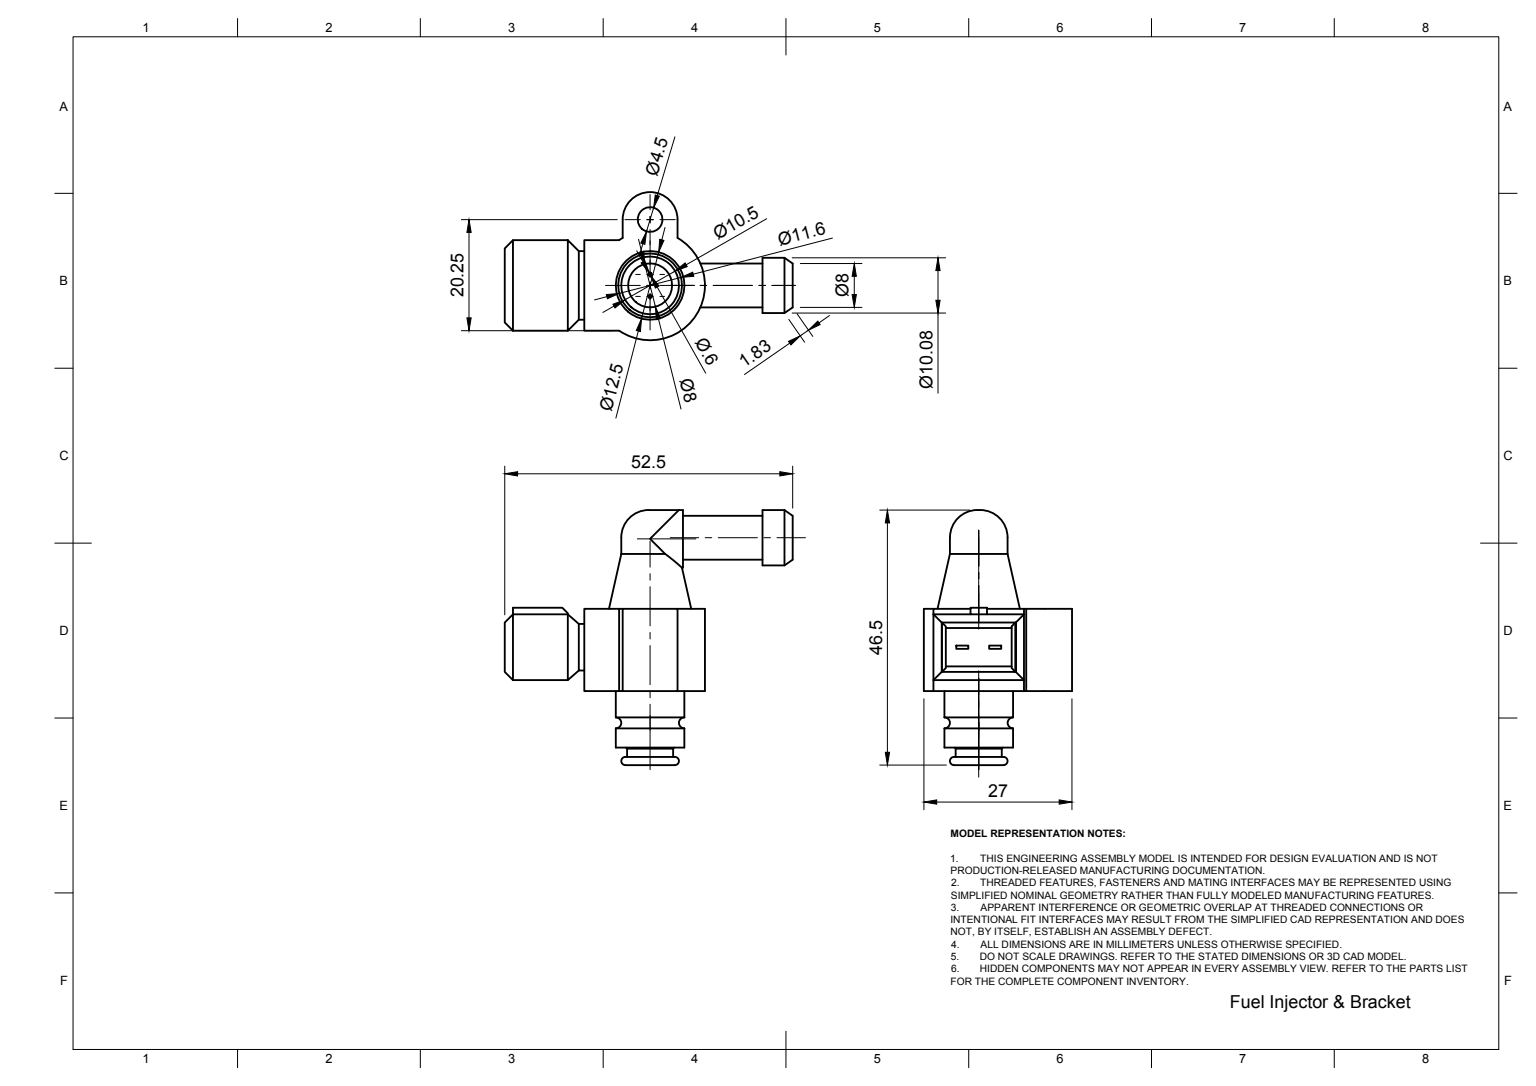
ISO-10303-21;
HEADER;
/* Generated by software containing ST-Developer
 * from STEP Tools, Inc. (www.steptools.com) 
 */

FILE_DESCRIPTION(
/* description */ ('STEP AP214'),
/* implementation_level */ '2;1');

FILE_NAME(
/* name */ 'Fuel Injector & Bracket.step',
/* time_stamp */ '2026-10-07T12:18:07-07:00',
/* author */ (''),
/* organization */ (''),
/* preprocessor_version */ 'ST-DEVELOPER v20.2',
/* originating_system */ 'Autodesk Translation Framework v15.15.0.0',
/* authorisation */ '');

FILE_SCHEMA (('AUTOMOTIVE_DESIGN { 1 0 10303 214 3 1 1 }'));
ENDSEC;

DATA;
#10=MECHANICAL_DESIGN_GEOMETRIC_PRESENTATION_REPRESENTATION('',(#122),#62974);
#98=SHAPE_REPRESENTATION_RELATIONSHIP('SRR','None',#63021,#110);
#110=ADVANCED_BREP_SHAPE_REPRESENTATION('',(#134),#62962);
#122=STYLED_ITEM('',(#63090),#134);
#134=MANIFOLD_SOLID_BREP('Body1',#15192);
#146=(
BOUNDED_SURFACE()
B_SPLINE_SURFACE(2,2,((#27768,#27769,#27770,#27771,#27772,#27773,#27774),
(#27775,#27776,#27777,#27778,#27779,#27780,#27781),(#27782,#27783,#27784,
#27785,#27786,#27787,#27788)),.UNSPECIFIED.,.F.,.F.,.F.)
B_SPLINE_SURFACE_WITH_KNOTS((3,3),(3,2,2,3),(-1.57079632681342,3.50763862399952E-12),
(-1.6184333897888,-0.539477796596266,0.539477796596266,1.6184333897888),
 .UNSPECIFIED.)
GEOMETRIC_REPRESENTATION_ITEM()
RATIONAL_B_SPLINE_SURFACE(((1.,0.857977047969415,1.,0.857977047969415,1.,
0.857977047969415,1.),(0.707106781178761,0.606681388714908,0.707106781178761,
0.606681388714908,0.707106781178761,0.606681388714908,0.707106781178761),
(1.,0.857977047969415,1.,0.857977047969415,1.,0.857977047969415,1.)))
REPRESENTATION_ITEM('')
SURFACE()
);
#192=B_SPLINE_SURFACE_WITH_KNOTS('',3,3,((#21716,#21717,#21718,#21719,#21720,
#21721,#21722,#21723,#21724,#21725,#21726,#21727,#21728,#21729,#21730,#21731,
#21732,#21733,#21734,#21735,#21736,#21737,#21738,#21739,#21740,#21741,#21742,
#21743,#21744,#21745,#21746,#21747,#21748,#21749,#21750,#21751,#21752,#21753,
#21754,#21755,#21756,#21757,#21758,#21759,#21760,#21761,#21762,#21763,#21764),
(#21765,#21766,#21767,#21768,#21769,#21770,#21771,#21772,#21773,#21774,
#21775,#21776,#21777,#21778,#21779,#21780,#21781,#21782,#21783,#21784,#21785,
#21786,#21787,#21788,#21789,#21790,#21791,#21792,#21793,#21794,#21795,#21796,
#21797,#21798,#21799,#21800,#21801,#21802,#21803,#21804,#21805,#21806,#21807,
#21808,#21809,#21810,#21811,#21812,#21813),(#21814,#21815,#21816,#21817,
#21818,#21819,#21820,#21821,#21822,#21823,#21824,#21825,#21826,#21827,#21828,
#21829,#21830,#21831,#21832,#21833,#21834,#21835,#21836,#21837,#21838,#21839,
#21840,#21841,#21842,#21843,#21844,#21845,#21846,#21847,#21848,#21849,#21850,
#21851,#21852,#21853,#21854,#21855,#21856,#21857,#21858,#21859,#21860,#21861,
#21862),(#21863,#21864,#21865,#21866,#21867,#21868,#21869,#21870,#21871,
#21872,#21873,#21874,#21875,#21876,#21877,#21878,#21879,#21880,#21881,#21882,
#21883,#21884,#21885,#21886,#21887,#21888,#21889,#21890,#21891,#21892,#21893,
#21894,#21895,#21896,#21897,#21898,#21899,#21900,#21901,#21902,#21903,#21904,
#21905,#21906,#21907,#21908,#21909,#21910,#21911),(#21912,#21913,#21914,
#21915,#21916,#21917,#21918,#21919,#21920,#21921,#21922,#21923,#21924,#21925,
#21926,#21927,#21928,#21929,#21930,#21931,#21932,#21933,#21934,#21935,#21936,
#21937,#21938,#21939,#21940,#21941,#21942,#21943,#21944,#21945,#21946,#21947,
#21948,#21949,#21950,#21951,#21952,#21953,#21954,#21955,#21956,#21957,#21958,
#21959,#21960),(#21961,#21962,#21963,#21964,#21965,#21966,#21967,#21968,
#21969,#21970,#21971,#21972,#21973,#21974,#21975,#21976,#21977,#21978,#21979,
#21980,#21981,#21982,#21983,#21984,#21985,#21986,#21987,#21988,#21989,#21990,
#21991,#21992,#21993,#21994,#21995,#21996,#21997,#21998,#21999,#22000,#22001,
#22002,#22003,#22004,#22005,#22006,#22007,#22008,#22009),(#22010,#22011,
#22012,#22013,#22014,#22015,#22016,#22017,#22018,#22019,#22020,#22021,#22022,
#22023,#22024,#22025,#22026,#22027,#22028,#22029,#22030,#22031,#22032,#22033,
#22034,#22035,#22036,#22037,#22038,#22039,#22040,#22041,#22042,#22043,#22044,
#22045,#22046,#22047,#22048,#22049,#22050,#22051,#22052,#22053,#22054,#22055,
#22056,#22057,#22058),(#22059,#22060,#22061,#22062,#22063,#22064,#22065,
#22066,#22067,#22068,#22069,#22070,#22071,#22072,#22073,#22074,#22075,#22076,
#22077,#22078,#22079,#22080,#22081,#22082,#22083,#22084,#22085,#22086,#22087,
#22088,#22089,#22090,#22091,#22092,#22093,#22094,#22095,#22096,#22097,#22098,
#22099,#22100,#22101,#22102,#22103,#22104,#22105,#22106,#22107),(#22108,
#22109,#22110,#22111,#22112,#22113,#22114,#22115,#22116,#22117,#22118,#22119,
#22120,#22121,#22122,#22123,#22124,#22125,#22126,#22127,#22128,#22129,#22130,
#22131,#22132,#22133,#22134,#22135,#22136,#22137,#22138,#22139,#22140,#22141,
#22142,#22143,#22144,#22145,#22146,#22147,#22148,#22149,#22150,#22151,#22152,
#22153,#22154,#22155,#22156),(#22157,#22158,#22159,#22160,#22161,#22162,
#22163,#22164,#22165,#22166,#22167,#22168,#22169,#22170,#22171,#22172,#22173,
#22174,#22175,#22176,#22177,#22178,#22179,#22180,#22181,#22182,#22183,#22184,
#22185,#22186,#22187,#22188,#22189,#22190,#22191,#22192,#22193,#22194,#22195,
#22196,#22197,#22198,#22199,#22200,#22201,#22202,#22203,#22204,#22205),
(#22206,#22207,#22208,#22209,#22210,#22211,#22212,#22213,#22214,#22215,
#22216,#22217,#22218,#22219,#22220,#22221,#22222,#22223,#22224,#22225,#22226,
#22227,#22228,#22229,#22230,#22231,#22232,#22233,#22234,#22235,#22236,#22237,
#22238,#22239,#22240,#22241,#22242,#22243,#22244,#22245,#22246,#22247,#22248,
#22249,#22250,#22251,#22252,#22253,#22254),(#22255,#22256,#22257,#22258,
#22259,#22260,#22261,#22262,#22263,#22264,#22265,#22266,#22267,#22268,#22269,
#22270,#22271,#22272,#22273,#22274,#22275,#22276,#22277,#22278,#22279,#22280,
#22281,#22282,#22283,#22284,#22285,#22286,#22287,#22288,#22289,#22290,#22291,
#22292,#22293,#22294,#22295,#22296,#22297,#22298,#22299,#22300,#22301,#22302,
#22303),(#22304,#22305,#22306,#22307,#22308,#22309,#22310,#22311,#22312,
#22313,#22314,#22315,#22316,#22317,#22318,#22319,#22320,#22321,#22322,#22323,
#22324,#22325,#22326,#22327,#22328,#22329,#22330,#22331,#22332,#22333,#22334,
#22335,#22336,#22337,#22338,#22339,#22340,#22341,#22342,#22343,#22344,#22345,
#22346,#22347,#22348,#22349,#22350,#22351,#22352),(#22353,#22354,#22355,
#22356,#22357,#22358,#22359,#22360,#22361,#22362,#22363,#22364,#22365,#22366,
#22367,#22368,#22369,#22370,#22371,#22372,#22373,#22374,#22375,#22376,#22377,
#22378,#22379,#22380,#22381,#22382,#22383,#22384,#22385,#22386,#22387,#22388,
#22389,#22390,#22391,#22392,#22393,#22394,#22395,#22396,#22397,#22398,#22399,
#22400,#22401),(#22402,#22403,#22404,#22405,#22406,#22407,#22408,#22409,
#22410,#22411,#22412,#22413,#22414,#22415,#22416,#22417,#22418,#22419,#22420,
#22421,#22422,#22423,#22424,#22425,#22426,#22427,#22428,#22429,#22430,#22431,
#22432,#22433,#22434,#22435,#22436,#22437,#22438,#22439,#22440,#22441,#22442,
#22443,#22444,#22445,#22446,#22447,#22448,#22449,#22450),(#22451,#22452,
#22453,#22454,#22455,#22456,#22457,#22458,#22459,#22460,#22461,#22462,#22463,
#22464,#22465,#22466,#22467,#22468,#22469,#22470,#22471,#22472,#22473,#22474,
#22475,#22476,#22477,#22478,#22479,#22480,#22481,#22482,#22483,#22484,#22485,
#22486,#22487,#22488,#22489,#22490,#22491,#22492,#22493,#22494,#22495,#22496,
#22497,#22498,#22499),(#22500,#22501,#22502,#22503,#22504,#22505,#22506,
#22507,#22508,#22509,#22510,#22511,#22512,#22513,#22514,#22515,#22516,#22517,
#22518,#22519,#22520,#22521,#22522,#22523,#22524,#22525,#22526,#22527,#22528,
#22529,#22530,#22531,#22532,#22533,#22534,#22535,#22536,#22537,#22538,#22539,
#22540,#22541,#22542,#22543,#22544,#22545,#22546,#22547,#22548),(#22549,
#22550,#22551,#22552,#22553,#22554,#22555,#22556,#22557,#22558,#22559,#22560,
#22561,#22562,#22563,#22564,#22565,#22566,#22567,#22568,#22569,#22570,#22571,
#22572,#22573,#22574,#22575,#22576,#22577,#22578,#22579,#22580,#22581,#22582,
#22583,#22584,#22585,#22586,#22587,#22588,#22589,#22590,#22591,#22592,#22593,
#22594,#22595,#22596,#22597),(#22598,#22599,#22600,#22601,#22602,#22603,
#22604,#22605,#22606,#22607,#22608,#22609,#22610,#22611,#22612,#22613,#22614,
#22615,#22616,#22617,#22618,#22619,#22620,#22621,#22622,#22623,#22624,#22625,
#22626,#22627,#22628,#22629,#22630,#22631,#22632,#22633,#22634,#22635,#22636,
#22637,#22638,#22639,#22640,#22641,#22642,#22643,#22644,#22645,#22646),
(#22647,#22648,#22649,#22650,#22651,#22652,#22653,#22654,#22655,#22656,
#22657,#22658,#22659,#22660,#22661,#22662,#22663,#22664,#22665,#22666,#22667,
#22668,#22669,#22670,#22671,#22672,#22673,#22674,#22675,#22676,#22677,#22678,
#22679,#22680,#22681,#22682,#22683,#22684,#22685,#22686,#22687,#22688,#22689,
#22690,#22691,#22692,#22693,#22694,#22695),(#22696,#22697,#22698,#22699,
#22700,#22701,#22702,#22703,#22704,#22705,#22706,#22707,#22708,#22709,#22710,
#22711,#22712,#22713,#22714,#22715,#22716,#22717,#22718,#22719,#22720,#22721,
#22722,#22723,#22724,#22725,#22726,#22727,#22728,#22729,#22730,#22731,#22732,
#22733,#22734,#22735,#22736,#22737,#22738,#22739,#22740,#22741,#22742,#22743,
#22744),(#22745,#22746,#22747,#22748,#22749,#22750,#22751,#22752,#22753,
#22754,#22755,#22756,#22757,#22758,#22759,#22760,#22761,#22762,#22763,#22764,
#22765,#22766,#22767,#22768,#22769,#22770,#22771,#22772,#22773,#22774,#22775,
#22776,#22777,#22778,#22779,#22780,#22781,#22782,#22783,#22784,#22785,#22786,
#22787,#22788,#22789,#22790,#22791,#22792,#22793),(#22794,#22795,#22796,
#22797,#22798,#22799,#22800,#22801,#22802,#22803,#22804,#22805,#22806,#22807,
#22808,#22809,#22810,#22811,#22812,#22813,#22814,#22815,#22816,#22817,#22818,
#22819,#22820,#22821,#22822,#22823,#22824,#22825,#22826,#22827,#22828,#22829,
#22830,#22831,#22832,#22833,#22834,#22835,#22836,#22837,#22838,#22839,#22840,
#22841,#22842),(#22843,#22844,#22845,#22846,#22847,#22848,#22849,#22850,
#22851,#22852,#22853,#22854,#22855,#22856,#22857,#22858,#22859,#22860,#22861,
#22862,#22863,#22864,#22865,#22866,#22867,#22868,#22869,#22870,#22871,#22872,
#22873,#22874,#22875,#22876,#22877,#22878,#22879,#22880,#22881,#22882,#22883,
#22884,#22885,#22886,#22887,#22888,#22889,#22890,#22891),(#22892,#22893,
#22894,#22895,#22896,#22897,#22898,#22899,#22900,#22901,#22902,#22903,#22904,
#22905,#22906,#22907,#22908,#22909,#22910,#22911,#22912,#22913,#22914,#22915,
#22916,#22917,#22918,#22919,#22920,#22921,#22922,#22923,#22924,#22925,#22926,
#22927,#22928,#22929,#22930,#22931,#22932,#22933,#22934,#22935,#22936,#22937,
#22938,#22939,#22940),(#22941,#22942,#22943,#22944,#22945,#22946,#22947,
#22948,#22949,#22950,#22951,#22952,#22953,#22954,#22955,#22956,#22957,#22958,
#22959,#22960,#22961,#22962,#22963,#22964,#22965,#22966,#22967,#22968,#22969,
#22970,#22971,#22972,#22973,#22974,#22975,#22976,#22977,#22978,#22979,#22980,
#22981,#22982,#22983,#22984,#22985,#22986,#22987,#22988,#22989),(#22990,
#22991,#22992,#22993,#22994,#22995,#22996,#22997,#22998,#22999,#23000,#23001,
#23002,#23003,#23004,#23005,#23006,#23007,#23008,#23009,#23010,#23011,#23012,
#23013,#23014,#23015,#23016,#23017,#23018,#23019,#23020,#23021,#23022,#23023,
#23024,#23025,#23026,#23027,#23028,#23029,#23030,#23031,#23032,#23033,#23034,
#23035,#23036,#23037,#23038),(#23039,#23040,#23041,#23042,#23043,#23044,
#23045,#23046,#23047,#23048,#23049,#23050,#23051,#23052,#23053,#23054,#23055,
#23056,#23057,#23058,#23059,#23060,#23061,#23062,#23063,#23064,#23065,#23066,
#23067,#23068,#23069,#23070,#23071,#23072,#23073,#23074,#23075,#23076,#23077,
#23078,#23079,#23080,#23081,#23082,#23083,#23084,#23085,#23086,#23087),
(#23088,#23089,#23090,#23091,#23092,#23093,#23094,#23095,#23096,#23097,
#23098,#23099,#23100,#23101,#23102,#23103,#23104,#23105,#23106,#23107,#23108,
#23109,#23110,#23111,#23112,#23113,#23114,#23115,#23116,#23117,#23118,#23119,
#23120,#23121,#23122,#23123,#23124,#23125,#23126,#23127,#23128,#23129,#23130,
#23131,#23132,#23133,#23134,#23135,#23136),(#23137,#23138,#23139,#23140,
#23141,#23142,#23143,#23144,#23145,#23146,#23147,#23148,#23149,#23150,#23151,
#23152,#23153,#23154,#23155,#23156,#23157,#23158,#23159,#23160,#23161,#23162,
#23163,#23164,#23165,#23166,#23167,#23168,#23169,#23170,#23171,#23172,#23173,
#23174,#23175,#23176,#23177,#23178,#23179,#23180,#23181,#23182,#23183,#23184,
#23185),(#23186,#23187,#23188,#23189,#23190,#23191,#23192,#23193,#23194,
#23195,#23196,#23197,#23198,#23199,#23200,#23201,#23202,#23203,#23204,#23205,
#23206,#23207,#23208,#23209,#23210,#23211,#23212,#23213,#23214,#23215,#23216,
#23217,#23218,#23219,#23220,#23221,#23222,#23223,#23224,#23225,#23226,#23227,
#23228,#23229,#23230,#23231,#23232,#23233,#23234),(#23235,#23236,#23237,
#23238,#23239,#23240,#23241,#23242,#23243,#23244,#23245,#23246,#23247,#23248,
#23249,#23250,#23251,#23252,#23253,#23254,#23255,#23256,#23257,#23258,#23259,
#23260,#23261,#23262,#23263,#23264,#23265,#23266,#23267,#23268,#23269,#23270,
#23271,#23272,#23273,#23274,#23275,#23276,#23277,#23278,#23279,#23280,#23281,
#23282,#23283),(#23284,#23285,#23286,#23287,#23288,#23289,#23290,#23291,
#23292,#23293,#23294,#23295,#23296,#23297,#23298,#23299,#23300,#23301,#23302,
#23303,#23304,#23305,#23306,#23307,#23308,#23309,#23310,#23311,#23312,#23313,
#23314,#23315,#23316,#23317,#23318,#23319,#23320,#23321,#23322,#23323,#23324,
#23325,#23326,#23327,#23328,#23329,#23330,#23331,#23332),(#23333,#23334,
#23335,#23336,#23337,#23338,#23339,#23340,#23341,#23342,#23343,#23344,#23345,
#23346,#23347,#23348,#23349,#23350,#23351,#23352,#23353,#23354,#23355,#23356,
#23357,#23358,#23359,#23360,#23361,#23362,#23363,#23364,#23365,#23366,#23367,
#23368,#23369,#23370,#23371,#23372,#23373,#23374,#23375,#23376,#23377,#23378,
#23379,#23380,#23381),(#23382,#23383,#23384,#23385,#23386,#23387,#23388,
#23389,#23390,#23391,#23392,#23393,#23394,#23395,#23396,#23397,#23398,#23399,
#23400,#23401,#23402,#23403,#23404,#23405,#23406,#23407,#23408,#23409,#23410,
#23411,#23412,#23413,#23414,#23415,#23416,#23417,#23418,#23419,#23420,#23421,
#23422,#23423,#23424,#23425,#23426,#23427,#23428,#23429,#23430),(#23431,
#23432,#23433,#23434,#23435,#23436,#23437,#23438,#23439,#23440,#23441,#23442,
#23443,#23444,#23445,#23446,#23447,#23448,#23449,#23450,#23451,#23452,#23453,
#23454,#23455,#23456,#23457,#23458,#23459,#23460,#23461,#23462,#23463,#23464,
#23465,#23466,#23467,#23468,#23469,#23470,#23471,#23472,#23473,#23474,#23475,
#23476,#23477,#23478,#23479),(#23480,#23481,#23482,#23483,#23484,#23485,
#23486,#23487,#23488,#23489,#23490,#23491,#23492,#23493,#23494,#23495,#23496,
#23497,#23498,#23499,#23500,#23501,#23502,#23503,#23504,#23505,#23506,#23507,
#23508,#23509,#23510,#23511,#23512,#23513,#23514,#23515,#23516,#23517,#23518,
#23519,#23520,#23521,#23522,#23523,#23524,#23525,#23526,#23527,#23528),
(#23529,#23530,#23531,#23532,#23533,#23534,#23535,#23536,#23537,#23538,
#23539,#23540,#23541,#23542,#23543,#23544,#23545,#23546,#23547,#23548,#23549,
#23550,#23551,#23552,#23553,#23554,#23555,#23556,#23557,#23558,#23559,#23560,
#23561,#23562,#23563,#23564,#23565,#23566,#23567,#23568,#23569,#23570,#23571,
#23572,#23573,#23574,#23575,#23576,#23577),(#23578,#23579,#23580,#23581,
#23582,#23583,#23584,#23585,#23586,#23587,#23588,#23589,#23590,#23591,#23592,
#23593,#23594,#23595,#23596,#23597,#23598,#23599,#23600,#23601,#23602,#23603,
#23604,#23605,#23606,#23607,#23608,#23609,#23610,#23611,#23612,#23613,#23614,
#23615,#23616,#23617,#23618,#23619,#23620,#23621,#23622,#23623,#23624,#23625,
#23626),(#23627,#23628,#23629,#23630,#23631,#23632,#23633,#23634,#23635,
#23636,#23637,#23638,#23639,#23640,#23641,#23642,#23643,#23644,#23645,#23646,
#23647,#23648,#23649,#23650,#23651,#23652,#23653,#23654,#23655,#23656,#23657,
#23658,#23659,#23660,#23661,#23662,#23663,#23664,#23665,#23666,#23667,#23668,
#23669,#23670,#23671,#23672,#23673,#23674,#23675),(#23676,#23677,#23678,
#23679,#23680,#23681,#23682,#23683,#23684,#23685,#23686,#23687,#23688,#23689,
#23690,#23691,#23692,#23693,#23694,#23695,#23696,#23697,#23698,#23699,#23700,
#23701,#23702,#23703,#23704,#23705,#23706,#23707,#23708,#23709,#23710,#23711,
#23712,#23713,#23714,#23715,#23716,#23717,#23718,#23719,#23720,#23721,#23722,
#23723,#23724),(#23725,#23726,#23727,#23728,#23729,#23730,#23731,#23732,
#23733,#23734,#23735,#23736,#23737,#23738,#23739,#23740,#23741,#23742,#23743,
#23744,#23745,#23746,#23747,#23748,#23749,#23750,#23751,#23752,#23753,#23754,
#23755,#23756,#23757,#23758,#23759,#23760,#23761,#23762,#23763,#23764,#23765,
#23766,#23767,#23768,#23769,#23770,#23771,#23772,#23773),(#23774,#23775,
#23776,#23777,#23778,#23779,#23780,#23781,#23782,#23783,#23784,#23785,#23786,
#23787,#23788,#23789,#23790,#23791,#23792,#23793,#23794,#23795,#23796,#23797,
#23798,#23799,#23800,#23801,#23802,#23803,#23804,#23805,#23806,#23807,#23808,
#23809,#23810,#23811,#23812,#23813,#23814,#23815,#23816,#23817,#23818,#23819,
#23820,#23821,#23822),(#23823,#23824,#23825,#23826,#23827,#23828,#23829,
#23830,#23831,#23832,#23833,#23834,#23835,#23836,#23837,#23838,#23839,#23840,
#23841,#23842,#23843,#23844,#23845,#23846,#23847,#23848,#23849,#23850,#23851,
#23852,#23853,#23854,#23855,#23856,#23857,#23858,#23859,#23860,#23861,#23862,
#23863,#23864,#23865,#23866,#23867,#23868,#23869,#23870,#23871),(#23872,
#23873,#23874,#23875,#23876,#23877,#23878,#23879,#23880,#23881,#23882,#23883,
#23884,#23885,#23886,#23887,#23888,#23889,#23890,#23891,#23892,#23893,#23894,
#23895,#23896,#23897,#23898,#23899,#23900,#23901,#23902,#23903,#23904,#23905,
#23906,#23907,#23908,#23909,#23910,#23911,#23912,#23913,#23914,#23915,#23916,
#23917,#23918,#23919,#23920),(#23921,#23922,#23923,#23924,#23925,#23926,
#23927,#23928,#23929,#23930,#23931,#23932,#23933,#23934,#23935,#23936,#23937,
#23938,#23939,#23940,#23941,#23942,#23943,#23944,#23945,#23946,#23947,#23948,
#23949,#23950,#23951,#23952,#23953,#23954,#23955,#23956,#23957,#23958,#23959,
#23960,#23961,#23962,#23963,#23964,#23965,#23966,#23967,#23968,#23969),
(#23970,#23971,#23972,#23973,#23974,#23975,#23976,#23977,#23978,#23979,
#23980,#23981,#23982,#23983,#23984,#23985,#23986,#23987,#23988,#23989,#23990,
#23991,#23992,#23993,#23994,#23995,#23996,#23997,#23998,#23999,#24000,#24001,
#24002,#24003,#24004,#24005,#24006,#24007,#24008,#24009,#24010,#24011,#24012,
#24013,#24014,#24015,#24016,#24017,#24018),(#24019,#24020,#24021,#24022,
#24023,#24024,#24025,#24026,#24027,#24028,#24029,#24030,#24031,#24032,#24033,
#24034,#24035,#24036,#24037,#24038,#24039,#24040,#24041,#24042,#24043,#24044,
#24045,#24046,#24047,#24048,#24049,#24050,#24051,#24052,#24053,#24054,#24055,
#24056,#24057,#24058,#24059,#24060,#24061,#24062,#24063,#24064,#24065,#24066,
#24067),(#24068,#24069,#24070,#24071,#24072,#24073,#24074,#24075,#24076,
#24077,#24078,#24079,#24080,#24081,#24082,#24083,#24084,#24085,#24086,#24087,
#24088,#24089,#24090,#24091,#24092,#24093,#24094,#24095,#24096,#24097,#24098,
#24099,#24100,#24101,#24102,#24103,#24104,#24105,#24106,#24107,#24108,#24109,
#24110,#24111,#24112,#24113,#24114,#24115,#24116),(#24117,#24118,#24119,
#24120,#24121,#24122,#24123,#24124,#24125,#24126,#24127,#24128,#24129,#24130,
#24131,#24132,#24133,#24134,#24135,#24136,#24137,#24138,#24139,#24140,#24141,
#24142,#24143,#24144,#24145,#24146,#24147,#24148,#24149,#24150,#24151,#24152,
#24153,#24154,#24155,#24156,#24157,#24158,#24159,#24160,#24161,#24162,#24163,
#24164,#24165),(#24166,#24167,#24168,#24169,#24170,#24171,#24172,#24173,
#24174,#24175,#24176,#24177,#24178,#24179,#24180,#24181,#24182,#24183,#24184,
#24185,#24186,#24187,#24188,#24189,#24190,#24191,#24192,#24193,#24194,#24195,
#24196,#24197,#24198,#24199,#24200,#24201,#24202,#24203,#24204,#24205,#24206,
#24207,#24208,#24209,#24210,#24211,#24212,#24213,#24214),(#24215,#24216,
#24217,#24218,#24219,#24220,#24221,#24222,#24223,#24224,#24225,#24226,#24227,
#24228,#24229,#24230,#24231,#24232,#24233,#24234,#24235,#24236,#24237,#24238,
#24239,#24240,#24241,#24242,#24243,#24244,#24245,#24246,#24247,#24248,#24249,
#24250,#24251,#24252,#24253,#24254,#24255,#24256,#24257,#24258,#24259,#24260,
#24261,#24262,#24263),(#24264,#24265,#24266,#24267,#24268,#24269,#24270,
#24271,#24272,#24273,#24274,#24275,#24276,#24277,#24278,#24279,#24280,#24281,
#24282,#24283,#24284,#24285,#24286,#24287,#24288,#24289,#24290,#24291,#24292,
#24293,#24294,#24295,#24296,#24297,#24298,#24299,#24300,#24301,#24302,#24303,
#24304,#24305,#24306,#24307,#24308,#24309,#24310,#24311,#24312),(#24313,
#24314,#24315,#24316,#24317,#24318,#24319,#24320,#24321,#24322,#24323,#24324,
#24325,#24326,#24327,#24328,#24329,#24330,#24331,#24332,#24333,#24334,#24335,
#24336,#24337,#24338,#24339,#24340,#24341,#24342,#24343,#24344,#24345,#24346,
#24347,#24348,#24349,#24350,#24351,#24352,#24353,#24354,#24355,#24356,#24357,
#24358,#24359,#24360,#24361),(#24362,#24363,#24364,#24365,#24366,#24367,
#24368,#24369,#24370,#24371,#24372,#24373,#24374,#24375,#24376,#24377,#24378,
#24379,#24380,#24381,#24382,#24383,#24384,#24385,#24386,#24387,#24388,#24389,
#24390,#24391,#24392,#24393,#24394,#24395,#24396,#24397,#24398,#24399,#24400,
#24401,#24402,#24403,#24404,#24405,#24406,#24407,#24408,#24409,#24410),
(#24411,#24412,#24413,#24414,#24415,#24416,#24417,#24418,#24419,#24420,
#24421,#24422,#24423,#24424,#24425,#24426,#24427,#24428,#24429,#24430,#24431,
#24432,#24433,#24434,#24435,#24436,#24437,#24438,#24439,#24440,#24441,#24442,
#24443,#24444,#24445,#24446,#24447,#24448,#24449,#24450,#24451,#24452,#24453,
#24454,#24455,#24456,#24457,#24458,#24459),(#24460,#24461,#24462,#24463,
#24464,#24465,#24466,#24467,#24468,#24469,#24470,#24471,#24472,#24473,#24474,
#24475,#24476,#24477,#24478,#24479,#24480,#24481,#24482,#24483,#24484,#24485,
#24486,#24487,#24488,#24489,#24490,#24491,#24492,#24493,#24494,#24495,#24496,
#24497,#24498,#24499,#24500,#24501,#24502,#24503,#24504,#24505,#24506,#24507,
#24508),(#24509,#24510,#24511,#24512,#24513,#24514,#24515,#24516,#24517,
#24518,#24519,#24520,#24521,#24522,#24523,#24524,#24525,#24526,#24527,#24528,
#24529,#24530,#24531,#24532,#24533,#24534,#24535,#24536,#24537,#24538,#24539,
#24540,#24541,#24542,#24543,#24544,#24545,#24546,#24547,#24548,#24549,#24550,
#24551,#24552,#24553,#24554,#24555,#24556,#24557),(#24558,#24559,#24560,
#24561,#24562,#24563,#24564,#24565,#24566,#24567,#24568,#24569,#24570,#24571,
#24572,#24573,#24574,#24575,#24576,#24577,#24578,#24579,#24580,#24581,#24582,
#24583,#24584,#24585,#24586,#24587,#24588,#24589,#24590,#24591,#24592,#24593,
#24594,#24595,#24596,#24597,#24598,#24599,#24600,#24601,#24602,#24603,#24604,
#24605,#24606),(#24607,#24608,#24609,#24610,#24611,#24612,#24613,#24614,
#24615,#24616,#24617,#24618,#24619,#24620,#24621,#24622,#24623,#24624,#24625,
#24626,#24627,#24628,#24629,#24630,#24631,#24632,#24633,#24634,#24635,#24636,
#24637,#24638,#24639,#24640,#24641,#24642,#24643,#24644,#24645,#24646,#24647,
#24648,#24649,#24650,#24651,#24652,#24653,#24654,#24655),(#24656,#24657,
#24658,#24659,#24660,#24661,#24662,#24663,#24664,#24665,#24666,#24667,#24668,
#24669,#24670,#24671,#24672,#24673,#24674,#24675,#24676,#24677,#24678,#24679,
#24680,#24681,#24682,#24683,#24684,#24685,#24686,#24687,#24688,#24689,#24690,
#24691,#24692,#24693,#24694,#24695,#24696,#24697,#24698,#24699,#24700,#24701,
#24702,#24703,#24704),(#24705,#24706,#24707,#24708,#24709,#24710,#24711,
#24712,#24713,#24714,#24715,#24716,#24717,#24718,#24719,#24720,#24721,#24722,
#24723,#24724,#24725,#24726,#24727,#24728,#24729,#24730,#24731,#24732,#24733,
#24734,#24735,#24736,#24737,#24738,#24739,#24740,#24741,#24742,#24743,#24744,
#24745,#24746,#24747,#24748,#24749,#24750,#24751,#24752,#24753),(#24754,
#24755,#24756,#24757,#24758,#24759,#24760,#24761,#24762,#24763,#24764,#24765,
#24766,#24767,#24768,#24769,#24770,#24771,#24772,#24773,#24774,#24775,#24776,
#24777,#24778,#24779,#24780,#24781,#24782,#24783,#24784,#24785,#24786,#24787,
#24788,#24789,#24790,#24791,#24792,#24793,#24794,#24795,#24796,#24797,#24798,
#24799,#24800,#24801,#24802),(#24803,#24804,#24805,#24806,#24807,#24808,
#24809,#24810,#24811,#24812,#24813,#24814,#24815,#24816,#24817,#24818,#24819,
#24820,#24821,#24822,#24823,#24824,#24825,#24826,#24827,#24828,#24829,#24830,
#24831,#24832,#24833,#24834,#24835,#24836,#24837,#24838,#24839,#24840,#24841,
#24842,#24843,#24844,#24845,#24846,#24847,#24848,#24849,#24850,#24851),
(#24852,#24853,#24854,#24855,#24856,#24857,#24858,#24859,#24860,#24861,
#24862,#24863,#24864,#24865,#24866,#24867,#24868,#24869,#24870,#24871,#24872,
#24873,#24874,#24875,#24876,#24877,#24878,#24879,#24880,#24881,#24882,#24883,
#24884,#24885,#24886,#24887,#24888,#24889,#24890,#24891,#24892,#24893,#24894,
#24895,#24896,#24897,#24898,#24899,#24900),(#24901,#24902,#24903,#24904,
#24905,#24906,#24907,#24908,#24909,#24910,#24911,#24912,#24913,#24914,#24915,
#24916,#24917,#24918,#24919,#24920,#24921,#24922,#24923,#24924,#24925,#24926,
#24927,#24928,#24929,#24930,#24931,#24932,#24933,#24934,#24935,#24936,#24937,
#24938,#24939,#24940,#24941,#24942,#24943,#24944,#24945,#24946,#24947,#24948,
#24949),(#24950,#24951,#24952,#24953,#24954,#24955,#24956,#24957,#24958,
#24959,#24960,#24961,#24962,#24963,#24964,#24965,#24966,#24967,#24968,#24969,
#24970,#24971,#24972,#24973,#24974,#24975,#24976,#24977,#24978,#24979,#24980,
#24981,#24982,#24983,#24984,#24985,#24986,#24987,#24988,#24989,#24990,#24991,
#24992,#24993,#24994,#24995,#24996,#24997,#24998),(#24999,#25000,#25001,
#25002,#25003,#25004,#25005,#25006,#25007,#25008,#25009,#25010,#25011,#25012,
#25013,#25014,#25015,#25016,#25017,#25018,#25019,#25020,#25021,#25022,#25023,
#25024,#25025,#25026,#25027,#25028,#25029,#25030,#25031,#25032,#25033,#25034,
#25035,#25036,#25037,#25038,#25039,#25040,#25041,#25042,#25043,#25044,#25045,
#25046,#25047),(#25048,#25049,#25050,#25051,#25052,#25053,#25054,#25055,
#25056,#25057,#25058,#25059,#25060,#25061,#25062,#25063,#25064,#25065,#25066,
#25067,#25068,#25069,#25070,#25071,#25072,#25073,#25074,#25075,#25076,#25077,
#25078,#25079,#25080,#25081,#25082,#25083,#25084,#25085,#25086,#25087,#25088,
#25089,#25090,#25091,#25092,#25093,#25094,#25095,#25096),(#25097,#25098,
#25099,#25100,#25101,#25102,#25103,#25104,#25105,#25106,#25107,#25108,#25109,
#25110,#25111,#25112,#25113,#25114,#25115,#25116,#25117,#25118,#25119,#25120,
#25121,#25122,#25123,#25124,#25125,#25126,#25127,#25128,#25129,#25130,#25131,
#25132,#25133,#25134,#25135,#25136,#25137,#25138,#25139,#25140,#25141,#25142,
#25143,#25144,#25145),(#25146,#25147,#25148,#25149,#25150,#25151,#25152,
#25153,#25154,#25155,#25156,#25157,#25158,#25159,#25160,#25161,#25162,#25163,
#25164,#25165,#25166,#25167,#25168,#25169,#25170,#25171,#25172,#25173,#25174,
#25175,#25176,#25177,#25178,#25179,#25180,#25181,#25182,#25183,#25184,#25185,
#25186,#25187,#25188,#25189,#25190,#25191,#25192,#25193,#25194),(#25195,
#25196,#25197,#25198,#25199,#25200,#25201,#25202,#25203,#25204,#25205,#25206,
#25207,#25208,#25209,#25210,#25211,#25212,#25213,#25214,#25215,#25216,#25217,
#25218,#25219,#25220,#25221,#25222,#25223,#25224,#25225,#25226,#25227,#25228,
#25229,#25230,#25231,#25232,#25233,#25234,#25235,#25236,#25237,#25238,#25239,
#25240,#25241,#25242,#25243),(#25244,#25245,#25246,#25247,#25248,#25249,
#25250,#25251,#25252,#25253,#25254,#25255,#25256,#25257,#25258,#25259,#25260,
#25261,#25262,#25263,#25264,#25265,#25266,#25267,#25268,#25269,#25270,#25271,
#25272,#25273,#25274,#25275,#25276,#25277,#25278,#25279,#25280,#25281,#25282,
#25283,#25284,#25285,#25286,#25287,#25288,#25289,#25290,#25291,#25292),
(#25293,#25294,#25295,#25296,#25297,#25298,#25299,#25300,#25301,#25302,
#25303,#25304,#25305,#25306,#25307,#25308,#25309,#25310,#25311,#25312,#25313,
#25314,#25315,#25316,#25317,#25318,#25319,#25320,#25321,#25322,#25323,#25324,
#25325,#25326,#25327,#25328,#25329,#25330,#25331,#25332,#25333,#25334,#25335,
#25336,#25337,#25338,#25339,#25340,#25341),(#25342,#25343,#25344,#25345,
#25346,#25347,#25348,#25349,#25350,#25351,#25352,#25353,#25354,#25355,#25356,
#25357,#25358,#25359,#25360,#25361,#25362,#25363,#25364,#25365,#25366,#25367,
#25368,#25369,#25370,#25371,#25372,#25373,#25374,#25375,#25376,#25377,#25378,
#25379,#25380,#25381,#25382,#25383,#25384,#25385,#25386,#25387,#25388,#25389,
#25390),(#25391,#25392,#25393,#25394,#25395,#25396,#25397,#25398,#25399,
#25400,#25401,#25402,#25403,#25404,#25405,#25406,#25407,#25408,#25409,#25410,
#25411,#25412,#25413,#25414,#25415,#25416,#25417,#25418,#25419,#25420,#25421,
#25422,#25423,#25424,#25425,#25426,#25427,#25428,#25429,#25430,#25431,#25432,
#25433,#25434,#25435,#25436,#25437,#25438,#25439),(#25440,#25441,#25442,
#25443,#25444,#25445,#25446,#25447,#25448,#25449,#25450,#25451,#25452,#25453,
#25454,#25455,#25456,#25457,#25458,#25459,#25460,#25461,#25462,#25463,#25464,
#25465,#25466,#25467,#25468,#25469,#25470,#25471,#25472,#25473,#25474,#25475,
#25476,#25477,#25478,#25479,#25480,#25481,#25482,#25483,#25484,#25485,#25486,
#25487,#25488),(#25489,#25490,#25491,#25492,#25493,#25494,#25495,#25496,
#25497,#25498,#25499,#25500,#25501,#25502,#25503,#25504,#25505,#25506,#25507,
#25508,#25509,#25510,#25511,#25512,#25513,#25514,#25515,#25516,#25517,#25518,
#25519,#25520,#25521,#25522,#25523,#25524,#25525,#25526,#25527,#25528,#25529,
#25530,#25531,#25532,#25533,#25534,#25535,#25536,#25537),(#25538,#25539,
#25540,#25541,#25542,#25543,#25544,#25545,#25546,#25547,#25548,#25549,#25550,
#25551,#25552,#25553,#25554,#25555,#25556,#25557,#25558,#25559,#25560,#25561,
#25562,#25563,#25564,#25565,#25566,#25567,#25568,#25569,#25570,#25571,#25572,
#25573,#25574,#25575,#25576,#25577,#25578,#25579,#25580,#25581,#25582,#25583,
#25584,#25585,#25586),(#25587,#25588,#25589,#25590,#25591,#25592,#25593,
#25594,#25595,#25596,#25597,#25598,#25599,#25600,#25601,#25602,#25603,#25604,
#25605,#25606,#25607,#25608,#25609,#25610,#25611,#25612,#25613,#25614,#25615,
#25616,#25617,#25618,#25619,#25620,#25621,#25622,#25623,#25624,#25625,#25626,
#25627,#25628,#25629,#25630,#25631,#25632,#25633,#25634,#25635),(#25636,
#25637,#25638,#25639,#25640,#25641,#25642,#25643,#25644,#25645,#25646,#25647,
#25648,#25649,#25650,#25651,#25652,#25653,#25654,#25655,#25656,#25657,#25658,
#25659,#25660,#25661,#25662,#25663,#25664,#25665,#25666,#25667,#25668,#25669,
#25670,#25671,#25672,#25673,#25674,#25675,#25676,#25677,#25678,#25679,#25680,
#25681,#25682,#25683,#25684),(#25685,#25686,#25687,#25688,#25689,#25690,
#25691,#25692,#25693,#25694,#25695,#25696,#25697,#25698,#25699,#25700,#25701,
#25702,#25703,#25704,#25705,#25706,#25707,#25708,#25709,#25710,#25711,#25712,
#25713,#25714,#25715,#25716,#25717,#25718,#25719,#25720,#25721,#25722,#25723,
#25724,#25725,#25726,#25727,#25728,#25729,#25730,#25731,#25732,#25733),
(#25734,#25735,#25736,#25737,#25738,#25739,#25740,#25741,#25742,#25743,
#25744,#25745,#25746,#25747,#25748,#25749,#25750,#25751,#25752,#25753,#25754,
#25755,#25756,#25757,#25758,#25759,#25760,#25761,#25762,#25763,#25764,#25765,
#25766,#25767,#25768,#25769,#25770,#25771,#25772,#25773,#25774,#25775,#25776,
#25777,#25778,#25779,#25780,#25781,#25782),(#25783,#25784,#25785,#25786,
#25787,#25788,#25789,#25790,#25791,#25792,#25793,#25794,#25795,#25796,#25797,
#25798,#25799,#25800,#25801,#25802,#25803,#25804,#25805,#25806,#25807,#25808,
#25809,#25810,#25811,#25812,#25813,#25814,#25815,#25816,#25817,#25818,#25819,
#25820,#25821,#25822,#25823,#25824,#25825,#25826,#25827,#25828,#25829,#25830,
#25831),(#25832,#25833,#25834,#25835,#25836,#25837,#25838,#25839,#25840,
#25841,#25842,#25843,#25844,#25845,#25846,#25847,#25848,#25849,#25850,#25851,
#25852,#25853,#25854,#25855,#25856,#25857,#25858,#25859,#25860,#25861,#25862,
#25863,#25864,#25865,#25866,#25867,#25868,#25869,#25870,#25871,#25872,#25873,
#25874,#25875,#25876,#25877,#25878,#25879,#25880),(#25881,#25882,#25883,
#25884,#25885,#25886,#25887,#25888,#25889,#25890,#25891,#25892,#25893,#25894,
#25895,#25896,#25897,#25898,#25899,#25900,#25901,#25902,#25903,#25904,#25905,
#25906,#25907,#25908,#25909,#25910,#25911,#25912,#25913,#25914,#25915,#25916,
#25917,#25918,#25919,#25920,#25921,#25922,#25923,#25924,#25925,#25926,#25927,
#25928,#25929),(#25930,#25931,#25932,#25933,#25934,#25935,#25936,#25937,
#25938,#25939,#25940,#25941,#25942,#25943,#25944,#25945,#25946,#25947,#25948,
#25949,#25950,#25951,#25952,#25953,#25954,#25955,#25956,#25957,#25958,#25959,
#25960,#25961,#25962,#25963,#25964,#25965,#25966,#25967,#25968,#25969,#25970,
#25971,#25972,#25973,#25974,#25975,#25976,#25977,#25978),(#25979,#25980,
#25981,#25982,#25983,#25984,#25985,#25986,#25987,#25988,#25989,#25990,#25991,
#25992,#25993,#25994,#25995,#25996,#25997,#25998,#25999,#26000,#26001,#26002,
#26003,#26004,#26005,#26006,#26007,#26008,#26009,#26010,#26011,#26012,#26013,
#26014,#26015,#26016,#26017,#26018,#26019,#26020,#26021,#26022,#26023,#26024,
#26025,#26026,#26027),(#26028,#26029,#26030,#26031,#26032,#26033,#26034,
#26035,#26036,#26037,#26038,#26039,#26040,#26041,#26042,#26043,#26044,#26045,
#26046,#26047,#26048,#26049,#26050,#26051,#26052,#26053,#26054,#26055,#26056,
#26057,#26058,#26059,#26060,#26061,#26062,#26063,#26064,#26065,#26066,#26067,
#26068,#26069,#26070,#26071,#26072,#26073,#26074,#26075,#26076),(#26077,
#26078,#26079,#26080,#26081,#26082,#26083,#26084,#26085,#26086,#26087,#26088,
#26089,#26090,#26091,#26092,#26093,#26094,#26095,#26096,#26097,#26098,#26099,
#26100,#26101,#26102,#26103,#26104,#26105,#26106,#26107,#26108,#26109,#26110,
#26111,#26112,#26113,#26114,#26115,#26116,#26117,#26118,#26119,#26120,#26121,
#26122,#26123,#26124,#26125),(#26126,#26127,#26128,#26129,#26130,#26131,
#26132,#26133,#26134,#26135,#26136,#26137,#26138,#26139,#26140,#26141,#26142,
#26143,#26144,#26145,#26146,#26147,#26148,#26149,#26150,#26151,#26152,#26153,
#26154,#26155,#26156,#26157,#26158,#26159,#26160,#26161,#26162,#26163,#26164,
#26165,#26166,#26167,#26168,#26169,#26170,#26171,#26172,#26173,#26174),
(#26175,#26176,#26177,#26178,#26179,#26180,#26181,#26182,#26183,#26184,
#26185,#26186,#26187,#26188,#26189,#26190,#26191,#26192,#26193,#26194,#26195,
#26196,#26197,#26198,#26199,#26200,#26201,#26202,#26203,#26204,#26205,#26206,
#26207,#26208,#26209,#26210,#26211,#26212,#26213,#26214,#26215,#26216,#26217,
#26218,#26219,#26220,#26221,#26222,#26223),(#26224,#26225,#26226,#26227,
#26228,#26229,#26230,#26231,#26232,#26233,#26234,#26235,#26236,#26237,#26238,
#26239,#26240,#26241,#26242,#26243,#26244,#26245,#26246,#26247,#26248,#26249,
#26250,#26251,#26252,#26253,#26254,#26255,#26256,#26257,#26258,#26259,#26260,
#26261,#26262,#26263,#26264,#26265,#26266,#26267,#26268,#26269,#26270,#26271,
#26272),(#26273,#26274,#26275,#26276,#26277,#26278,#26279,#26280,#26281,
#26282,#26283,#26284,#26285,#26286,#26287,#26288,#26289,#26290,#26291,#26292,
#26293,#26294,#26295,#26296,#26297,#26298,#26299,#26300,#26301,#26302,#26303,
#26304,#26305,#26306,#26307,#26308,#26309,#26310,#26311,#26312,#26313,#26314,
#26315,#26316,#26317,#26318,#26319,#26320,#26321),(#26322,#26323,#26324,
#26325,#26326,#26327,#26328,#26329,#26330,#26331,#26332,#26333,#26334,#26335,
#26336,#26337,#26338,#26339,#26340,#26341,#26342,#26343,#26344,#26345,#26346,
#26347,#26348,#26349,#26350,#26351,#26352,#26353,#26354,#26355,#26356,#26357,
#26358,#26359,#26360,#26361,#26362,#26363,#26364,#26365,#26366,#26367,#26368,
#26369,#26370),(#26371,#26372,#26373,#26374,#26375,#26376,#26377,#26378,
#26379,#26380,#26381,#26382,#26383,#26384,#26385,#26386,#26387,#26388,#26389,
#26390,#26391,#26392,#26393,#26394,#26395,#26396,#26397,#26398,#26399,#26400,
#26401,#26402,#26403,#26404,#26405,#26406,#26407,#26408,#26409,#26410,#26411,
#26412,#26413,#26414,#26415,#26416,#26417,#26418,#26419),(#26420,#26421,
#26422,#26423,#26424,#26425,#26426,#26427,#26428,#26429,#26430,#26431,#26432,
#26433,#26434,#26435,#26436,#26437,#26438,#26439,#26440,#26441,#26442,#26443,
#26444,#26445,#26446,#26447,#26448,#26449,#26450,#26451,#26452,#26453,#26454,
#26455,#26456,#26457,#26458,#26459,#26460,#26461,#26462,#26463,#26464,#26465,
#26466,#26467,#26468),(#26469,#26470,#26471,#26472,#26473,#26474,#26475,
#26476,#26477,#26478,#26479,#26480,#26481,#26482,#26483,#26484,#26485,#26486,
#26487,#26488,#26489,#26490,#26491,#26492,#26493,#26494,#26495,#26496,#26497,
#26498,#26499,#26500,#26501,#26502,#26503,#26504,#26505,#26506,#26507,#26508,
#26509,#26510,#26511,#26512,#26513,#26514,#26515,#26516,#26517),(#26518,
#26519,#26520,#26521,#26522,#26523,#26524,#26525,#26526,#26527,#26528,#26529,
#26530,#26531,#26532,#26533,#26534,#26535,#26536,#26537,#26538,#26539,#26540,
#26541,#26542,#26543,#26544,#26545,#26546,#26547,#26548,#26549,#26550,#26551,
#26552,#26553,#26554,#26555,#26556,#26557,#26558,#26559,#26560,#26561,#26562,
#26563,#26564,#26565,#26566),(#26567,#26568,#26569,#26570,#26571,#26572,
#26573,#26574,#26575,#26576,#26577,#26578,#26579,#26580,#26581,#26582,#26583,
#26584,#26585,#26586,#26587,#26588,#26589,#26590,#26591,#26592,#26593,#26594,
#26595,#26596,#26597,#26598,#26599,#26600,#26601,#26602,#26603,#26604,#26605,
#26606,#26607,#26608,#26609,#26610,#26611,#26612,#26613,#26614,#26615),
(#26616,#26617,#26618,#26619,#26620,#26621,#26622,#26623,#26624,#26625,
#26626,#26627,#26628,#26629,#26630,#26631,#26632,#26633,#26634,#26635,#26636,
#26637,#26638,#26639,#26640,#26641,#26642,#26643,#26644,#26645,#26646,#26647,
#26648,#26649,#26650,#26651,#26652,#26653,#26654,#26655,#26656,#26657,#26658,
#26659,#26660,#26661,#26662,#26663,#26664),(#26665,#26666,#26667,#26668,
#26669,#26670,#26671,#26672,#26673,#26674,#26675,#26676,#26677,#26678,#26679,
#26680,#26681,#26682,#26683,#26684,#26685,#26686,#26687,#26688,#26689,#26690,
#26691,#26692,#26693,#26694,#26695,#26696,#26697,#26698,#26699,#26700,#26701,
#26702,#26703,#26704,#26705,#26706,#26707,#26708,#26709,#26710,#26711,#26712,
#26713),(#26714,#26715,#26716,#26717,#26718,#26719,#26720,#26721,#26722,
#26723,#26724,#26725,#26726,#26727,#26728,#26729,#26730,#26731,#26732,#26733,
#26734,#26735,#26736,#26737,#26738,#26739,#26740,#26741,#26742,#26743,#26744,
#26745,#26746,#26747,#26748,#26749,#26750,#26751,#26752,#26753,#26754,#26755,
#26756,#26757,#26758,#26759,#26760,#26761,#26762),(#26763,#26764,#26765,
#26766,#26767,#26768,#26769,#26770,#26771,#26772,#26773,#26774,#26775,#26776,
#26777,#26778,#26779,#26780,#26781,#26782,#26783,#26784,#26785,#26786,#26787,
#26788,#26789,#26790,#26791,#26792,#26793,#26794,#26795,#26796,#26797,#26798,
#26799,#26800,#26801,#26802,#26803,#26804,#26805,#26806,#26807,#26808,#26809,
#26810,#26811),(#26812,#26813,#26814,#26815,#26816,#26817,#26818,#26819,
#26820,#26821,#26822,#26823,#26824,#26825,#26826,#26827,#26828,#26829,#26830,
#26831,#26832,#26833,#26834,#26835,#26836,#26837,#26838,#26839,#26840,#26841,
#26842,#26843,#26844,#26845,#26846,#26847,#26848,#26849,#26850,#26851,#26852,
#26853,#26854,#26855,#26856,#26857,#26858,#26859,#26860),(#26861,#26862,
#26863,#26864,#26865,#26866,#26867,#26868,#26869,#26870,#26871,#26872,#26873,
#26874,#26875,#26876,#26877,#26878,#26879,#26880,#26881,#26882,#26883,#26884,
#26885,#26886,#26887,#26888,#26889,#26890,#26891,#26892,#26893,#26894,#26895,
#26896,#26897,#26898,#26899,#26900,#26901,#26902,#26903,#26904,#26905,#26906,
#26907,#26908,#26909),(#26910,#26911,#26912,#26913,#26914,#26915,#26916,
#26917,#26918,#26919,#26920,#26921,#26922,#26923,#26924,#26925,#26926,#26927,
#26928,#26929,#26930,#26931,#26932,#26933,#26934,#26935,#26936,#26937,#26938,
#26939,#26940,#26941,#26942,#26943,#26944,#26945,#26946,#26947,#26948,#26949,
#26950,#26951,#26952,#26953,#26954,#26955,#26956,#26957,#26958),(#26959,
#26960,#26961,#26962,#26963,#26964,#26965,#26966,#26967,#26968,#26969,#26970,
#26971,#26972,#26973,#26974,#26975,#26976,#26977,#26978,#26979,#26980,#26981,
#26982,#26983,#26984,#26985,#26986,#26987,#26988,#26989,#26990,#26991,#26992,
#26993,#26994,#26995,#26996,#26997,#26998,#26999,#27000,#27001,#27002,#27003,
#27004,#27005,#27006,#27007),(#27008,#27009,#27010,#27011,#27012,#27013,
#27014,#27015,#27016,#27017,#27018,#27019,#27020,#27021,#27022,#27023,#27024,
#27025,#27026,#27027,#27028,#27029,#27030,#27031,#27032,#27033,#27034,#27035,
#27036,#27037,#27038,#27039,#27040,#27041,#27042,#27043,#27044,#27045,#27046,
#27047,#27048,#27049,#27050,#27051,#27052,#27053,#27054,#27055,#27056),
(#27057,#27058,#27059,#27060,#27061,#27062,#27063,#27064,#27065,#27066,
#27067,#27068,#27069,#27070,#27071,#27072,#27073,#27074,#27075,#27076,#27077,
#27078,#27079,#27080,#27081,#27082,#27083,#27084,#27085,#27086,#27087,#27088,
#27089,#27090,#27091,#27092,#27093,#27094,#27095,#27096,#27097,#27098,#27099,
#27100,#27101,#27102,#27103,#27104,#27105),(#27106,#27107,#27108,#27109,
#27110,#27111,#27112,#27113,#27114,#27115,#27116,#27117,#27118,#27119,#27120,
#27121,#27122,#27123,#27124,#27125,#27126,#27127,#27128,#27129,#27130,#27131,
#27132,#27133,#27134,#27135,#27136,#27137,#27138,#27139,#27140,#27141,#27142,
#27143,#27144,#27145,#27146,#27147,#27148,#27149,#27150,#27151,#27152,#27153,
#27154),(#27155,#27156,#27157,#27158,#27159,#27160,#27161,#27162,#27163,
#27164,#27165,#27166,#27167,#27168,#27169,#27170,#27171,#27172,#27173,#27174,
#27175,#27176,#27177,#27178,#27179,#27180,#27181,#27182,#27183,#27184,#27185,
#27186,#27187,#27188,#27189,#27190,#27191,#27192,#27193,#27194,#27195,#27196,
#27197,#27198,#27199,#27200,#27201,#27202,#27203),(#27204,#27205,#27206,
#27207,#27208,#27209,#27210,#27211,#27212,#27213,#27214,#27215,#27216,#27217,
#27218,#27219,#27220,#27221,#27222,#27223,#27224,#27225,#27226,#27227,#27228,
#27229,#27230,#27231,#27232,#27233,#27234,#27235,#27236,#27237,#27238,#27239,
#27240,#27241,#27242,#27243,#27244,#27245,#27246,#27247,#27248,#27249,#27250,
#27251,#27252),(#27253,#27254,#27255,#27256,#27257,#27258,#27259,#27260,
#27261,#27262,#27263,#27264,#27265,#27266,#27267,#27268,#27269,#27270,#27271,
#27272,#27273,#27274,#27275,#27276,#27277,#27278,#27279,#27280,#27281,#27282,
#27283,#27284,#27285,#27286,#27287,#27288,#27289,#27290,#27291,#27292,#27293,
#27294,#27295,#27296,#27297,#27298,#27299,#27300,#27301),(#27302,#27303,
#27304,#27305,#27306,#27307,#27308,#27309,#27310,#27311,#27312,#27313,#27314,
#27315,#27316,#27317,#27318,#27319,#27320,#27321,#27322,#27323,#27324,#27325,
#27326,#27327,#27328,#27329,#27330,#27331,#27332,#27333,#27334,#27335,#27336,
#27337,#27338,#27339,#27340,#27341,#27342,#27343,#27344,#27345,#27346,#27347,
#27348,#27349,#27350),(#27351,#27352,#27353,#27354,#27355,#27356,#27357,
#27358,#27359,#27360,#27361,#27362,#27363,#27364,#27365,#27366,#27367,#27368,
#27369,#27370,#27371,#27372,#27373,#27374,#27375,#27376,#27377,#27378,#27379,
#27380,#27381,#27382,#27383,#27384,#27385,#27386,#27387,#27388,#27389,#27390,
#27391,#27392,#27393,#27394,#27395,#27396,#27397,#27398,#27399),(#27400,
#27401,#27402,#27403,#27404,#27405,#27406,#27407,#27408,#27409,#27410,#27411,
#27412,#27413,#27414,#27415,#27416,#27417,#27418,#27419,#27420,#27421,#27422,
#27423,#27424,#27425,#27426,#27427,#27428,#27429,#27430,#27431,#27432,#27433,
#27434,#27435,#27436,#27437,#27438,#27439,#27440,#27441,#27442,#27443,#27444,
#27445,#27446,#27447,#27448),(#27449,#27450,#27451,#27452,#27453,#27454,
#27455,#27456,#27457,#27458,#27459,#27460,#27461,#27462,#27463,#27464,#27465,
#27466,#27467,#27468,#27469,#27470,#27471,#27472,#27473,#27474,#27475,#27476,
#27477,#27478,#27479,#27480,#27481,#27482,#27483,#27484,#27485,#27486,#27487,
#27488,#27489,#27490,#27491,#27492,#27493,#27494,#27495,#27496,#27497),
(#27498,#27499,#27500,#27501,#27502,#27503,#27504,#27505,#27506,#27507,
#27508,#27509,#27510,#27511,#27512,#27513,#27514,#27515,#27516,#27517,#27518,
#27519,#27520,#27521,#27522,#27523,#27524,#27525,#27526,#27527,#27528,#27529,
#27530,#27531,#27532,#27533,#27534,#27535,#27536,#27537,#27538,#27539,#27540,
#27541,#27542,#27543,#27544,#27545,#27546),(#27547,#27548,#27549,#27550,
#27551,#27552,#27553,#27554,#27555,#27556,#27557,#27558,#27559,#27560,#27561,
#27562,#27563,#27564,#27565,#27566,#27567,#27568,#27569,#27570,#27571,#27572,
#27573,#27574,#27575,#27576,#27577,#27578,#27579,#27580,#27581,#27582,#27583,
#27584,#27585,#27586,#27587,#27588,#27589,#27590,#27591,#27592,#27593,#27594,
#27595),(#27596,#27597,#27598,#27599,#27600,#27601,#27602,#27603,#27604,
#27605,#27606,#27607,#27608,#27609,#27610,#27611,#27612,#27613,#27614,#27615,
#27616,#27617,#27618,#27619,#27620,#27621,#27622,#27623,#27624,#27625,#27626,
#27627,#27628,#27629,#27630,#27631,#27632,#27633,#27634,#27635,#27636,#27637,
#27638,#27639,#27640,#27641,#27642,#27643,#27644)),.UNSPECIFIED.,.F.,.F.,
 .F.,(4,3,3,3,3,3,3,3,3,3,3,3,3,3,3,3,3,3,3,3,3,3,3,3,3,3,3,3,3,3,3,3,3,
3,3,3,3,3,3,3,4),(4,3,3,3,3,3,3,3,3,3,3,3,3,3,3,3,4),(-1.41424042909535E-5,
-3.89974880004448E-6,-1.33908492731722E-6,-5.87529909535886E-8,1.22157894541004E-6,
6.34290669086456E-6,2.68282176726826E-5,4.73135286545007E-5,6.77988396363188E-5,
8.82841506181369E-5,0.000108769461599955,0.000129254772581773,0.000149740083563591,
0.000190710705527227,0.000231681327490863,0.0002726519494545,0.000313622571418136,
0.000354593193381772,0.000395563815345408,0.00047750505927268,0.000559446303199953,
0.000641387547127225,0.000723328791054497,0.00080527003498177,0.000887211278909042,
0.000969152522836314,0.00113303501069086,0.0012969174985454,0.00146079998639995,
0.00162468247425449,0.00178856496210904,0.00195244744996358,0.00228021242567267,
0.00260797740138176,0.00293574237709085,0.00326350735279994,0.00359127232850903,
0.00391903730421812,0.00424680227992721,0.0045745672556363,0.00528564362815289),
(-5.55464210984207E-5,0.0625,0.125,0.1875,0.25,0.3125,0.375,0.4375,0.5,
0.5625,0.625,0.6875,0.75,0.8125,0.875,0.9375,1.),.UNSPECIFIED.);
#193=B_SPLINE_SURFACE_WITH_KNOTS('',3,3,((#27792,#27793,#27794,#27795,#27796,
#27797,#27798,#27799,#27800,#27801,#27802,#27803,#27804,#27805,#27806,#27807,
#27808,#27809,#27810,#27811,#27812,#27813,#27814,#27815,#27816,#27817,#27818,
#27819,#27820,#27821,#27822,#27823,#27824,#27825,#27826,#27827,#27828,#27829,
#27830,#27831,#27832,#27833,#27834,#27835,#27836,#27837,#27838,#27839,#27840),
(#27841,#27842,#27843,#27844,#27845,#27846,#27847,#27848,#27849,#27850,
#27851,#27852,#27853,#27854,#27855,#27856,#27857,#27858,#27859,#27860,#27861,
#27862,#27863,#27864,#27865,#27866,#27867,#27868,#27869,#27870,#27871,#27872,
#27873,#27874,#27875,#27876,#27877,#27878,#27879,#27880,#27881,#27882,#27883,
#27884,#27885,#27886,#27887,#27888,#27889),(#27890,#27891,#27892,#27893,
#27894,#27895,#27896,#27897,#27898,#27899,#27900,#27901,#27902,#27903,#27904,
#27905,#27906,#27907,#27908,#27909,#27910,#27911,#27912,#27913,#27914,#27915,
#27916,#27917,#27918,#27919,#27920,#27921,#27922,#27923,#27924,#27925,#27926,
#27927,#27928,#27929,#27930,#27931,#27932,#27933,#27934,#27935,#27936,#27937,
#27938),(#27939,#27940,#27941,#27942,#27943,#27944,#27945,#27946,#27947,
#27948,#27949,#27950,#27951,#27952,#27953,#27954,#27955,#27956,#27957,#27958,
#27959,#27960,#27961,#27962,#27963,#27964,#27965,#27966,#27967,#27968,#27969,
#27970,#27971,#27972,#27973,#27974,#27975,#27976,#27977,#27978,#27979,#27980,
#27981,#27982,#27983,#27984,#27985,#27986,#27987),(#27988,#27989,#27990,
#27991,#27992,#27993,#27994,#27995,#27996,#27997,#27998,#27999,#28000,#28001,
#28002,#28003,#28004,#28005,#28006,#28007,#28008,#28009,#28010,#28011,#28012,
#28013,#28014,#28015,#28016,#28017,#28018,#28019,#28020,#28021,#28022,#28023,
#28024,#28025,#28026,#28027,#28028,#28029,#28030,#28031,#28032,#28033,#28034,
#28035,#28036),(#28037,#28038,#28039,#28040,#28041,#28042,#28043,#28044,
#28045,#28046,#28047,#28048,#28049,#28050,#28051,#28052,#28053,#28054,#28055,
#28056,#28057,#28058,#28059,#28060,#28061,#28062,#28063,#28064,#28065,#28066,
#28067,#28068,#28069,#28070,#28071,#28072,#28073,#28074,#28075,#28076,#28077,
#28078,#28079,#28080,#28081,#28082,#28083,#28084,#28085),(#28086,#28087,
#28088,#28089,#28090,#28091,#28092,#28093,#28094,#28095,#28096,#28097,#28098,
#28099,#28100,#28101,#28102,#28103,#28104,#28105,#28106,#28107,#28108,#28109,
#28110,#28111,#28112,#28113,#28114,#28115,#28116,#28117,#28118,#28119,#28120,
#28121,#28122,#28123,#28124,#28125,#28126,#28127,#28128,#28129,#28130,#28131,
#28132,#28133,#28134),(#28135,#28136,#28137,#28138,#28139,#28140,#28141,
#28142,#28143,#28144,#28145,#28146,#28147,#28148,#28149,#28150,#28151,#28152,
#28153,#28154,#28155,#28156,#28157,#28158,#28159,#28160,#28161,#28162,#28163,
#28164,#28165,#28166,#28167,#28168,#28169,#28170,#28171,#28172,#28173,#28174,
#28175,#28176,#28177,#28178,#28179,#28180,#28181,#28182,#28183),(#28184,
#28185,#28186,#28187,#28188,#28189,#28190,#28191,#28192,#28193,#28194,#28195,
#28196,#28197,#28198,#28199,#28200,#28201,#28202,#28203,#28204,#28205,#28206,
#28207,#28208,#28209,#28210,#28211,#28212,#28213,#28214,#28215,#28216,#28217,
#28218,#28219,#28220,#28221,#28222,#28223,#28224,#28225,#28226,#28227,#28228,
#28229,#28230,#28231,#28232),(#28233,#28234,#28235,#28236,#28237,#28238,
#28239,#28240,#28241,#28242,#28243,#28244,#28245,#28246,#28247,#28248,#28249,
#28250,#28251,#28252,#28253,#28254,#28255,#28256,#28257,#28258,#28259,#28260,
#28261,#28262,#28263,#28264,#28265,#28266,#28267,#28268,#28269,#28270,#28271,
#28272,#28273,#28274,#28275,#28276,#28277,#28278,#28279,#28280,#28281),
(#28282,#28283,#28284,#28285,#28286,#28287,#28288,#28289,#28290,#28291,
#28292,#28293,#28294,#28295,#28296,#28297,#28298,#28299,#28300,#28301,#28302,
#28303,#28304,#28305,#28306,#28307,#28308,#28309,#28310,#28311,#28312,#28313,
#28314,#28315,#28316,#28317,#28318,#28319,#28320,#28321,#28322,#28323,#28324,
#28325,#28326,#28327,#28328,#28329,#28330),(#28331,#28332,#28333,#28334,
#28335,#28336,#28337,#28338,#28339,#28340,#28341,#28342,#28343,#28344,#28345,
#28346,#28347,#28348,#28349,#28350,#28351,#28352,#28353,#28354,#28355,#28356,
#28357,#28358,#28359,#28360,#28361,#28362,#28363,#28364,#28365,#28366,#28367,
#28368,#28369,#28370,#28371,#28372,#28373,#28374,#28375,#28376,#28377,#28378,
#28379),(#28380,#28381,#28382,#28383,#28384,#28385,#28386,#28387,#28388,
#28389,#28390,#28391,#28392,#28393,#28394,#28395,#28396,#28397,#28398,#28399,
#28400,#28401,#28402,#28403,#28404,#28405,#28406,#28407,#28408,#28409,#28410,
#28411,#28412,#28413,#28414,#28415,#28416,#28417,#28418,#28419,#28420,#28421,
#28422,#28423,#28424,#28425,#28426,#28427,#28428),(#28429,#28430,#28431,
#28432,#28433,#28434,#28435,#28436,#28437,#28438,#28439,#28440,#28441,#28442,
#28443,#28444,#28445,#28446,#28447,#28448,#28449,#28450,#28451,#28452,#28453,
#28454,#28455,#28456,#28457,#28458,#28459,#28460,#28461,#28462,#28463,#28464,
#28465,#28466,#28467,#28468,#28469,#28470,#28471,#28472,#28473,#28474,#28475,
#28476,#28477),(#28478,#28479,#28480,#28481,#28482,#28483,#28484,#28485,
#28486,#28487,#28488,#28489,#28490,#28491,#28492,#28493,#28494,#28495,#28496,
#28497,#28498,#28499,#28500,#28501,#28502,#28503,#28504,#28505,#28506,#28507,
#28508,#28509,#28510,#28511,#28512,#28513,#28514,#28515,#28516,#28517,#28518,
#28519,#28520,#28521,#28522,#28523,#28524,#28525,#28526),(#28527,#28528,
#28529,#28530,#28531,#28532,#28533,#28534,#28535,#28536,#28537,#28538,#28539,
#28540,#28541,#28542,#28543,#28544,#28545,#28546,#28547,#28548,#28549,#28550,
#28551,#28552,#28553,#28554,#28555,#28556,#28557,#28558,#28559,#28560,#28561,
#28562,#28563,#28564,#28565,#28566,#28567,#28568,#28569,#28570,#28571,#28572,
#28573,#28574,#28575),(#28576,#28577,#28578,#28579,#28580,#28581,#28582,
#28583,#28584,#28585,#28586,#28587,#28588,#28589,#28590,#28591,#28592,#28593,
#28594,#28595,#28596,#28597,#28598,#28599,#28600,#28601,#28602,#28603,#28604,
#28605,#28606,#28607,#28608,#28609,#28610,#28611,#28612,#28613,#28614,#28615,
#28616,#28617,#28618,#28619,#28620,#28621,#28622,#28623,#28624),(#28625,
#28626,#28627,#28628,#28629,#28630,#28631,#28632,#28633,#28634,#28635,#28636,
#28637,#28638,#28639,#28640,#28641,#28642,#28643,#28644,#28645,#28646,#28647,
#28648,#28649,#28650,#28651,#28652,#28653,#28654,#28655,#28656,#28657,#28658,
#28659,#28660,#28661,#28662,#28663,#28664,#28665,#28666,#28667,#28668,#28669,
#28670,#28671,#28672,#28673),(#28674,#28675,#28676,#28677,#28678,#28679,
#28680,#28681,#28682,#28683,#28684,#28685,#28686,#28687,#28688,#28689,#28690,
#28691,#28692,#28693,#28694,#28695,#28696,#28697,#28698,#28699,#28700,#28701,
#28702,#28703,#28704,#28705,#28706,#28707,#28708,#28709,#28710,#28711,#28712,
#28713,#28714,#28715,#28716,#28717,#28718,#28719,#28720,#28721,#28722),
(#28723,#28724,#28725,#28726,#28727,#28728,#28729,#28730,#28731,#28732,
#28733,#28734,#28735,#28736,#28737,#28738,#28739,#28740,#28741,#28742,#28743,
#28744,#28745,#28746,#28747,#28748,#28749,#28750,#28751,#28752,#28753,#28754,
#28755,#28756,#28757,#28758,#28759,#28760,#28761,#28762,#28763,#28764,#28765,
#28766,#28767,#28768,#28769,#28770,#28771),(#28772,#28773,#28774,#28775,
#28776,#28777,#28778,#28779,#28780,#28781,#28782,#28783,#28784,#28785,#28786,
#28787,#28788,#28789,#28790,#28791,#28792,#28793,#28794,#28795,#28796,#28797,
#28798,#28799,#28800,#28801,#28802,#28803,#28804,#28805,#28806,#28807,#28808,
#28809,#28810,#28811,#28812,#28813,#28814,#28815,#28816,#28817,#28818,#28819,
#28820),(#28821,#28822,#28823,#28824,#28825,#28826,#28827,#28828,#28829,
#28830,#28831,#28832,#28833,#28834,#28835,#28836,#28837,#28838,#28839,#28840,
#28841,#28842,#28843,#28844,#28845,#28846,#28847,#28848,#28849,#28850,#28851,
#28852,#28853,#28854,#28855,#28856,#28857,#28858,#28859,#28860,#28861,#28862,
#28863,#28864,#28865,#28866,#28867,#28868,#28869),(#28870,#28871,#28872,
#28873,#28874,#28875,#28876,#28877,#28878,#28879,#28880,#28881,#28882,#28883,
#28884,#28885,#28886,#28887,#28888,#28889,#28890,#28891,#28892,#28893,#28894,
#28895,#28896,#28897,#28898,#28899,#28900,#28901,#28902,#28903,#28904,#28905,
#28906,#28907,#28908,#28909,#28910,#28911,#28912,#28913,#28914,#28915,#28916,
#28917,#28918),(#28919,#28920,#28921,#28922,#28923,#28924,#28925,#28926,
#28927,#28928,#28929,#28930,#28931,#28932,#28933,#28934,#28935,#28936,#28937,
#28938,#28939,#28940,#28941,#28942,#28943,#28944,#28945,#28946,#28947,#28948,
#28949,#28950,#28951,#28952,#28953,#28954,#28955,#28956,#28957,#28958,#28959,
#28960,#28961,#28962,#28963,#28964,#28965,#28966,#28967),(#28968,#28969,
#28970,#28971,#28972,#28973,#28974,#28975,#28976,#28977,#28978,#28979,#28980,
#28981,#28982,#28983,#28984,#28985,#28986,#28987,#28988,#28989,#28990,#28991,
#28992,#28993,#28994,#28995,#28996,#28997,#28998,#28999,#29000,#29001,#29002,
#29003,#29004,#29005,#29006,#29007,#29008,#29009,#29010,#29011,#29012,#29013,
#29014,#29015,#29016),(#29017,#29018,#29019,#29020,#29021,#29022,#29023,
#29024,#29025,#29026,#29027,#29028,#29029,#29030,#29031,#29032,#29033,#29034,
#29035,#29036,#29037,#29038,#29039,#29040,#29041,#29042,#29043,#29044,#29045,
#29046,#29047,#29048,#29049,#29050,#29051,#29052,#29053,#29054,#29055,#29056,
#29057,#29058,#29059,#29060,#29061,#29062,#29063,#29064,#29065),(#29066,
#29067,#29068,#29069,#29070,#29071,#29072,#29073,#29074,#29075,#29076,#29077,
#29078,#29079,#29080,#29081,#29082,#29083,#29084,#29085,#29086,#29087,#29088,
#29089,#29090,#29091,#29092,#29093,#29094,#29095,#29096,#29097,#29098,#29099,
#29100,#29101,#29102,#29103,#29104,#29105,#29106,#29107,#29108,#29109,#29110,
#29111,#29112,#29113,#29114),(#29115,#29116,#29117,#29118,#29119,#29120,
#29121,#29122,#29123,#29124,#29125,#29126,#29127,#29128,#29129,#29130,#29131,
#29132,#29133,#29134,#29135,#29136,#29137,#29138,#29139,#29140,#29141,#29142,
#29143,#29144,#29145,#29146,#29147,#29148,#29149,#29150,#29151,#29152,#29153,
#29154,#29155,#29156,#29157,#29158,#29159,#29160,#29161,#29162,#29163),
(#29164,#29165,#29166,#29167,#29168,#29169,#29170,#29171,#29172,#29173,
#29174,#29175,#29176,#29177,#29178,#29179,#29180,#29181,#29182,#29183,#29184,
#29185,#29186,#29187,#29188,#29189,#29190,#29191,#29192,#29193,#29194,#29195,
#29196,#29197,#29198,#29199,#29200,#29201,#29202,#29203,#29204,#29205,#29206,
#29207,#29208,#29209,#29210,#29211,#29212),(#29213,#29214,#29215,#29216,
#29217,#29218,#29219,#29220,#29221,#29222,#29223,#29224,#29225,#29226,#29227,
#29228,#29229,#29230,#29231,#29232,#29233,#29234,#29235,#29236,#29237,#29238,
#29239,#29240,#29241,#29242,#29243,#29244,#29245,#29246,#29247,#29248,#29249,
#29250,#29251,#29252,#29253,#29254,#29255,#29256,#29257,#29258,#29259,#29260,
#29261),(#29262,#29263,#29264,#29265,#29266,#29267,#29268,#29269,#29270,
#29271,#29272,#29273,#29274,#29275,#29276,#29277,#29278,#29279,#29280,#29281,
#29282,#29283,#29284,#29285,#29286,#29287,#29288,#29289,#29290,#29291,#29292,
#29293,#29294,#29295,#29296,#29297,#29298,#29299,#29300,#29301,#29302,#29303,
#29304,#29305,#29306,#29307,#29308,#29309,#29310),(#29311,#29312,#29313,
#29314,#29315,#29316,#29317,#29318,#29319,#29320,#29321,#29322,#29323,#29324,
#29325,#29326,#29327,#29328,#29329,#29330,#29331,#29332,#29333,#29334,#29335,
#29336,#29337,#29338,#29339,#29340,#29341,#29342,#29343,#29344,#29345,#29346,
#29347,#29348,#29349,#29350,#29351,#29352,#29353,#29354,#29355,#29356,#29357,
#29358,#29359),(#29360,#29361,#29362,#29363,#29364,#29365,#29366,#29367,
#29368,#29369,#29370,#29371,#29372,#29373,#29374,#29375,#29376,#29377,#29378,
#29379,#29380,#29381,#29382,#29383,#29384,#29385,#29386,#29387,#29388,#29389,
#29390,#29391,#29392,#29393,#29394,#29395,#29396,#29397,#29398,#29399,#29400,
#29401,#29402,#29403,#29404,#29405,#29406,#29407,#29408),(#29409,#29410,
#29411,#29412,#29413,#29414,#29415,#29416,#29417,#29418,#29419,#29420,#29421,
#29422,#29423,#29424,#29425,#29426,#29427,#29428,#29429,#29430,#29431,#29432,
#29433,#29434,#29435,#29436,#29437,#29438,#29439,#29440,#29441,#29442,#29443,
#29444,#29445,#29446,#29447,#29448,#29449,#29450,#29451,#29452,#29453,#29454,
#29455,#29456,#29457),(#29458,#29459,#29460,#29461,#29462,#29463,#29464,
#29465,#29466,#29467,#29468,#29469,#29470,#29471,#29472,#29473,#29474,#29475,
#29476,#29477,#29478,#29479,#29480,#29481,#29482,#29483,#29484,#29485,#29486,
#29487,#29488,#29489,#29490,#29491,#29492,#29493,#29494,#29495,#29496,#29497,
#29498,#29499,#29500,#29501,#29502,#29503,#29504,#29505,#29506),(#29507,
#29508,#29509,#29510,#29511,#29512,#29513,#29514,#29515,#29516,#29517,#29518,
#29519,#29520,#29521,#29522,#29523,#29524,#29525,#29526,#29527,#29528,#29529,
#29530,#29531,#29532,#29533,#29534,#29535,#29536,#29537,#29538,#29539,#29540,
#29541,#29542,#29543,#29544,#29545,#29546,#29547,#29548,#29549,#29550,#29551,
#29552,#29553,#29554,#29555),(#29556,#29557,#29558,#29559,#29560,#29561,
#29562,#29563,#29564,#29565,#29566,#29567,#29568,#29569,#29570,#29571,#29572,
#29573,#29574,#29575,#29576,#29577,#29578,#29579,#29580,#29581,#29582,#29583,
#29584,#29585,#29586,#29587,#29588,#29589,#29590,#29591,#29592,#29593,#29594,
#29595,#29596,#29597,#29598,#29599,#29600,#29601,#29602,#29603,#29604),
(#29605,#29606,#29607,#29608,#29609,#29610,#29611,#29612,#29613,#29614,
#29615,#29616,#29617,#29618,#29619,#29620,#29621,#29622,#29623,#29624,#29625,
#29626,#29627,#29628,#29629,#29630,#29631,#29632,#29633,#29634,#29635,#29636,
#29637,#29638,#29639,#29640,#29641,#29642,#29643,#29644,#29645,#29646,#29647,
#29648,#29649,#29650,#29651,#29652,#29653),(#29654,#29655,#29656,#29657,
#29658,#29659,#29660,#29661,#29662,#29663,#29664,#29665,#29666,#29667,#29668,
#29669,#29670,#29671,#29672,#29673,#29674,#29675,#29676,#29677,#29678,#29679,
#29680,#29681,#29682,#29683,#29684,#29685,#29686,#29687,#29688,#29689,#29690,
#29691,#29692,#29693,#29694,#29695,#29696,#29697,#29698,#29699,#29700,#29701,
#29702),(#29703,#29704,#29705,#29706,#29707,#29708,#29709,#29710,#29711,
#29712,#29713,#29714,#29715,#29716,#29717,#29718,#29719,#29720,#29721,#29722,
#29723,#29724,#29725,#29726,#29727,#29728,#29729,#29730,#29731,#29732,#29733,
#29734,#29735,#29736,#29737,#29738,#29739,#29740,#29741,#29742,#29743,#29744,
#29745,#29746,#29747,#29748,#29749,#29750,#29751),(#29752,#29753,#29754,
#29755,#29756,#29757,#29758,#29759,#29760,#29761,#29762,#29763,#29764,#29765,
#29766,#29767,#29768,#29769,#29770,#29771,#29772,#29773,#29774,#29775,#29776,
#29777,#29778,#29779,#29780,#29781,#29782,#29783,#29784,#29785,#29786,#29787,
#29788,#29789,#29790,#29791,#29792,#29793,#29794,#29795,#29796,#29797,#29798,
#29799,#29800),(#29801,#29802,#29803,#29804,#29805,#29806,#29807,#29808,
#29809,#29810,#29811,#29812,#29813,#29814,#29815,#29816,#29817,#29818,#29819,
#29820,#29821,#29822,#29823,#29824,#29825,#29826,#29827,#29828,#29829,#29830,
#29831,#29832,#29833,#29834,#29835,#29836,#29837,#29838,#29839,#29840,#29841,
#29842,#29843,#29844,#29845,#29846,#29847,#29848,#29849),(#29850,#29851,
#29852,#29853,#29854,#29855,#29856,#29857,#29858,#29859,#29860,#29861,#29862,
#29863,#29864,#29865,#29866,#29867,#29868,#29869,#29870,#29871,#29872,#29873,
#29874,#29875,#29876,#29877,#29878,#29879,#29880,#29881,#29882,#29883,#29884,
#29885,#29886,#29887,#29888,#29889,#29890,#29891,#29892,#29893,#29894,#29895,
#29896,#29897,#29898),(#29899,#29900,#29901,#29902,#29903,#29904,#29905,
#29906,#29907,#29908,#29909,#29910,#29911,#29912,#29913,#29914,#29915,#29916,
#29917,#29918,#29919,#29920,#29921,#29922,#29923,#29924,#29925,#29926,#29927,
#29928,#29929,#29930,#29931,#29932,#29933,#29934,#29935,#29936,#29937,#29938,
#29939,#29940,#29941,#29942,#29943,#29944,#29945,#29946,#29947),(#29948,
#29949,#29950,#29951,#29952,#29953,#29954,#29955,#29956,#29957,#29958,#29959,
#29960,#29961,#29962,#29963,#29964,#29965,#29966,#29967,#29968,#29969,#29970,
#29971,#29972,#29973,#29974,#29975,#29976,#29977,#29978,#29979,#29980,#29981,
#29982,#29983,#29984,#29985,#29986,#29987,#29988,#29989,#29990,#29991,#29992,
#29993,#29994,#29995,#29996),(#29997,#29998,#29999,#30000,#30001,#30002,
#30003,#30004,#30005,#30006,#30007,#30008,#30009,#30010,#30011,#30012,#30013,
#30014,#30015,#30016,#30017,#30018,#30019,#30020,#30021,#30022,#30023,#30024,
#30025,#30026,#30027,#30028,#30029,#30030,#30031,#30032,#30033,#30034,#30035,
#30036,#30037,#30038,#30039,#30040,#30041,#30042,#30043,#30044,#30045),
(#30046,#30047,#30048,#30049,#30050,#30051,#30052,#30053,#30054,#30055,
#30056,#30057,#30058,#30059,#30060,#30061,#30062,#30063,#30064,#30065,#30066,
#30067,#30068,#30069,#30070,#30071,#30072,#30073,#30074,#30075,#30076,#30077,
#30078,#30079,#30080,#30081,#30082,#30083,#30084,#30085,#30086,#30087,#30088,
#30089,#30090,#30091,#30092,#30093,#30094),(#30095,#30096,#30097,#30098,
#30099,#30100,#30101,#30102,#30103,#30104,#30105,#30106,#30107,#30108,#30109,
#30110,#30111,#30112,#30113,#30114,#30115,#30116,#30117,#30118,#30119,#30120,
#30121,#30122,#30123,#30124,#30125,#30126,#30127,#30128,#30129,#30130,#30131,
#30132,#30133,#30134,#30135,#30136,#30137,#30138,#30139,#30140,#30141,#30142,
#30143),(#30144,#30145,#30146,#30147,#30148,#30149,#30150,#30151,#30152,
#30153,#30154,#30155,#30156,#30157,#30158,#30159,#30160,#30161,#30162,#30163,
#30164,#30165,#30166,#30167,#30168,#30169,#30170,#30171,#30172,#30173,#30174,
#30175,#30176,#30177,#30178,#30179,#30180,#30181,#30182,#30183,#30184,#30185,
#30186,#30187,#30188,#30189,#30190,#30191,#30192),(#30193,#30194,#30195,
#30196,#30197,#30198,#30199,#30200,#30201,#30202,#30203,#30204,#30205,#30206,
#30207,#30208,#30209,#30210,#30211,#30212,#30213,#30214,#30215,#30216,#30217,
#30218,#30219,#30220,#30221,#30222,#30223,#30224,#30225,#30226,#30227,#30228,
#30229,#30230,#30231,#30232,#30233,#30234,#30235,#30236,#30237,#30238,#30239,
#30240,#30241),(#30242,#30243,#30244,#30245,#30246,#30247,#30248,#30249,
#30250,#30251,#30252,#30253,#30254,#30255,#30256,#30257,#30258,#30259,#30260,
#30261,#30262,#30263,#30264,#30265,#30266,#30267,#30268,#30269,#30270,#30271,
#30272,#30273,#30274,#30275,#30276,#30277,#30278,#30279,#30280,#30281,#30282,
#30283,#30284,#30285,#30286,#30287,#30288,#30289,#30290),(#30291,#30292,
#30293,#30294,#30295,#30296,#30297,#30298,#30299,#30300,#30301,#30302,#30303,
#30304,#30305,#30306,#30307,#30308,#30309,#30310,#30311,#30312,#30313,#30314,
#30315,#30316,#30317,#30318,#30319,#30320,#30321,#30322,#30323,#30324,#30325,
#30326,#30327,#30328,#30329,#30330,#30331,#30332,#30333,#30334,#30335,#30336,
#30337,#30338,#30339),(#30340,#30341,#30342,#30343,#30344,#30345,#30346,
#30347,#30348,#30349,#30350,#30351,#30352,#30353,#30354,#30355,#30356,#30357,
#30358,#30359,#30360,#30361,#30362,#30363,#30364,#30365,#30366,#30367,#30368,
#30369,#30370,#30371,#30372,#30373,#30374,#30375,#30376,#30377,#30378,#30379,
#30380,#30381,#30382,#30383,#30384,#30385,#30386,#30387,#30388),(#30389,
#30390,#30391,#30392,#30393,#30394,#30395,#30396,#30397,#30398,#30399,#30400,
#30401,#30402,#30403,#30404,#30405,#30406,#30407,#30408,#30409,#30410,#30411,
#30412,#30413,#30414,#30415,#30416,#30417,#30418,#30419,#30420,#30421,#30422,
#30423,#30424,#30425,#30426,#30427,#30428,#30429,#30430,#30431,#30432,#30433,
#30434,#30435,#30436,#30437),(#30438,#30439,#30440,#30441,#30442,#30443,
#30444,#30445,#30446,#30447,#30448,#30449,#30450,#30451,#30452,#30453,#30454,
#30455,#30456,#30457,#30458,#30459,#30460,#30461,#30462,#30463,#30464,#30465,
#30466,#30467,#30468,#30469,#30470,#30471,#30472,#30473,#30474,#30475,#30476,
#30477,#30478,#30479,#30480,#30481,#30482,#30483,#30484,#30485,#30486),
(#30487,#30488,#30489,#30490,#30491,#30492,#30493,#30494,#30495,#30496,
#30497,#30498,#30499,#30500,#30501,#30502,#30503,#30504,#30505,#30506,#30507,
#30508,#30509,#30510,#30511,#30512,#30513,#30514,#30515,#30516,#30517,#30518,
#30519,#30520,#30521,#30522,#30523,#30524,#30525,#30526,#30527,#30528,#30529,
#30530,#30531,#30532,#30533,#30534,#30535),(#30536,#30537,#30538,#30539,
#30540,#30541,#30542,#30543,#30544,#30545,#30546,#30547,#30548,#30549,#30550,
#30551,#30552,#30553,#30554,#30555,#30556,#30557,#30558,#30559,#30560,#30561,
#30562,#30563,#30564,#30565,#30566,#30567,#30568,#30569,#30570,#30571,#30572,
#30573,#30574,#30575,#30576,#30577,#30578,#30579,#30580,#30581,#30582,#30583,
#30584),(#30585,#30586,#30587,#30588,#30589,#30590,#30591,#30592,#30593,
#30594,#30595,#30596,#30597,#30598,#30599,#30600,#30601,#30602,#30603,#30604,
#30605,#30606,#30607,#30608,#30609,#30610,#30611,#30612,#30613,#30614,#30615,
#30616,#30617,#30618,#30619,#30620,#30621,#30622,#30623,#30624,#30625,#30626,
#30627,#30628,#30629,#30630,#30631,#30632,#30633),(#30634,#30635,#30636,
#30637,#30638,#30639,#30640,#30641,#30642,#30643,#30644,#30645,#30646,#30647,
#30648,#30649,#30650,#30651,#30652,#30653,#30654,#30655,#30656,#30657,#30658,
#30659,#30660,#30661,#30662,#30663,#30664,#30665,#30666,#30667,#30668,#30669,
#30670,#30671,#30672,#30673,#30674,#30675,#30676,#30677,#30678,#30679,#30680,
#30681,#30682),(#30683,#30684,#30685,#30686,#30687,#30688,#30689,#30690,
#30691,#30692,#30693,#30694,#30695,#30696,#30697,#30698,#30699,#30700,#30701,
#30702,#30703,#30704,#30705,#30706,#30707,#30708,#30709,#30710,#30711,#30712,
#30713,#30714,#30715,#30716,#30717,#30718,#30719,#30720,#30721,#30722,#30723,
#30724,#30725,#30726,#30727,#30728,#30729,#30730,#30731),(#30732,#30733,
#30734,#30735,#30736,#30737,#30738,#30739,#30740,#30741,#30742,#30743,#30744,
#30745,#30746,#30747,#30748,#30749,#30750,#30751,#30752,#30753,#30754,#30755,
#30756,#30757,#30758,#30759,#30760,#30761,#30762,#30763,#30764,#30765,#30766,
#30767,#30768,#30769,#30770,#30771,#30772,#30773,#30774,#30775,#30776,#30777,
#30778,#30779,#30780),(#30781,#30782,#30783,#30784,#30785,#30786,#30787,
#30788,#30789,#30790,#30791,#30792,#30793,#30794,#30795,#30796,#30797,#30798,
#30799,#30800,#30801,#30802,#30803,#30804,#30805,#30806,#30807,#30808,#30809,
#30810,#30811,#30812,#30813,#30814,#30815,#30816,#30817,#30818,#30819,#30820,
#30821,#30822,#30823,#30824,#30825,#30826,#30827,#30828,#30829),(#30830,
#30831,#30832,#30833,#30834,#30835,#30836,#30837,#30838,#30839,#30840,#30841,
#30842,#30843,#30844,#30845,#30846,#30847,#30848,#30849,#30850,#30851,#30852,
#30853,#30854,#30855,#30856,#30857,#30858,#30859,#30860,#30861,#30862,#30863,
#30864,#30865,#30866,#30867,#30868,#30869,#30870,#30871,#30872,#30873,#30874,
#30875,#30876,#30877,#30878),(#30879,#30880,#30881,#30882,#30883,#30884,
#30885,#30886,#30887,#30888,#30889,#30890,#30891,#30892,#30893,#30894,#30895,
#30896,#30897,#30898,#30899,#30900,#30901,#30902,#30903,#30904,#30905,#30906,
#30907,#30908,#30909,#30910,#30911,#30912,#30913,#30914,#30915,#30916,#30917,
#30918,#30919,#30920,#30921,#30922,#30923,#30924,#30925,#30926,#30927),
(#30928,#30929,#30930,#30931,#30932,#30933,#30934,#30935,#30936,#30937,
#30938,#30939,#30940,#30941,#30942,#30943,#30944,#30945,#30946,#30947,#30948,
#30949,#30950,#30951,#30952,#30953,#30954,#30955,#30956,#30957,#30958,#30959,
#30960,#30961,#30962,#30963,#30964,#30965,#30966,#30967,#30968,#30969,#30970,
#30971,#30972,#30973,#30974,#30975,#30976),(#30977,#30978,#30979,#30980,
#30981,#30982,#30983,#30984,#30985,#30986,#30987,#30988,#30989,#30990,#30991,
#30992,#30993,#30994,#30995,#30996,#30997,#30998,#30999,#31000,#31001,#31002,
#31003,#31004,#31005,#31006,#31007,#31008,#31009,#31010,#31011,#31012,#31013,
#31014,#31015,#31016,#31017,#31018,#31019,#31020,#31021,#31022,#31023,#31024,
#31025),(#31026,#31027,#31028,#31029,#31030,#31031,#31032,#31033,#31034,
#31035,#31036,#31037,#31038,#31039,#31040,#31041,#31042,#31043,#31044,#31045,
#31046,#31047,#31048,#31049,#31050,#31051,#31052,#31053,#31054,#31055,#31056,
#31057,#31058,#31059,#31060,#31061,#31062,#31063,#31064,#31065,#31066,#31067,
#31068,#31069,#31070,#31071,#31072,#31073,#31074),(#31075,#31076,#31077,
#31078,#31079,#31080,#31081,#31082,#31083,#31084,#31085,#31086,#31087,#31088,
#31089,#31090,#31091,#31092,#31093,#31094,#31095,#31096,#31097,#31098,#31099,
#31100,#31101,#31102,#31103,#31104,#31105,#31106,#31107,#31108,#31109,#31110,
#31111,#31112,#31113,#31114,#31115,#31116,#31117,#31118,#31119,#31120,#31121,
#31122,#31123),(#31124,#31125,#31126,#31127,#31128,#31129,#31130,#31131,
#31132,#31133,#31134,#31135,#31136,#31137,#31138,#31139,#31140,#31141,#31142,
#31143,#31144,#31145,#31146,#31147,#31148,#31149,#31150,#31151,#31152,#31153,
#31154,#31155,#31156,#31157,#31158,#31159,#31160,#31161,#31162,#31163,#31164,
#31165,#31166,#31167,#31168,#31169,#31170,#31171,#31172),(#31173,#31174,
#31175,#31176,#31177,#31178,#31179,#31180,#31181,#31182,#31183,#31184,#31185,
#31186,#31187,#31188,#31189,#31190,#31191,#31192,#31193,#31194,#31195,#31196,
#31197,#31198,#31199,#31200,#31201,#31202,#31203,#31204,#31205,#31206,#31207,
#31208,#31209,#31210,#31211,#31212,#31213,#31214,#31215,#31216,#31217,#31218,
#31219,#31220,#31221),(#31222,#31223,#31224,#31225,#31226,#31227,#31228,
#31229,#31230,#31231,#31232,#31233,#31234,#31235,#31236,#31237,#31238,#31239,
#31240,#31241,#31242,#31243,#31244,#31245,#31246,#31247,#31248,#31249,#31250,
#31251,#31252,#31253,#31254,#31255,#31256,#31257,#31258,#31259,#31260,#31261,
#31262,#31263,#31264,#31265,#31266,#31267,#31268,#31269,#31270),(#31271,
#31272,#31273,#31274,#31275,#31276,#31277,#31278,#31279,#31280,#31281,#31282,
#31283,#31284,#31285,#31286,#31287,#31288,#31289,#31290,#31291,#31292,#31293,
#31294,#31295,#31296,#31297,#31298,#31299,#31300,#31301,#31302,#31303,#31304,
#31305,#31306,#31307,#31308,#31309,#31310,#31311,#31312,#31313,#31314,#31315,
#31316,#31317,#31318,#31319),(#31320,#31321,#31322,#31323,#31324,#31325,
#31326,#31327,#31328,#31329,#31330,#31331,#31332,#31333,#31334,#31335,#31336,
#31337,#31338,#31339,#31340,#31341,#31342,#31343,#31344,#31345,#31346,#31347,
#31348,#31349,#31350,#31351,#31352,#31353,#31354,#31355,#31356,#31357,#31358,
#31359,#31360,#31361,#31362,#31363,#31364,#31365,#31366,#31367,#31368),
(#31369,#31370,#31371,#31372,#31373,#31374,#31375,#31376,#31377,#31378,
#31379,#31380,#31381,#31382,#31383,#31384,#31385,#31386,#31387,#31388,#31389,
#31390,#31391,#31392,#31393,#31394,#31395,#31396,#31397,#31398,#31399,#31400,
#31401,#31402,#31403,#31404,#31405,#31406,#31407,#31408,#31409,#31410,#31411,
#31412,#31413,#31414,#31415,#31416,#31417),(#31418,#31419,#31420,#31421,
#31422,#31423,#31424,#31425,#31426,#31427,#31428,#31429,#31430,#31431,#31432,
#31433,#31434,#31435,#31436,#31437,#31438,#31439,#31440,#31441,#31442,#31443,
#31444,#31445,#31446,#31447,#31448,#31449,#31450,#31451,#31452,#31453,#31454,
#31455,#31456,#31457,#31458,#31459,#31460,#31461,#31462,#31463,#31464,#31465,
#31466),(#31467,#31468,#31469,#31470,#31471,#31472,#31473,#31474,#31475,
#31476,#31477,#31478,#31479,#31480,#31481,#31482,#31483,#31484,#31485,#31486,
#31487,#31488,#31489,#31490,#31491,#31492,#31493,#31494,#31495,#31496,#31497,
#31498,#31499,#31500,#31501,#31502,#31503,#31504,#31505,#31506,#31507,#31508,
#31509,#31510,#31511,#31512,#31513,#31514,#31515),(#31516,#31517,#31518,
#31519,#31520,#31521,#31522,#31523,#31524,#31525,#31526,#31527,#31528,#31529,
#31530,#31531,#31532,#31533,#31534,#31535,#31536,#31537,#31538,#31539,#31540,
#31541,#31542,#31543,#31544,#31545,#31546,#31547,#31548,#31549,#31550,#31551,
#31552,#31553,#31554,#31555,#31556,#31557,#31558,#31559,#31560,#31561,#31562,
#31563,#31564),(#31565,#31566,#31567,#31568,#31569,#31570,#31571,#31572,
#31573,#31574,#31575,#31576,#31577,#31578,#31579,#31580,#31581,#31582,#31583,
#31584,#31585,#31586,#31587,#31588,#31589,#31590,#31591,#31592,#31593,#31594,
#31595,#31596,#31597,#31598,#31599,#31600,#31601,#31602,#31603,#31604,#31605,
#31606,#31607,#31608,#31609,#31610,#31611,#31612,#31613),(#31614,#31615,
#31616,#31617,#31618,#31619,#31620,#31621,#31622,#31623,#31624,#31625,#31626,
#31627,#31628,#31629,#31630,#31631,#31632,#31633,#31634,#31635,#31636,#31637,
#31638,#31639,#31640,#31641,#31642,#31643,#31644,#31645,#31646,#31647,#31648,
#31649,#31650,#31651,#31652,#31653,#31654,#31655,#31656,#31657,#31658,#31659,
#31660,#31661,#31662),(#31663,#31664,#31665,#31666,#31667,#31668,#31669,
#31670,#31671,#31672,#31673,#31674,#31675,#31676,#31677,#31678,#31679,#31680,
#31681,#31682,#31683,#31684,#31685,#31686,#31687,#31688,#31689,#31690,#31691,
#31692,#31693,#31694,#31695,#31696,#31697,#31698,#31699,#31700,#31701,#31702,
#31703,#31704,#31705,#31706,#31707,#31708,#31709,#31710,#31711),(#31712,
#31713,#31714,#31715,#31716,#31717,#31718,#31719,#31720,#31721,#31722,#31723,
#31724,#31725,#31726,#31727,#31728,#31729,#31730,#31731,#31732,#31733,#31734,
#31735,#31736,#31737,#31738,#31739,#31740,#31741,#31742,#31743,#31744,#31745,
#31746,#31747,#31748,#31749,#31750,#31751,#31752,#31753,#31754,#31755,#31756,
#31757,#31758,#31759,#31760),(#31761,#31762,#31763,#31764,#31765,#31766,
#31767,#31768,#31769,#31770,#31771,#31772,#31773,#31774,#31775,#31776,#31777,
#31778,#31779,#31780,#31781,#31782,#31783,#31784,#31785,#31786,#31787,#31788,
#31789,#31790,#31791,#31792,#31793,#31794,#31795,#31796,#31797,#31798,#31799,
#31800,#31801,#31802,#31803,#31804,#31805,#31806,#31807,#31808,#31809),
(#31810,#31811,#31812,#31813,#31814,#31815,#31816,#31817,#31818,#31819,
#31820,#31821,#31822,#31823,#31824,#31825,#31826,#31827,#31828,#31829,#31830,
#31831,#31832,#31833,#31834,#31835,#31836,#31837,#31838,#31839,#31840,#31841,
#31842,#31843,#31844,#31845,#31846,#31847,#31848,#31849,#31850,#31851,#31852,
#31853,#31854,#31855,#31856,#31857,#31858),(#31859,#31860,#31861,#31862,
#31863,#31864,#31865,#31866,#31867,#31868,#31869,#31870,#31871,#31872,#31873,
#31874,#31875,#31876,#31877,#31878,#31879,#31880,#31881,#31882,#31883,#31884,
#31885,#31886,#31887,#31888,#31889,#31890,#31891,#31892,#31893,#31894,#31895,
#31896,#31897,#31898,#31899,#31900,#31901,#31902,#31903,#31904,#31905,#31906,
#31907),(#31908,#31909,#31910,#31911,#31912,#31913,#31914,#31915,#31916,
#31917,#31918,#31919,#31920,#31921,#31922,#31923,#31924,#31925,#31926,#31927,
#31928,#31929,#31930,#31931,#31932,#31933,#31934,#31935,#31936,#31937,#31938,
#31939,#31940,#31941,#31942,#31943,#31944,#31945,#31946,#31947,#31948,#31949,
#31950,#31951,#31952,#31953,#31954,#31955,#31956),(#31957,#31958,#31959,
#31960,#31961,#31962,#31963,#31964,#31965,#31966,#31967,#31968,#31969,#31970,
#31971,#31972,#31973,#31974,#31975,#31976,#31977,#31978,#31979,#31980,#31981,
#31982,#31983,#31984,#31985,#31986,#31987,#31988,#31989,#31990,#31991,#31992,
#31993,#31994,#31995,#31996,#31997,#31998,#31999,#32000,#32001,#32002,#32003,
#32004,#32005),(#32006,#32007,#32008,#32009,#32010,#32011,#32012,#32013,
#32014,#32015,#32016,#32017,#32018,#32019,#32020,#32021,#32022,#32023,#32024,
#32025,#32026,#32027,#32028,#32029,#32030,#32031,#32032,#32033,#32034,#32035,
#32036,#32037,#32038,#32039,#32040,#32041,#32042,#32043,#32044,#32045,#32046,
#32047,#32048,#32049,#32050,#32051,#32052,#32053,#32054),(#32055,#32056,
#32057,#32058,#32059,#32060,#32061,#32062,#32063,#32064,#32065,#32066,#32067,
#32068,#32069,#32070,#32071,#32072,#32073,#32074,#32075,#32076,#32077,#32078,
#32079,#32080,#32081,#32082,#32083,#32084,#32085,#32086,#32087,#32088,#32089,
#32090,#32091,#32092,#32093,#32094,#32095,#32096,#32097,#32098,#32099,#32100,
#32101,#32102,#32103),(#32104,#32105,#32106,#32107,#32108,#32109,#32110,
#32111,#32112,#32113,#32114,#32115,#32116,#32117,#32118,#32119,#32120,#32121,
#32122,#32123,#32124,#32125,#32126,#32127,#32128,#32129,#32130,#32131,#32132,
#32133,#32134,#32135,#32136,#32137,#32138,#32139,#32140,#32141,#32142,#32143,
#32144,#32145,#32146,#32147,#32148,#32149,#32150,#32151,#32152),(#32153,
#32154,#32155,#32156,#32157,#32158,#32159,#32160,#32161,#32162,#32163,#32164,
#32165,#32166,#32167,#32168,#32169,#32170,#32171,#32172,#32173,#32174,#32175,
#32176,#32177,#32178,#32179,#32180,#32181,#32182,#32183,#32184,#32185,#32186,
#32187,#32188,#32189,#32190,#32191,#32192,#32193,#32194,#32195,#32196,#32197,
#32198,#32199,#32200,#32201),(#32202,#32203,#32204,#32205,#32206,#32207,
#32208,#32209,#32210,#32211,#32212,#32213,#32214,#32215,#32216,#32217,#32218,
#32219,#32220,#32221,#32222,#32223,#32224,#32225,#32226,#32227,#32228,#32229,
#32230,#32231,#32232,#32233,#32234,#32235,#32236,#32237,#32238,#32239,#32240,
#32241,#32242,#32243,#32244,#32245,#32246,#32247,#32248,#32249,#32250),
(#32251,#32252,#32253,#32254,#32255,#32256,#32257,#32258,#32259,#32260,
#32261,#32262,#32263,#32264,#32265,#32266,#32267,#32268,#32269,#32270,#32271,
#32272,#32273,#32274,#32275,#32276,#32277,#32278,#32279,#32280,#32281,#32282,
#32283,#32284,#32285,#32286,#32287,#32288,#32289,#32290,#32291,#32292,#32293,
#32294,#32295,#32296,#32297,#32298,#32299),(#32300,#32301,#32302,#32303,
#32304,#32305,#32306,#32307,#32308,#32309,#32310,#32311,#32312,#32313,#32314,
#32315,#32316,#32317,#32318,#32319,#32320,#32321,#32322,#32323,#32324,#32325,
#32326,#32327,#32328,#32329,#32330,#32331,#32332,#32333,#32334,#32335,#32336,
#32337,#32338,#32339,#32340,#32341,#32342,#32343,#32344,#32345,#32346,#32347,
#32348),(#32349,#32350,#32351,#32352,#32353,#32354,#32355,#32356,#32357,
#32358,#32359,#32360,#32361,#32362,#32363,#32364,#32365,#32366,#32367,#32368,
#32369,#32370,#32371,#32372,#32373,#32374,#32375,#32376,#32377,#32378,#32379,
#32380,#32381,#32382,#32383,#32384,#32385,#32386,#32387,#32388,#32389,#32390,
#32391,#32392,#32393,#32394,#32395,#32396,#32397),(#32398,#32399,#32400,
#32401,#32402,#32403,#32404,#32405,#32406,#32407,#32408,#32409,#32410,#32411,
#32412,#32413,#32414,#32415,#32416,#32417,#32418,#32419,#32420,#32421,#32422,
#32423,#32424,#32425,#32426,#32427,#32428,#32429,#32430,#32431,#32432,#32433,
#32434,#32435,#32436,#32437,#32438,#32439,#32440,#32441,#32442,#32443,#32444,
#32445,#32446),(#32447,#32448,#32449,#32450,#32451,#32452,#32453,#32454,
#32455,#32456,#32457,#32458,#32459,#32460,#32461,#32462,#32463,#32464,#32465,
#32466,#32467,#32468,#32469,#32470,#32471,#32472,#32473,#32474,#32475,#32476,
#32477,#32478,#32479,#32480,#32481,#32482,#32483,#32484,#32485,#32486,#32487,
#32488,#32489,#32490,#32491,#32492,#32493,#32494,#32495),(#32496,#32497,
#32498,#32499,#32500,#32501,#32502,#32503,#32504,#32505,#32506,#32507,#32508,
#32509,#32510,#32511,#32512,#32513,#32514,#32515,#32516,#32517,#32518,#32519,
#32520,#32521,#32522,#32523,#32524,#32525,#32526,#32527,#32528,#32529,#32530,
#32531,#32532,#32533,#32534,#32535,#32536,#32537,#32538,#32539,#32540,#32541,
#32542,#32543,#32544),(#32545,#32546,#32547,#32548,#32549,#32550,#32551,
#32552,#32553,#32554,#32555,#32556,#32557,#32558,#32559,#32560,#32561,#32562,
#32563,#32564,#32565,#32566,#32567,#32568,#32569,#32570,#32571,#32572,#32573,
#32574,#32575,#32576,#32577,#32578,#32579,#32580,#32581,#32582,#32583,#32584,
#32585,#32586,#32587,#32588,#32589,#32590,#32591,#32592,#32593),(#32594,
#32595,#32596,#32597,#32598,#32599,#32600,#32601,#32602,#32603,#32604,#32605,
#32606,#32607,#32608,#32609,#32610,#32611,#32612,#32613,#32614,#32615,#32616,
#32617,#32618,#32619,#32620,#32621,#32622,#32623,#32624,#32625,#32626,#32627,
#32628,#32629,#32630,#32631,#32632,#32633,#32634,#32635,#32636,#32637,#32638,
#32639,#32640,#32641,#32642),(#32643,#32644,#32645,#32646,#32647,#32648,
#32649,#32650,#32651,#32652,#32653,#32654,#32655,#32656,#32657,#32658,#32659,
#32660,#32661,#32662,#32663,#32664,#32665,#32666,#32667,#32668,#32669,#32670,
#32671,#32672,#32673,#32674,#32675,#32676,#32677,#32678,#32679,#32680,#32681,
#32682,#32683,#32684,#32685,#32686,#32687,#32688,#32689,#32690,#32691),
(#32692,#32693,#32694,#32695,#32696,#32697,#32698,#32699,#32700,#32701,
#32702,#32703,#32704,#32705,#32706,#32707,#32708,#32709,#32710,#32711,#32712,
#32713,#32714,#32715,#32716,#32717,#32718,#32719,#32720,#32721,#32722,#32723,
#32724,#32725,#32726,#32727,#32728,#32729,#32730,#32731,#32732,#32733,#32734,
#32735,#32736,#32737,#32738,#32739,#32740),(#32741,#32742,#32743,#32744,
#32745,#32746,#32747,#32748,#32749,#32750,#32751,#32752,#32753,#32754,#32755,
#32756,#32757,#32758,#32759,#32760,#32761,#32762,#32763,#32764,#32765,#32766,
#32767,#32768,#32769,#32770,#32771,#32772,#32773,#32774,#32775,#32776,#32777,
#32778,#32779,#32780,#32781,#32782,#32783,#32784,#32785,#32786,#32787,#32788,
#32789),(#32790,#32791,#32792,#32793,#32794,#32795,#32796,#32797,#32798,
#32799,#32800,#32801,#32802,#32803,#32804,#32805,#32806,#32807,#32808,#32809,
#32810,#32811,#32812,#32813,#32814,#32815,#32816,#32817,#32818,#32819,#32820,
#32821,#32822,#32823,#32824,#32825,#32826,#32827,#32828,#32829,#32830,#32831,
#32832,#32833,#32834,#32835,#32836,#32837,#32838),(#32839,#32840,#32841,
#32842,#32843,#32844,#32845,#32846,#32847,#32848,#32849,#32850,#32851,#32852,
#32853,#32854,#32855,#32856,#32857,#32858,#32859,#32860,#32861,#32862,#32863,
#32864,#32865,#32866,#32867,#32868,#32869,#32870,#32871,#32872,#32873,#32874,
#32875,#32876,#32877,#32878,#32879,#32880,#32881,#32882,#32883,#32884,#32885,
#32886,#32887),(#32888,#32889,#32890,#32891,#32892,#32893,#32894,#32895,
#32896,#32897,#32898,#32899,#32900,#32901,#32902,#32903,#32904,#32905,#32906,
#32907,#32908,#32909,#32910,#32911,#32912,#32913,#32914,#32915,#32916,#32917,
#32918,#32919,#32920,#32921,#32922,#32923,#32924,#32925,#32926,#32927,#32928,
#32929,#32930,#32931,#32932,#32933,#32934,#32935,#32936),(#32937,#32938,
#32939,#32940,#32941,#32942,#32943,#32944,#32945,#32946,#32947,#32948,#32949,
#32950,#32951,#32952,#32953,#32954,#32955,#32956,#32957,#32958,#32959,#32960,
#32961,#32962,#32963,#32964,#32965,#32966,#32967,#32968,#32969,#32970,#32971,
#32972,#32973,#32974,#32975,#32976,#32977,#32978,#32979,#32980,#32981,#32982,
#32983,#32984,#32985),(#32986,#32987,#32988,#32989,#32990,#32991,#32992,
#32993,#32994,#32995,#32996,#32997,#32998,#32999,#33000,#33001,#33002,#33003,
#33004,#33005,#33006,#33007,#33008,#33009,#33010,#33011,#33012,#33013,#33014,
#33015,#33016,#33017,#33018,#33019,#33020,#33021,#33022,#33023,#33024,#33025,
#33026,#33027,#33028,#33029,#33030,#33031,#33032,#33033,#33034),(#33035,
#33036,#33037,#33038,#33039,#33040,#33041,#33042,#33043,#33044,#33045,#33046,
#33047,#33048,#33049,#33050,#33051,#33052,#33053,#33054,#33055,#33056,#33057,
#33058,#33059,#33060,#33061,#33062,#33063,#33064,#33065,#33066,#33067,#33068,
#33069,#33070,#33071,#33072,#33073,#33074,#33075,#33076,#33077,#33078,#33079,
#33080,#33081,#33082,#33083),(#33084,#33085,#33086,#33087,#33088,#33089,
#33090,#33091,#33092,#33093,#33094,#33095,#33096,#33097,#33098,#33099,#33100,
#33101,#33102,#33103,#33104,#33105,#33106,#33107,#33108,#33109,#33110,#33111,
#33112,#33113,#33114,#33115,#33116,#33117,#33118,#33119,#33120,#33121,#33122,
#33123,#33124,#33125,#33126,#33127,#33128,#33129,#33130,#33131,#33132),
(#33133,#33134,#33135,#33136,#33137,#33138,#33139,#33140,#33141,#33142,
#33143,#33144,#33145,#33146,#33147,#33148,#33149,#33150,#33151,#33152,#33153,
#33154,#33155,#33156,#33157,#33158,#33159,#33160,#33161,#33162,#33163,#33164,
#33165,#33166,#33167,#33168,#33169,#33170,#33171,#33172,#33173,#33174,#33175,
#33176,#33177,#33178,#33179,#33180,#33181),(#33182,#33183,#33184,#33185,
#33186,#33187,#33188,#33189,#33190,#33191,#33192,#33193,#33194,#33195,#33196,
#33197,#33198,#33199,#33200,#33201,#33202,#33203,#33204,#33205,#33206,#33207,
#33208,#33209,#33210,#33211,#33212,#33213,#33214,#33215,#33216,#33217,#33218,
#33219,#33220,#33221,#33222,#33223,#33224,#33225,#33226,#33227,#33228,#33229,
#33230),(#33231,#33232,#33233,#33234,#33235,#33236,#33237,#33238,#33239,
#33240,#33241,#33242,#33243,#33244,#33245,#33246,#33247,#33248,#33249,#33250,
#33251,#33252,#33253,#33254,#33255,#33256,#33257,#33258,#33259,#33260,#33261,
#33262,#33263,#33264,#33265,#33266,#33267,#33268,#33269,#33270,#33271,#33272,
#33273,#33274,#33275,#33276,#33277,#33278,#33279),(#33280,#33281,#33282,
#33283,#33284,#33285,#33286,#33287,#33288,#33289,#33290,#33291,#33292,#33293,
#33294,#33295,#33296,#33297,#33298,#33299,#33300,#33301,#33302,#33303,#33304,
#33305,#33306,#33307,#33308,#33309,#33310,#33311,#33312,#33313,#33314,#33315,
#33316,#33317,#33318,#33319,#33320,#33321,#33322,#33323,#33324,#33325,#33326,
#33327,#33328),(#33329,#33330,#33331,#33332,#33333,#33334,#33335,#33336,
#33337,#33338,#33339,#33340,#33341,#33342,#33343,#33344,#33345,#33346,#33347,
#33348,#33349,#33350,#33351,#33352,#33353,#33354,#33355,#33356,#33357,#33358,
#33359,#33360,#33361,#33362,#33363,#33364,#33365,#33366,#33367,#33368,#33369,
#33370,#33371,#33372,#33373,#33374,#33375,#33376,#33377),(#33378,#33379,
#33380,#33381,#33382,#33383,#33384,#33385,#33386,#33387,#33388,#33389,#33390,
#33391,#33392,#33393,#33394,#33395,#33396,#33397,#33398,#33399,#33400,#33401,
#33402,#33403,#33404,#33405,#33406,#33407,#33408,#33409,#33410,#33411,#33412,
#33413,#33414,#33415,#33416,#33417,#33418,#33419,#33420,#33421,#33422,#33423,
#33424,#33425,#33426),(#33427,#33428,#33429,#33430,#33431,#33432,#33433,
#33434,#33435,#33436,#33437,#33438,#33439,#33440,#33441,#33442,#33443,#33444,
#33445,#33446,#33447,#33448,#33449,#33450,#33451,#33452,#33453,#33454,#33455,
#33456,#33457,#33458,#33459,#33460,#33461,#33462,#33463,#33464,#33465,#33466,
#33467,#33468,#33469,#33470,#33471,#33472,#33473,#33474,#33475),(#33476,
#33477,#33478,#33479,#33480,#33481,#33482,#33483,#33484,#33485,#33486,#33487,
#33488,#33489,#33490,#33491,#33492,#33493,#33494,#33495,#33496,#33497,#33498,
#33499,#33500,#33501,#33502,#33503,#33504,#33505,#33506,#33507,#33508,#33509,
#33510,#33511,#33512,#33513,#33514,#33515,#33516,#33517,#33518,#33519,#33520,
#33521,#33522,#33523,#33524),(#33525,#33526,#33527,#33528,#33529,#33530,
#33531,#33532,#33533,#33534,#33535,#33536,#33537,#33538,#33539,#33540,#33541,
#33542,#33543,#33544,#33545,#33546,#33547,#33548,#33549,#33550,#33551,#33552,
#33553,#33554,#33555,#33556,#33557,#33558,#33559,#33560,#33561,#33562,#33563,
#33564,#33565,#33566,#33567,#33568,#33569,#33570,#33571,#33572,#33573),
(#33574,#33575,#33576,#33577,#33578,#33579,#33580,#33581,#33582,#33583,
#33584,#33585,#33586,#33587,#33588,#33589,#33590,#33591,#33592,#33593,#33594,
#33595,#33596,#33597,#33598,#33599,#33600,#33601,#33602,#33603,#33604,#33605,
#33606,#33607,#33608,#33609,#33610,#33611,#33612,#33613,#33614,#33615,#33616,
#33617,#33618,#33619,#33620,#33621,#33622),(#33623,#33624,#33625,#33626,
#33627,#33628,#33629,#33630,#33631,#33632,#33633,#33634,#33635,#33636,#33637,
#33638,#33639,#33640,#33641,#33642,#33643,#33644,#33645,#33646,#33647,#33648,
#33649,#33650,#33651,#33652,#33653,#33654,#33655,#33656,#33657,#33658,#33659,
#33660,#33661,#33662,#33663,#33664,#33665,#33666,#33667,#33668,#33669,#33670,
#33671),(#33672,#33673,#33674,#33675,#33676,#33677,#33678,#33679,#33680,
#33681,#33682,#33683,#33684,#33685,#33686,#33687,#33688,#33689,#33690,#33691,
#33692,#33693,#33694,#33695,#33696,#33697,#33698,#33699,#33700,#33701,#33702,
#33703,#33704,#33705,#33706,#33707,#33708,#33709,#33710,#33711,#33712,#33713,
#33714,#33715,#33716,#33717,#33718,#33719,#33720)),.UNSPECIFIED.,.F.,.F.,
 .F.,(4,3,3,3,3,3,3,3,3,3,3,3,3,3,3,3,3,3,3,3,3,3,3,3,3,3,3,3,3,3,3,3,3,
3,3,3,3,3,3,3,4),(4,3,3,3,3,3,3,3,3,3,3,3,3,3,3,3,4),(-1.4142404152185E-5,
-3.89974866163591E-6,-1.33908478899864E-6,-5.87528526800003E-8,1.22157908363864E-6,
6.34290682891319E-6,2.68282178100114E-5,4.73135287911096E-5,6.77988397722078E-5,
8.8284150753306E-5,0.000108769461734404,0.000129254772715502,0.000149740083696601,
0.000190710705658797,0.000231681327620994,0.00027265194958319,0.000313622571545386,
0.000354593193507583,0.000395563815469779,0.000477505059394172,0.000559446303318565,
0.000641387547242958,0.00072332879116735,0.000805270035091743,0.000887211279016136,
0.000969152522940529,0.00113303501078931,0.0012969174986381,0.00146079998648689,
0.00162468247433567,0.00178856496218446,0.00195244745003324,0.00228021242573081,
0.00260797740142839,0.00293574237712596,0.00326350735282353,0.0035912723285211,
0.00391903730421867,0.00424680227991624,0.00457456725561381,0.00528564362278571),
(0.,0.0625,0.125,0.1875,0.25,0.3125,0.375,0.4375,0.5,0.5625,0.625,0.6875,
0.75,0.8125,0.875,0.9375,1.00005554641578),.UNSPECIFIED.);
#194=FACE_BOUND('',#4577,.T.);
#195=FACE_BOUND('',#4579,.T.);
#196=FACE_BOUND('',#4581,.T.);
#197=FACE_BOUND('',#4604,.T.);
#198=FACE_BOUND('',#4623,.T.);
#199=FACE_BOUND('',#4632,.T.);
#200=FACE_BOUND('',#4638,.T.);
#201=FACE_BOUND('',#4639,.T.);
#202=FACE_BOUND('',#4642,.T.);
#203=FACE_BOUND('',#4643,.T.);
#204=FACE_BOUND('',#4645,.T.);
#205=FACE_BOUND('',#4646,.T.);
#206=FACE_BOUND('',#4648,.T.);
#207=FACE_BOUND('',#4652,.T.);
#208=FACE_BOUND('',#4653,.T.);
#209=FACE_BOUND('',#4655,.T.);
#279=PLANE('',#15399);
#280=PLANE('',#15400);
#281=PLANE('',#15401);
#282=PLANE('',#15402);
#283=PLANE('',#15403);
#284=PLANE('',#15404);
#285=PLANE('',#15405);
#286=PLANE('',#15406);
#287=PLANE('',#15407);
#288=PLANE('',#15408);
#289=PLANE('',#15409);
#290=PLANE('',#15410);
#291=PLANE('',#15411);
#292=PLANE('',#15412);
#293=PLANE('',#15413);
#294=PLANE('',#15414);
#295=PLANE('',#15415);
#296=PLANE('',#15416);
#297=PLANE('',#15417);
#298=PLANE('',#15418);
#299=PLANE('',#15419);
#300=PLANE('',#15420);
#301=PLANE('',#15421);
#302=PLANE('',#15422);
#303=PLANE('',#15423);
#304=PLANE('',#15424);
#305=PLANE('',#15425);
#306=PLANE('',#15426);
#307=PLANE('',#15427);
#308=PLANE('',#15428);
#309=PLANE('',#15429);
#310=PLANE('',#15430);
#311=PLANE('',#15431);
#312=PLANE('',#15432);
#313=PLANE('',#15433);
#314=PLANE('',#15434);
#315=PLANE('',#15435);
#316=PLANE('',#15436);
#317=PLANE('',#15437);
#318=PLANE('',#15438);
#319=PLANE('',#15439);
#320=PLANE('',#15440);
#321=PLANE('',#15441);
#322=PLANE('',#15448);
#323=PLANE('',#15452);
#324=PLANE('',#15453);
#325=PLANE('',#15454);
#326=PLANE('',#15455);
#327=PLANE('',#15456);
#328=PLANE('',#15457);
#329=PLANE('',#15458);
#330=PLANE('',#15459);
#331=PLANE('',#15460);
#332=PLANE('',#15461);
#333=PLANE('',#15462);
#334=PLANE('',#15463);
#335=PLANE('',#15464);
#336=PLANE('',#15465);
#337=PLANE('',#15466);
#338=PLANE('',#15467);
#339=PLANE('',#15468);
#340=PLANE('',#15469);
#341=PLANE('',#15470);
#735=ELLIPSE('',#15361,7.42462120254335,5.25000000010882);
#736=ELLIPSE('',#15365,7.42462120245347,5.24999999999376);
#737=ELLIPSE('',#15371,7.42470893119486,5.25007996454306);
#738=ELLIPSE('',#15372,7.42470893118818,5.25007996453788);
#795=B_SPLINE_CURVE_WITH_KNOTS('',3,(#21423,#21424,#21425,#21426,#21427,
#21428,#21429,#21430,#21431,#21432,#21433,#21434,#21435,#21436,#21437,#21438,
#21439,#21440,#21441,#21442,#21443,#21444),.UNSPECIFIED.,.F.,.F.,(4,2,2,
2,2,2,2,2,2,2,4),(-3.36585159579603,-3.23154274939443,-3.10218229476243,
-2.97282184013043,-2.86647922856163,-2.76013661699283,-2.65379400542402,
-2.54745139385522,-2.41809093922322,-2.28873048459122,-2.15442163818962),
 .UNSPECIFIED.);
#796=B_SPLINE_CURVE_WITH_KNOTS('',3,(#27646,#27647,#27648,#27649,#27650,
#27651,#27652,#27653,#27654,#27655,#27656,#27657,#27658,#27659,#27660,#27661,
#27662,#27663,#27664,#27665,#27666,#27667,#27668,#27669,#27670,#27671,#27672,
#27673,#27674,#27675,#27676,#27677,#27678,#27679,#27680,#27681,#27682,#27683,
#27684,#27685,#27686,#27687,#27688,#27689,#27690,#27691,#27692,#27693,#27694,
#27695,#27696,#27697,#27698,#27699,#27700,#27701,#27702,#27703,#27704,#27705,
#27706,#27707,#27708,#27709,#27710,#27711,#27712,#27713,#27714,#27715,#27716,
#27717,#27718,#27719,#27720,#27721,#27722,#27723,#27724,#27725,#27726,#27727,
#27728,#27729,#27730,#27731,#27732,#27733,#27734,#27735,#27736,#27737,#27738,
#27739,#27740,#27741,#27742,#27743,#27744,#27745,#27746,#27747,#27748,#27749,
#27750,#27751,#27752,#27753,#27754,#27755,#27756,#27757,#27758,#27759,#27760,
#27761,#27762,#27763,#27764,#27765,#27766),.UNSPECIFIED.,.F.,.F.,(4,3,3,
3,3,3,3,3,3,3,3,3,3,3,3,3,3,3,3,3,3,3,3,3,3,3,3,3,3,3,3,3,3,3,3,3,3,3,3,
3,4),(-0.00524423961119122,-0.00523399695570063,-0.00523143629190568,-0.00523015596002173,
-0.00522887562795533,-0.00522375430021003,-0.00520326898922881,-0.00518278367839879,
-0.00516229836726638,-0.00514181305643454,-0.00512132774545271,-0.00510084243447086,
-0.00508035712334152,-0.00503938650152429,-0.00499841587941665,-0.00495744525759613,
-0.00491647463549179,-0.00487550401366842,-0.00483453339170461,-0.00475259214764206,
-0.00467065090384962,-0.00458870965979234,-0.00450676841599483,-0.00442482717194261,
-0.00434288592814021,-0.00426094468409288,-0.00409706219635843,-0.00393317970839343,
-0.00376929722064964,-0.00360541473269398,-0.00344153224494097,-0.00327764975699452,
-0.00294988478137813,-0.00262211980559562,-0.0022943548299611,-0.00196658985425258,
-0.00163882487854402,-0.00131105990279781,-0.000983294927126725,-0.000655529951398905,
0.),.UNSPECIFIED.);
#797=B_SPLINE_CURVE_WITH_KNOTS('',3,(#33721,#33722,#33723,#33724,#33725,
#33726,#33727,#33728,#33729,#33730,#33731,#33732,#33733,#33734,#33735,#33736,
#33737,#33738,#33739,#33740,#33741,#33742,#33743,#33744,#33745,#33746,#33747,
#33748,#33749,#33750,#33751,#33752,#33753,#33754,#33755,#33756,#33757,#33758,
#33759,#33760,#33761,#33762,#33763,#33764,#33765,#33766,#33767,#33768,#33769,
#33770,#33771,#33772,#33773,#33774,#33775,#33776,#33777,#33778,#33779,#33780,
#33781,#33782,#33783,#33784,#33785,#33786,#33787,#33788,#33789,#33790,#33791,
#33792,#33793,#33794,#33795,#33796,#33797,#33798,#33799,#33800,#33801,#33802,
#33803,#33804,#33805,#33806,#33807,#33808,#33809,#33810,#33811,#33812,#33813,
#33814,#33815,#33816,#33817,#33818,#33819,#33820,#33821,#33822,#33823,#33824,
#33825,#33826,#33827,#33828,#33829,#33830,#33831,#33832,#33833,#33834,#33835,
#33836,#33837,#33838,#33839,#33840,#33841),.UNSPECIFIED.,.F.,.F.,(4,3,3,
3,3,3,3,3,3,3,3,3,3,3,3,3,3,3,3,3,3,3,3,3,3,3,3,3,3,3,3,3,3,3,3,3,3,3,3,
3,4),(0.,0.000655529951398911,0.000983294927092821,0.00131105990279782,
0.00163882487848811,0.0019665898541858,0.00229435482988349,0.00262211980559564,
0.00294988478127885,0.00327764975699456,0.00344153224482537,0.00360541473269401,
0.00376929722052302,0.00393317970839347,0.00409706219622063,0.00426094468409292,
0.00434288592799383,0.00442482717194265,0.0045067684158426,0.00458870965979238,
0.00467065090369136,0.00475259214764211,0.00483453339154007,0.00487550401350222,
0.00491647463549184,0.00495744525742651,0.0049984158794167,0.00503938650135109,
0.00508035712334157,0.00510084243429463,0.00512132774527543,0.00514181305625618,
0.00516229836726643,0.00518278367821808,0.00520326898922886,0.00522375430021008,
0.00522887562795538,0.00523015595986631,0.00523143629181281,0.00523399695570069,
0.0052442396111913),.UNSPECIFIED.);
#1032=CONICAL_SURFACE('',#15353,7.5,0.221314442347791);
#1033=CONICAL_SURFACE('',#15376,5.04017795657138,0.606317781856836);
#1034=CONICAL_SURFACE('',#15394,4.2,0.785398163397447);
#1057=LINE('',#21397,#2250);
#1058=LINE('',#21402,#2251);
#1059=LINE('',#21407,#2252);
#1060=LINE('',#21413,#2253);
#1061=LINE('',#21419,#2254);
#1062=LINE('',#21451,#2255);
#1063=LINE('',#21454,#2256);
#1064=LINE('',#21469,#2257);
#1065=LINE('',#21475,#2258);
#1066=LINE('',#21482,#2259);
#1067=LINE('',#21486,#2260);
#1068=LINE('',#21492,#2261);
#1069=LINE('',#21498,#2262);
#1070=LINE('',#21504,#2263);
#1071=LINE('',#21516,#2264);
#1072=LINE('',#21521,#2265);
#1073=LINE('',#21526,#2266);
#1074=LINE('',#21536,#2267);
#1075=LINE('',#21538,#2268);
#1076=LINE('',#21540,#2269);
#1077=LINE('',#21541,#2270);
#1078=LINE('',#21545,#2271);
#1079=LINE('',#21546,#2272);
#1080=LINE('',#21547,#2273);
#1081=LINE('',#21550,#2274);
#1082=LINE('',#21551,#2275);
#1083=LINE('',#21554,#2276);
#1084=LINE('',#21555,#2277);
#1085=LINE('',#21559,#2278);
#1086=LINE('',#21561,#2279);
#1087=LINE('',#21563,#2280);
#1088=LINE('',#21564,#2281);
#1089=LINE('',#21568,#2282);
#1090=LINE('',#21570,#2283);
#1091=LINE('',#21571,#2284);
#1092=LINE('',#21572,#2285);
#1093=LINE('',#21575,#2286);
#1094=LINE('',#21576,#2287);
#1095=LINE('',#21580,#2288);
#1096=LINE('',#21582,#2289);
#1097=LINE('',#21584,#2290);
#1098=LINE('',#21585,#2291);
#1099=LINE('',#21589,#2292);
#1100=LINE('',#21590,#2293);
#1101=LINE('',#21591,#2294);
#1102=LINE('',#21595,#2295);
#1103=LINE('',#21596,#2296);
#1104=LINE('',#21597,#2297);
#1105=LINE('',#21600,#2298);
#1106=LINE('',#21602,#2299);
#1107=LINE('',#21603,#2300);
#1108=LINE('',#21606,#2301);
#1109=LINE('',#21607,#2302);
#1110=LINE('',#21609,#2303);
#1111=LINE('',#21610,#2304);
#1112=LINE('',#21613,#2305);
#1113=LINE('',#21615,#2306);
#1114=LINE('',#21616,#2307);
#1115=LINE('',#21617,#2308);
#1116=LINE('',#21619,#2309);
#1117=LINE('',#21623,#2310);
#1118=LINE('',#21624,#2311);
#1119=LINE('',#21625,#2312);
#1120=LINE('',#21628,#2313);
#1121=LINE('',#21629,#2314);
#1122=LINE('',#21632,#2315);
#1123=LINE('',#21633,#2316);
#1124=LINE('',#21635,#2317);
#1125=LINE('',#21640,#2318);
#1126=LINE('',#21642,#2319);
#1127=LINE('',#21644,#2320);
#1128=LINE('',#21645,#2321);
#1129=LINE('',#21649,#2322);
#1130=LINE('',#21651,#2323);
#1131=LINE('',#21653,#2324);
#1132=LINE('',#21654,#2325);
#1133=LINE('',#21657,#2326);
#1134=LINE('',#21659,#2327);
#1135=LINE('',#21661,#2328);
#1136=LINE('',#21663,#2329);
#1137=LINE('',#21664,#2330);
#1138=LINE('',#21666,#2331);
#1139=LINE('',#21669,#2332);
#1140=LINE('',#21671,#2333);
#1141=LINE('',#21672,#2334);
#1142=LINE('',#21675,#2335);
#1143=LINE('',#21677,#2336);
#1144=LINE('',#21678,#2337);
#1145=LINE('',#21681,#2338);
#1146=LINE('',#21682,#2339);
#1147=LINE('',#21683,#2340);
#1148=LINE('',#21685,#2341);
#1149=LINE('',#21687,#2342);
#1150=LINE('',#21688,#2343);
#1151=LINE('',#21691,#2344);
#1152=LINE('',#21692,#2345);
#1153=LINE('',#21694,#2346);
#1154=LINE('',#21695,#2347);
#1155=LINE('',#21697,#2348);
#1156=LINE('',#21700,#2349);
#1157=LINE('',#21702,#2350);
#1158=LINE('',#21703,#2351);
#1159=LINE('',#21705,#2352);
#1160=LINE('',#21706,#2353);
#1161=LINE('',#21708,#2354);
#1162=LINE('',#21709,#2355);
#1163=LINE('',#21711,#2356);
#1164=LINE('',#21713,#2357);
#1165=LINE('',#33847,#2358);
#1166=LINE('',#33850,#2359);
#1167=LINE('',#33853,#2360);
#1168=LINE('',#33855,#2361);
#1169=LINE('',#33856,#2362);
#1170=LINE('',#33862,#2363);
#1171=LINE('',#33867,#2364);
#1172=LINE('',#33869,#2365);
#1173=LINE('',#33871,#2366);
#1174=LINE('',#33872,#2367);
#1175=LINE('',#33874,#2368);
#1176=LINE('',#33875,#2369);
#1177=LINE('',#33877,#2370);
#1178=LINE('',#33878,#2371);
#1179=LINE('',#33881,#2372);
#1180=LINE('',#33882,#2373);
#1181=LINE('',#33891,#2374);
#1182=LINE('',#33893,#2375);
#1183=LINE('',#33895,#2376);
#1184=LINE('',#33896,#2377);
#1185=LINE('',#33899,#2378);
#1186=LINE('',#33901,#2379);
#1187=LINE('',#33902,#2380);
#1188=LINE('',#33905,#2381);
#1189=LINE('',#33906,#2382);
#1190=LINE('',#33910,#2383);
#1191=LINE('',#33911,#2384);
#1192=LINE('',#33913,#2385);
#2250=VECTOR('',#16970,6.25);
#2251=VECTOR('',#16977,6.25);
#2252=VECTOR('',#16982,2.25);
#2253=VECTOR('',#16989,3.);
#2254=VECTOR('',#16996,7.5);
#2255=VECTOR('',#17005,1000.);
#2256=VECTOR('',#17008,1000.);
#2257=VECTOR('',#17025,4.);
#2258=VECTOR('',#17032,5.25);
#2259=VECTOR('',#17041,5.04017795657138);
#2260=VECTOR('',#17046,5.04017795657138);
#2261=VECTOR('',#17053,0.300000000000003);
#2262=VECTOR('',#17060,0.300000000000003);
#2263=VECTOR('',#17067,4.);
#2264=VECTOR('',#17082,4.2);
#2265=VECTOR('',#17089,4.2);
#2266=VECTOR('',#17094,5.8);
#2267=VECTOR('',#17109,1000.);
#2268=VECTOR('',#17110,1000.);
#2269=VECTOR('',#17111,1000.);
#2270=VECTOR('',#17112,1000.);
#2271=VECTOR('',#17115,1000.);
#2272=VECTOR('',#17116,1000.);
#2273=VECTOR('',#17117,1000.);
#2274=VECTOR('',#17120,1000.);
#2275=VECTOR('',#17121,1000.);
#2276=VECTOR('',#17124,1000.);
#2277=VECTOR('',#17125,1000.);
#2278=VECTOR('',#17128,1000.);
#2279=VECTOR('',#17129,1000.);
#2280=VECTOR('',#17130,1000.);
#2281=VECTOR('',#17131,1000.);
#2282=VECTOR('',#17134,1000.);
#2283=VECTOR('',#17135,1000.);
#2284=VECTOR('',#17136,1000.);
#2285=VECTOR('',#17137,1000.);
#2286=VECTOR('',#17140,1000.);
#2287=VECTOR('',#17141,1000.);
#2288=VECTOR('',#17144,1000.);
#2289=VECTOR('',#17145,1000.);
#2290=VECTOR('',#17146,1000.);
#2291=VECTOR('',#17147,1000.);
#2292=VECTOR('',#17150,1000.);
#2293=VECTOR('',#17151,1000.);
#2294=VECTOR('',#17152,1000.);
#2295=VECTOR('',#17155,1000.);
#2296=VECTOR('',#17156,1000.);
#2297=VECTOR('',#17157,1000.);
#2298=VECTOR('',#17160,1000.);
#2299=VECTOR('',#17161,1000.);
#2300=VECTOR('',#17162,1000.);
#2301=VECTOR('',#17165,1000.);
#2302=VECTOR('',#17166,1000.);
#2303=VECTOR('',#17169,1000.);
#2304=VECTOR('',#17170,1000.);
#2305=VECTOR('',#17173,1000.);
#2306=VECTOR('',#17174,1000.);
#2307=VECTOR('',#17175,1000.);
#2308=VECTOR('',#17176,1000.);
#2309=VECTOR('',#17179,1000.);
#2310=VECTOR('',#17182,1000.);
#2311=VECTOR('',#17183,1000.);
#2312=VECTOR('',#17184,1000.);
#2313=VECTOR('',#17187,1000.);
#2314=VECTOR('',#17188,1000.);
#2315=VECTOR('',#17191,1000.);
#2316=VECTOR('',#17192,1000.);
#2317=VECTOR('',#17195,1000.);
#2318=VECTOR('',#17200,1000.);
#2319=VECTOR('',#17201,1000.);
#2320=VECTOR('',#17202,1000.);
#2321=VECTOR('',#17203,1000.);
#2322=VECTOR('',#17206,1000.);
#2323=VECTOR('',#17207,1000.);
#2324=VECTOR('',#17208,1000.);
#2325=VECTOR('',#17209,1000.);
#2326=VECTOR('',#17212,1000.);
#2327=VECTOR('',#17213,1000.);
#2328=VECTOR('',#17214,1000.);
#2329=VECTOR('',#17215,1000.);
#2330=VECTOR('',#17216,1000.);
#2331=VECTOR('',#17219,1000.);
#2332=VECTOR('',#17222,1000.);
#2333=VECTOR('',#17223,1000.);
#2334=VECTOR('',#17224,1000.);
#2335=VECTOR('',#17227,1000.);
#2336=VECTOR('',#17228,1000.);
#2337=VECTOR('',#17229,1000.);
#2338=VECTOR('',#17232,1000.);
#2339=VECTOR('',#17233,1000.);
#2340=VECTOR('',#17234,1000.);
#2341=VECTOR('',#17237,1000.);
#2342=VECTOR('',#17238,1000.);
#2343=VECTOR('',#17239,1000.);
#2344=VECTOR('',#17242,1000.);
#2345=VECTOR('',#17243,1000.);
#2346=VECTOR('',#17246,1000.);
#2347=VECTOR('',#17247,1000.);
#2348=VECTOR('',#17250,1000.);
#2349=VECTOR('',#17253,1000.);
#2350=VECTOR('',#17254,1000.);
#2351=VECTOR('',#17255,1000.);
#2352=VECTOR('',#17258,1000.);
#2353=VECTOR('',#17259,1000.);
#2354=VECTOR('',#17262,1000.);
#2355=VECTOR('',#17263,1000.);
#2356=VECTOR('',#17266,1000.);
#2357=VECTOR('',#17269,1000.);
#2358=VECTOR('',#17284,1000.);
#2359=VECTOR('',#17287,1000.);
#2360=VECTOR('',#17290,1000.);
#2361=VECTOR('',#17291,1000.);
#2362=VECTOR('',#17292,1000.);
#2363=VECTOR('',#17299,1000.);
#2364=VECTOR('',#17304,1000.);
#2365=VECTOR('',#17305,1000.);
#2366=VECTOR('',#17306,1000.);
#2367=VECTOR('',#17307,1000.);
#2368=VECTOR('',#17310,1000.);
#2369=VECTOR('',#17311,1000.);
#2370=VECTOR('',#17314,1000.);
#2371=VECTOR('',#17315,1000.);
#2372=VECTOR('',#17320,1000.);
#2373=VECTOR('',#17321,1000.);
#2374=VECTOR('',#17334,1000.);
#2375=VECTOR('',#17335,1000.);
#2376=VECTOR('',#17336,1000.);
#2377=VECTOR('',#17337,1000.);
#2378=VECTOR('',#17340,1000.);
#2379=VECTOR('',#17341,1000.);
#2380=VECTOR('',#17342,1000.);
#2381=VECTOR('',#17345,1000.);
#2382=VECTOR('',#17346,1000.);
#2383=VECTOR('',#17351,1000.);
#2384=VECTOR('',#17352,1000.);
#2385=VECTOR('',#17355,1000.);
#3443=CYLINDRICAL_SURFACE('',#15343,6.25);
#3444=CYLINDRICAL_SURFACE('',#15345,6.25);
#3445=CYLINDRICAL_SURFACE('',#15347,2.25);
#3446=CYLINDRICAL_SURFACE('',#15350,3.);
#3447=CYLINDRICAL_SURFACE('',#15357,10.0000000011845);
#3448=CYLINDRICAL_SURFACE('',#15360,5.25);
#3449=CYLINDRICAL_SURFACE('',#15366,4.);
#3450=CYLINDRICAL_SURFACE('',#15369,5.25);
#3451=CYLINDRICAL_SURFACE('',#15373,5.04017795657138);
#3452=CYLINDRICAL_SURFACE('',#15378,0.300000000000003);
#3453=CYLINDRICAL_SURFACE('',#15381,0.300000000000003);
#3454=CYLINDRICAL_SURFACE('',#15384,4.);
#3455=CYLINDRICAL_SURFACE('',#15391,4.2);
#3456=CYLINDRICAL_SURFACE('',#15396,5.8);
#3457=CYLINDRICAL_SURFACE('',#15445,5.);
#3458=CYLINDRICAL_SURFACE('',#15449,10.0000000011845);
#3690=FACE_OUTER_BOUND('',#4557,.T.);
#3691=FACE_OUTER_BOUND('',#4558,.T.);
#3692=FACE_OUTER_BOUND('',#4559,.T.);
#3693=FACE_OUTER_BOUND('',#4560,.T.);
#3694=FACE_OUTER_BOUND('',#4561,.T.);
#3695=FACE_OUTER_BOUND('',#4562,.T.);
#3696=FACE_OUTER_BOUND('',#4563,.T.);
#3697=FACE_OUTER_BOUND('',#4564,.T.);
#3698=FACE_OUTER_BOUND('',#4565,.T.);
#3699=FACE_OUTER_BOUND('',#4566,.T.);
#3700=FACE_OUTER_BOUND('',#4567,.T.);
#3701=FACE_OUTER_BOUND('',#4568,.T.);
#3702=FACE_OUTER_BOUND('',#4569,.T.);
#3703=FACE_OUTER_BOUND('',#4570,.T.);
#3704=FACE_OUTER_BOUND('',#4571,.T.);
#3705=FACE_OUTER_BOUND('',#4572,.T.);
#3706=FACE_OUTER_BOUND('',#4573,.T.);
#3707=FACE_OUTER_BOUND('',#4574,.T.);
#3708=FACE_OUTER_BOUND('',#4575,.T.);
#3709=FACE_OUTER_BOUND('',#4576,.T.);
#3710=FACE_OUTER_BOUND('',#4578,.T.);
#3711=FACE_OUTER_BOUND('',#4580,.T.);
#3712=FACE_OUTER_BOUND('',#4582,.T.);
#3713=FACE_OUTER_BOUND('',#4583,.T.);
#3714=FACE_OUTER_BOUND('',#4584,.T.);
#3715=FACE_OUTER_BOUND('',#4585,.T.);
#3716=FACE_OUTER_BOUND('',#4586,.T.);
#3717=FACE_OUTER_BOUND('',#4587,.T.);
#3718=FACE_OUTER_BOUND('',#4588,.T.);
#3719=FACE_OUTER_BOUND('',#4589,.T.);
#3720=FACE_OUTER_BOUND('',#4590,.T.);
#3721=FACE_OUTER_BOUND('',#4591,.T.);
#3722=FACE_OUTER_BOUND('',#4592,.T.);
#3723=FACE_OUTER_BOUND('',#4593,.T.);
#3724=FACE_OUTER_BOUND('',#4594,.T.);
#3725=FACE_OUTER_BOUND('',#4595,.T.);
#3726=FACE_OUTER_BOUND('',#4596,.T.);
#3727=FACE_OUTER_BOUND('',#4597,.T.);
#3728=FACE_OUTER_BOUND('',#4598,.T.);
#3729=FACE_OUTER_BOUND('',#4599,.T.);
#3730=FACE_OUTER_BOUND('',#4600,.T.);
#3731=FACE_OUTER_BOUND('',#4601,.T.);
#3732=FACE_OUTER_BOUND('',#4602,.T.);
#3733=FACE_OUTER_BOUND('',#4603,.T.);
#3734=FACE_OUTER_BOUND('',#4605,.T.);
#3735=FACE_OUTER_BOUND('',#4606,.T.);
#3736=FACE_OUTER_BOUND('',#4607,.T.);
#3737=FACE_OUTER_BOUND('',#4608,.T.);
#3738=FACE_OUTER_BOUND('',#4609,.T.);
#3739=FACE_OUTER_BOUND('',#4610,.T.);
#3740=FACE_OUTER_BOUND('',#4611,.T.);
#3741=FACE_OUTER_BOUND('',#4612,.T.);
#3742=FACE_OUTER_BOUND('',#4613,.T.);
#3743=FACE_OUTER_BOUND('',#4614,.T.);
#3744=FACE_OUTER_BOUND('',#4615,.T.);
#3745=FACE_OUTER_BOUND('',#4616,.T.);
#3746=FACE_OUTER_BOUND('',#4617,.T.);
#3747=FACE_OUTER_BOUND('',#4618,.T.);
#3748=FACE_OUTER_BOUND('',#4619,.T.);
#3749=FACE_OUTER_BOUND('',#4620,.T.);
#3750=FACE_OUTER_BOUND('',#4621,.T.);
#3751=FACE_OUTER_BOUND('',#4622,.T.);
#3752=FACE_OUTER_BOUND('',#4624,.T.);
#3753=FACE_OUTER_BOUND('',#4625,.T.);
#3754=FACE_OUTER_BOUND('',#4626,.T.);
#3755=FACE_OUTER_BOUND('',#4627,.T.);
#3756=FACE_OUTER_BOUND('',#4628,.T.);
#3757=FACE_OUTER_BOUND('',#4629,.T.);
#3758=FACE_OUTER_BOUND('',#4630,.T.);
#3759=FACE_OUTER_BOUND('',#4631,.T.);
#3760=FACE_OUTER_BOUND('',#4633,.T.);
#3761=FACE_OUTER_BOUND('',#4634,.T.);
#3762=FACE_OUTER_BOUND('',#4635,.T.);
#3763=FACE_OUTER_BOUND('',#4636,.T.);
#3764=FACE_OUTER_BOUND('',#4637,.T.);
#3765=FACE_OUTER_BOUND('',#4640,.T.);
#3766=FACE_OUTER_BOUND('',#4641,.T.);
#3767=FACE_OUTER_BOUND('',#4644,.T.);
#3768=FACE_OUTER_BOUND('',#4647,.T.);
#3769=FACE_OUTER_BOUND('',#4649,.T.);
#3770=FACE_OUTER_BOUND('',#4650,.T.);
#3771=FACE_OUTER_BOUND('',#4651,.T.);
#3772=FACE_OUTER_BOUND('',#4654,.T.);
#3773=FACE_OUTER_BOUND('',#4656,.T.);
#3774=FACE_OUTER_BOUND('',#4657,.T.);
#3775=FACE_OUTER_BOUND('',#4658,.T.);
#3776=FACE_OUTER_BOUND('',#4659,.T.);
#4557=EDGE_LOOP('',(#9833,#9834,#9835,#9836));
#4558=EDGE_LOOP('',(#9837,#9838,#9839,#9840));
#4559=EDGE_LOOP('',(#9841,#9842,#9843,#9844));
#4560=EDGE_LOOP('',(#9845,#9846,#9847,#9848));
#4561=EDGE_LOOP('',(#9849,#9850,#9851,#9852));
#4562=EDGE_LOOP('',(#9853,#9854,#9855,#9856,#9857,#9858));
#4563=EDGE_LOOP('',(#9859,#9860,#9861,#9862));
#4564=EDGE_LOOP('',(#9863,#9864,#9865,#9866,#9867,#9868,#9869));
#4565=EDGE_LOOP('',(#9870,#9871,#9872,#9873));
#4566=EDGE_LOOP('',(#9874,#9875,#9876,#9877,#9878,#9879,#9880,#9881,#9882,
#9883));
#4567=EDGE_LOOP('',(#9884,#9885,#9886,#9887));
#4568=EDGE_LOOP('',(#9888,#9889,#9890,#9891));
#4569=EDGE_LOOP('',(#9892,#9893,#9894,#9895));
#4570=EDGE_LOOP('',(#9896,#9897,#9898,#9899));
#4571=EDGE_LOOP('',(#9900,#9901,#9902,#9903));
#4572=EDGE_LOOP('',(#9904,#9905,#9906,#9907));
#4573=EDGE_LOOP('',(#9908,#9909,#9910,#9911));
#4574=EDGE_LOOP('',(#9912,#9913,#9914,#9915));
#4575=EDGE_LOOP('',(#9916,#9917,#9918,#9919));
#4576=EDGE_LOOP('',(#9920));
#4577=EDGE_LOOP('',(#9921));
#4578=EDGE_LOOP('',(#9922));
#4579=EDGE_LOOP('',(#9923));
#4580=EDGE_LOOP('',(#9924));
#4581=EDGE_LOOP('',(#9925));
#4582=EDGE_LOOP('',(#9926));
#4583=EDGE_LOOP('',(#9927));
#4584=EDGE_LOOP('',(#9928,#9929,#9930,#9931));
#4585=EDGE_LOOP('',(#9932,#9933,#9934,#9935));
#4586=EDGE_LOOP('',(#9936,#9937,#9938,#9939));
#4587=EDGE_LOOP('',(#9940,#9941,#9942,#9943));
#4588=EDGE_LOOP('',(#9944,#9945,#9946,#9947));
#4589=EDGE_LOOP('',(#9948,#9949,#9950,#9951,#9952));
#4590=EDGE_LOOP('',(#9953,#9954,#9955,#9956));
#4591=EDGE_LOOP('',(#9957,#9958,#9959,#9960));
#4592=EDGE_LOOP('',(#9961,#9962,#9963,#9964));
#4593=EDGE_LOOP('',(#9965,#9966,#9967,#9968));
#4594=EDGE_LOOP('',(#9969,#9970,#9971,#9972));
#4595=EDGE_LOOP('',(#9973,#9974,#9975,#9976));
#4596=EDGE_LOOP('',(#9977,#9978,#9979,#9980));
#4597=EDGE_LOOP('',(#9981,#9982,#9983,#9984,#9985,#9986));
#4598=EDGE_LOOP('',(#9987,#9988,#9989,#9990));
#4599=EDGE_LOOP('',(#9991,#9992,#9993,#9994));
#4600=EDGE_LOOP('',(#9995,#9996,#9997,#9998));
#4601=EDGE_LOOP('',(#9999,#10000,#10001,#10002));
#4602=EDGE_LOOP('',(#10003,#10004,#10005,#10006));
#4603=EDGE_LOOP('',(#10007));
#4604=EDGE_LOOP('',(#10008));
#4605=EDGE_LOOP('',(#10009,#10010,#10011,#10012));
#4606=EDGE_LOOP('',(#10013,#10014,#10015,#10016));
#4607=EDGE_LOOP('',(#10017,#10018,#10019,#10020,#10021,#10022));
#4608=EDGE_LOOP('',(#10023,#10024,#10025,#10026));
#4609=EDGE_LOOP('',(#10027,#10028,#10029,#10030));
#4610=EDGE_LOOP('',(#10031,#10032,#10033,#10034));
#4611=EDGE_LOOP('',(#10035,#10036,#10037,#10038,#10039,#10040));
#4612=EDGE_LOOP('',(#10041,#10042,#10043,#10044,#10045,#10046));
#4613=EDGE_LOOP('',(#10047,#10048,#10049,#10050));
#4614=EDGE_LOOP('',(#10051,#10052,#10053,#10054,#10055,#10056));
#4615=EDGE_LOOP('',(#10057,#10058,#10059,#10060));
#4616=EDGE_LOOP('',(#10061,#10062,#10063,#10064));
#4617=EDGE_LOOP('',(#10065,#10066,#10067,#10068));
#4618=EDGE_LOOP('',(#10069,#10070,#10071,#10072,#10073,#10074,#10075,#10076));
#4619=EDGE_LOOP('',(#10077,#10078,#10079,#10080,#10081,#10082));
#4620=EDGE_LOOP('',(#10083,#10084,#10085,#10086,#10087));
#4621=EDGE_LOOP('',(#10088,#10089,#10090,#10091));
#4622=EDGE_LOOP('',(#10092));
#4623=EDGE_LOOP('',(#10093));
#4624=EDGE_LOOP('',(#10094,#10095,#10096));
#4625=EDGE_LOOP('',(#10097,#10098,#10099,#10100));
#4626=EDGE_LOOP('',(#10101,#10102,#10103));
#4627=EDGE_LOOP('',(#10104,#10105,#10106,#10107));
#4628=EDGE_LOOP('',(#10108,#10109,#10110,#10111));
#4629=EDGE_LOOP('',(#10112,#10113,#10114,#10115));
#4630=EDGE_LOOP('',(#10116,#10117,#10118,#10119));
#4631=EDGE_LOOP('',(#10120,#10121,#10122,#10123));
#4632=EDGE_LOOP('',(#10124,#10125,#10126,#10127));
#4633=EDGE_LOOP('',(#10128,#10129,#10130,#10131));
#4634=EDGE_LOOP('',(#10132,#10133,#10134,#10135));
#4635=EDGE_LOOP('',(#10136,#10137,#10138));
#4636=EDGE_LOOP('',(#10139,#10140,#10141,#10142));
#4637=EDGE_LOOP('',(#10143,#10144,#10145,#10146,#10147,#10148,#10149,#10150));
#4638=EDGE_LOOP('',(#10151));
#4639=EDGE_LOOP('',(#10152));
#4640=EDGE_LOOP('',(#10153));
#4641=EDGE_LOOP('',(#10154));
#4642=EDGE_LOOP('',(#10155));
#4643=EDGE_LOOP('',(#10156));
#4644=EDGE_LOOP('',(#10157,#10158,#10159,#10160,#10161,#10162,#10163,#10164));
#4645=EDGE_LOOP('',(#10165));
#4646=EDGE_LOOP('',(#10166));
#4647=EDGE_LOOP('',(#10167));
#4648=EDGE_LOOP('',(#10168));
#4649=EDGE_LOOP('',(#10169,#10170,#10171,#10172));
#4650=EDGE_LOOP('',(#10173,#10174,#10175,#10176));
#4651=EDGE_LOOP('',(#10177,#10178,#10179,#10180));
#4652=EDGE_LOOP('',(#10181,#10182,#10183,#10184));
#4653=EDGE_LOOP('',(#10185,#10186,#10187,#10188));
#4654=EDGE_LOOP('',(#10189));
#4655=EDGE_LOOP('',(#10190));
#4656=EDGE_LOOP('',(#10191,#10192,#10193,#10194));
#4657=EDGE_LOOP('',(#10195,#10196,#10197,#10198));
#4658=EDGE_LOOP('',(#10199,#10200,#10201,#10202));
#4659=EDGE_LOOP('',(#10203,#10204,#10205,#10206));
#5509=CIRCLE('',#15340,6.25);
#5510=CIRCLE('',#15341,1.);
#5511=CIRCLE('',#15342,6.25);
#5512=CIRCLE('',#15344,6.25);
#5513=CIRCLE('',#15346,6.25);
#5514=CIRCLE('',#15348,2.25);
#5515=CIRCLE('',#15349,2.25);
#5516=CIRCLE('',#15351,3.);
#5517=CIRCLE('',#15352,3.);
#5518=CIRCLE('',#15354,7.5);
#5519=CIRCLE('',#15355,5.25);
#5520=CIRCLE('',#15356,5.25);
#5521=CIRCLE('',#15358,10.0000000011845);
#5522=CIRCLE('',#15359,10.0000000011845);
#5523=CIRCLE('',#15362,10.4947894497429);
#5524=CIRCLE('',#15363,5.25);
#5525=CIRCLE('',#15364,10.4947894499283);
#5526=CIRCLE('',#15367,4.);
#5527=CIRCLE('',#15368,4.);
#5528=CIRCLE('',#15370,5.25);
#5529=CIRCLE('',#15374,5.04017795657138);
#5530=CIRCLE('',#15375,5.04017795657138);
#5531=CIRCLE('',#15377,4.);
#5532=CIRCLE('',#15379,0.300000000000003);
#5533=CIRCLE('',#15380,0.300000000000003);
#5534=CIRCLE('',#15382,0.300000000000003);
#5535=CIRCLE('',#15383,0.300000000000003);
#5536=CIRCLE('',#15385,4.);
#5537=CIRCLE('',#15386,4.);
#5538=CIRCLE('',#15388,4.5);
#5539=CIRCLE('',#15389,0.75);
#5540=CIRCLE('',#15390,4.5);
#5541=CIRCLE('',#15392,4.19999999999999);
#5542=CIRCLE('',#15393,4.2);
#5543=CIRCLE('',#15395,4.5);
#5544=CIRCLE('',#15397,5.8);
#5545=CIRCLE('',#15398,5.8);
#5546=CIRCLE('',#15442,5.);
#5547=CIRCLE('',#15443,5.);
#5548=CIRCLE('',#15444,0.249999999999999);
#5549=CIRCLE('',#15446,5.);
#5550=CIRCLE('',#15447,5.);
#5551=CIRCLE('',#15450,10.0000000011845);
#5552=CIRCLE('',#15451,10.0000000011845);
#6221=VERTEX_POINT('',#21390);
#6222=VERTEX_POINT('',#21392);
#6223=VERTEX_POINT('',#21396);
#6224=VERTEX_POINT('',#21400);
#6225=VERTEX_POINT('',#21404);
#6226=VERTEX_POINT('',#21406);
#6227=VERTEX_POINT('',#21410);
#6228=VERTEX_POINT('',#21412);
#6229=VERTEX_POINT('',#21416);
#6230=VERTEX_POINT('',#21418);
#6231=VERTEX_POINT('',#21420);
#6232=VERTEX_POINT('',#21422);
#6233=VERTEX_POINT('',#21447);
#6234=VERTEX_POINT('',#21448);
#6235=VERTEX_POINT('',#21450);
#6236=VERTEX_POINT('',#21452);
#6237=VERTEX_POINT('',#21456);
#6238=VERTEX_POINT('',#21458);
#6239=VERTEX_POINT('',#21460);
#6240=VERTEX_POINT('',#21462);
#6241=VERTEX_POINT('',#21466);
#6242=VERTEX_POINT('',#21468);
#6243=VERTEX_POINT('',#21472);
#6244=VERTEX_POINT('',#21474);
#6245=VERTEX_POINT('',#21479);
#6246=VERTEX_POINT('',#21481);
#6247=VERTEX_POINT('',#21485);
#6248=VERTEX_POINT('',#21489);
#6249=VERTEX_POINT('',#21491);
#6250=VERTEX_POINT('',#21495);
#6251=VERTEX_POINT('',#21497);
#6252=VERTEX_POINT('',#21501);
#6253=VERTEX_POINT('',#21503);
#6254=VERTEX_POINT('',#21507);
#6255=VERTEX_POINT('',#21509);
#6256=VERTEX_POINT('',#21513);
#6257=VERTEX_POINT('',#21515);
#6258=VERTEX_POINT('',#21519);
#6259=VERTEX_POINT('',#21523);
#6260=VERTEX_POINT('',#21525);
#6261=VERTEX_POINT('',#21534);
#6262=VERTEX_POINT('',#21535);
#6263=VERTEX_POINT('',#21537);
#6264=VERTEX_POINT('',#21539);
#6265=VERTEX_POINT('',#21543);
#6266=VERTEX_POINT('',#21544);
#6267=VERTEX_POINT('',#21549);
#6268=VERTEX_POINT('',#21553);
#6269=VERTEX_POINT('',#21557);
#6270=VERTEX_POINT('',#21558);
#6271=VERTEX_POINT('',#21560);
#6272=VERTEX_POINT('',#21562);
#6273=VERTEX_POINT('',#21566);
#6274=VERTEX_POINT('',#21567);
#6275=VERTEX_POINT('',#21569);
#6276=VERTEX_POINT('',#21574);
#6277=VERTEX_POINT('',#21578);
#6278=VERTEX_POINT('',#21579);
#6279=VERTEX_POINT('',#21581);
#6280=VERTEX_POINT('',#21583);
#6281=VERTEX_POINT('',#21587);
#6282=VERTEX_POINT('',#21588);
#6283=VERTEX_POINT('',#21593);
#6284=VERTEX_POINT('',#21594);
#6285=VERTEX_POINT('',#21599);
#6286=VERTEX_POINT('',#21601);
#6287=VERTEX_POINT('',#21605);
#6288=VERTEX_POINT('',#21612);
#6289=VERTEX_POINT('',#21614);
#6290=VERTEX_POINT('',#21621);
#6291=VERTEX_POINT('',#21622);
#6292=VERTEX_POINT('',#21627);
#6293=VERTEX_POINT('',#21631);
#6294=VERTEX_POINT('',#21638);
#6295=VERTEX_POINT('',#21639);
#6296=VERTEX_POINT('',#21641);
#6297=VERTEX_POINT('',#21643);
#6298=VERTEX_POINT('',#21647);
#6299=VERTEX_POINT('',#21648);
#6300=VERTEX_POINT('',#21650);
#6301=VERTEX_POINT('',#21652);
#6302=VERTEX_POINT('',#21656);
#6303=VERTEX_POINT('',#21658);
#6304=VERTEX_POINT('',#21660);
#6305=VERTEX_POINT('',#21662);
#6306=VERTEX_POINT('',#21668);
#6307=VERTEX_POINT('',#21670);
#6308=VERTEX_POINT('',#21674);
#6309=VERTEX_POINT('',#21676);
#6310=VERTEX_POINT('',#21680);
#6311=VERTEX_POINT('',#21686);
#6312=VERTEX_POINT('',#21690);
#6313=VERTEX_POINT('',#21699);
#6314=VERTEX_POINT('',#21701);
#6315=VERTEX_POINT('',#27645);
#6316=VERTEX_POINT('',#27789);
#6317=VERTEX_POINT('',#33843);
#6318=VERTEX_POINT('',#33844);
#6319=VERTEX_POINT('',#33846);
#6320=VERTEX_POINT('',#33848);
#6321=VERTEX_POINT('',#33852);
#6322=VERTEX_POINT('',#33854);
#6323=VERTEX_POINT('',#33858);
#6324=VERTEX_POINT('',#33860);
#6325=VERTEX_POINT('',#33865);
#6326=VERTEX_POINT('',#33866);
#6327=VERTEX_POINT('',#33868);
#6328=VERTEX_POINT('',#33870);
#6329=VERTEX_POINT('',#33889);
#6330=VERTEX_POINT('',#33890);
#6331=VERTEX_POINT('',#33892);
#6332=VERTEX_POINT('',#33894);
#6333=VERTEX_POINT('',#33898);
#6334=VERTEX_POINT('',#33900);
#6335=VERTEX_POINT('',#33904);
#6336=VERTEX_POINT('',#33909);
#7623=EDGE_CURVE('',#6221,#6221,#5509,.T.);
#7624=EDGE_CURVE('',#6221,#6222,#5510,.T.);
#7625=EDGE_CURVE('',#6222,#6222,#5511,.T.);
#7626=EDGE_CURVE('',#6221,#6223,#1057,.T.);
#7627=EDGE_CURVE('',#6223,#6223,#5512,.T.);
#7628=EDGE_CURVE('',#6224,#6224,#5513,.T.);
#7629=EDGE_CURVE('',#6224,#6222,#1058,.T.);
#7630=EDGE_CURVE('',#6225,#6225,#5514,.T.);
#7631=EDGE_CURVE('',#6225,#6226,#1059,.T.);
#7632=EDGE_CURVE('',#6226,#6226,#5515,.T.);
#7633=EDGE_CURVE('',#6227,#6227,#5516,.T.);
#7634=EDGE_CURVE('',#6227,#6228,#1060,.T.);
#7635=EDGE_CURVE('',#6228,#6228,#5517,.T.);
#7636=EDGE_CURVE('',#6229,#6229,#5518,.T.);
#7637=EDGE_CURVE('',#6229,#6230,#1061,.T.);
#7638=EDGE_CURVE('',#6231,#6230,#5519,.T.);
#7639=EDGE_CURVE('',#6231,#6232,#795,.T.);
#7640=EDGE_CURVE('',#6230,#6232,#5520,.T.);
#7641=EDGE_CURVE('',#6233,#6234,#5521,.T.);
#7642=EDGE_CURVE('',#6235,#6233,#1062,.T.);
#7643=EDGE_CURVE('',#6235,#6236,#5522,.T.);
#7644=EDGE_CURVE('',#6236,#6234,#1063,.T.);
#7645=EDGE_CURVE('',#6232,#6237,#735,.T.);
#7646=EDGE_CURVE('',#6237,#6238,#5523,.T.);
#7647=EDGE_CURVE('',#6238,#6239,#5524,.T.);
#7648=EDGE_CURVE('',#6239,#6240,#5525,.T.);
#7649=EDGE_CURVE('',#6240,#6231,#736,.T.);
#7650=EDGE_CURVE('',#6241,#6241,#5526,.T.);
#7651=EDGE_CURVE('',#6241,#6242,#1064,.T.);
#7652=EDGE_CURVE('',#6242,#6242,#5527,.T.);
#7653=EDGE_CURVE('',#6243,#6243,#5528,.T.);
#7654=EDGE_CURVE('',#6243,#6244,#1065,.T.);
#7655=EDGE_CURVE('',#6238,#6244,#737,.T.);
#7656=EDGE_CURVE('',#6244,#6239,#738,.T.);
#7657=EDGE_CURVE('',#6245,#6245,#5529,.T.);
#7658=EDGE_CURVE('',#6245,#6246,#1066,.T.);
#7659=EDGE_CURVE('',#6246,#6246,#5530,.T.);
#7660=EDGE_CURVE('',#6245,#6247,#1067,.T.);
#7661=EDGE_CURVE('',#6247,#6247,#5531,.T.);
#7662=EDGE_CURVE('',#6248,#6248,#5532,.T.);
#7663=EDGE_CURVE('',#6248,#6249,#1068,.T.);
#7664=EDGE_CURVE('',#6249,#6249,#5533,.T.);
#7665=EDGE_CURVE('',#6250,#6250,#5534,.T.);
#7666=EDGE_CURVE('',#6250,#6251,#1069,.T.);
#7667=EDGE_CURVE('',#6251,#6251,#5535,.T.);
#7668=EDGE_CURVE('',#6252,#6252,#5536,.T.);
#7669=EDGE_CURVE('',#6252,#6253,#1070,.T.);
#7670=EDGE_CURVE('',#6253,#6253,#5537,.T.);
#7671=EDGE_CURVE('',#6254,#6254,#5538,.T.);
#7672=EDGE_CURVE('',#6254,#6255,#5539,.T.);
#7673=EDGE_CURVE('',#6255,#6255,#5540,.T.);
#7674=EDGE_CURVE('',#6256,#6256,#5541,.T.);
#7675=EDGE_CURVE('',#6256,#6257,#1071,.T.);
#7676=EDGE_CURVE('',#6257,#6257,#5542,.T.);
#7677=EDGE_CURVE('',#6258,#6258,#5543,.T.);
#7678=EDGE_CURVE('',#6258,#6257,#1072,.T.);
#7679=EDGE_CURVE('',#6259,#6259,#5544,.T.);
#7680=EDGE_CURVE('',#6259,#6260,#1073,.T.);
#7681=EDGE_CURVE('',#6260,#6260,#5545,.T.);
#7682=EDGE_CURVE('',#6261,#6262,#1074,.T.);
#7683=EDGE_CURVE('',#6263,#6261,#1075,.T.);
#7684=EDGE_CURVE('',#6264,#6263,#1076,.T.);
#7685=EDGE_CURVE('',#6262,#6264,#1077,.T.);
#7686=EDGE_CURVE('',#6265,#6266,#1078,.T.);
#7687=EDGE_CURVE('',#6263,#6265,#1079,.T.);
#7688=EDGE_CURVE('',#6261,#6266,#1080,.T.);
#7689=EDGE_CURVE('',#6267,#6265,#1081,.T.);
#7690=EDGE_CURVE('',#6264,#6267,#1082,.T.);
#7691=EDGE_CURVE('',#6268,#6267,#1083,.T.);
#7692=EDGE_CURVE('',#6262,#6268,#1084,.T.);
#7693=EDGE_CURVE('',#6269,#6270,#1085,.T.);
#7694=EDGE_CURVE('',#6271,#6269,#1086,.T.);
#7695=EDGE_CURVE('',#6272,#6271,#1087,.T.);
#7696=EDGE_CURVE('',#6270,#6272,#1088,.T.);
#7697=EDGE_CURVE('',#6273,#6274,#1089,.T.);
#7698=EDGE_CURVE('',#6273,#6275,#1090,.T.);
#7699=EDGE_CURVE('',#6272,#6275,#1091,.T.);
#7700=EDGE_CURVE('',#6271,#6274,#1092,.T.);
#7701=EDGE_CURVE('',#6275,#6276,#1093,.T.);
#7702=EDGE_CURVE('',#6270,#6276,#1094,.T.);
#7703=EDGE_CURVE('',#6277,#6278,#1095,.T.);
#7704=EDGE_CURVE('',#6277,#6279,#1096,.T.);
#7705=EDGE_CURVE('',#6279,#6280,#1097,.T.);
#7706=EDGE_CURVE('',#6278,#6280,#1098,.T.);
#7707=EDGE_CURVE('',#6281,#6282,#1099,.T.);
#7708=EDGE_CURVE('',#6281,#6277,#1100,.T.);
#7709=EDGE_CURVE('',#6282,#6278,#1101,.T.);
#7710=EDGE_CURVE('',#6283,#6284,#1102,.T.);
#7711=EDGE_CURVE('',#6283,#6281,#1103,.T.);
#7712=EDGE_CURVE('',#6284,#6282,#1104,.T.);
#7713=EDGE_CURVE('',#6278,#6285,#1105,.T.);
#7714=EDGE_CURVE('',#6285,#6286,#1106,.T.);
#7715=EDGE_CURVE('',#6282,#6286,#1107,.T.);
#7716=EDGE_CURVE('',#6280,#6287,#1108,.T.);
#7717=EDGE_CURVE('',#6287,#6285,#1109,.T.);
#7718=EDGE_CURVE('',#6271,#6283,#1110,.T.);
#7719=EDGE_CURVE('',#6274,#6284,#1111,.T.);
#7720=EDGE_CURVE('',#6288,#6287,#1112,.T.);
#7721=EDGE_CURVE('',#6280,#6289,#1113,.T.);
#7722=EDGE_CURVE('',#6274,#6289,#1114,.T.);
#7723=EDGE_CURVE('',#6284,#6288,#1115,.T.);
#7724=EDGE_CURVE('',#6286,#6288,#1116,.T.);
#7725=EDGE_CURVE('',#6290,#6291,#1117,.T.);
#7726=EDGE_CURVE('',#6286,#6291,#1118,.T.);
#7727=EDGE_CURVE('',#6285,#6290,#1119,.T.);
#7728=EDGE_CURVE('',#6292,#6290,#1120,.T.);
#7729=EDGE_CURVE('',#6287,#6292,#1121,.T.);
#7730=EDGE_CURVE('',#6293,#6292,#1122,.T.);
#7731=EDGE_CURVE('',#6288,#6293,#1123,.T.);
#7732=EDGE_CURVE('',#6291,#6293,#1124,.T.);
#7733=EDGE_CURVE('',#6294,#6295,#1125,.T.);
#7734=EDGE_CURVE('',#6295,#6296,#1126,.T.);
#7735=EDGE_CURVE('',#6296,#6297,#1127,.T.);
#7736=EDGE_CURVE('',#6297,#6294,#1128,.T.);
#7737=EDGE_CURVE('',#6298,#6299,#1129,.T.);
#7738=EDGE_CURVE('',#6299,#6300,#1130,.T.);
#7739=EDGE_CURVE('',#6301,#6300,#1131,.T.);
#7740=EDGE_CURVE('',#6298,#6301,#1132,.T.);
#7741=EDGE_CURVE('',#6300,#6302,#1133,.T.);
#7742=EDGE_CURVE('',#6302,#6303,#1134,.T.);
#7743=EDGE_CURVE('',#6303,#6304,#1135,.T.);
#7744=EDGE_CURVE('',#6305,#6304,#1136,.T.);
#7745=EDGE_CURVE('',#6301,#6305,#1137,.T.);
#7746=EDGE_CURVE('',#6266,#6268,#1138,.T.);
#7747=EDGE_CURVE('',#6306,#6302,#1139,.T.);
#7748=EDGE_CURVE('',#6307,#6306,#1140,.T.);
#7749=EDGE_CURVE('',#6303,#6307,#1141,.T.);
#7750=EDGE_CURVE('',#6304,#6308,#1142,.T.);
#7751=EDGE_CURVE('',#6309,#6308,#1143,.T.);
#7752=EDGE_CURVE('',#6305,#6309,#1144,.T.);
#7753=EDGE_CURVE('',#6310,#6299,#1145,.T.);
#7754=EDGE_CURVE('',#6310,#6295,#1146,.T.);
#7755=EDGE_CURVE('',#6295,#6306,#1147,.T.);
#7756=EDGE_CURVE('',#6307,#6296,#1148,.T.);
#7757=EDGE_CURVE('',#6296,#6311,#1149,.T.);
#7758=EDGE_CURVE('',#6308,#6311,#1150,.T.);
#7759=EDGE_CURVE('',#6289,#6312,#1151,.T.);
#7760=EDGE_CURVE('',#6312,#6273,#1152,.T.);
#7761=EDGE_CURVE('',#6311,#6310,#1153,.T.);
#7762=EDGE_CURVE('',#6309,#6298,#1154,.T.);
#7763=EDGE_CURVE('',#6276,#6312,#1155,.T.);
#7764=EDGE_CURVE('',#6313,#6307,#1156,.T.);
#7765=EDGE_CURVE('',#6306,#6314,#1157,.T.);
#7766=EDGE_CURVE('',#6314,#6313,#1158,.T.);
#7767=EDGE_CURVE('',#6313,#6277,#1159,.T.);
#7768=EDGE_CURVE('',#6279,#6314,#1160,.T.);
#7769=EDGE_CURVE('',#6283,#6294,#1161,.T.);
#7770=EDGE_CURVE('',#6279,#6269,#1162,.T.);
#7771=EDGE_CURVE('',#6297,#6281,#1163,.T.);
#7772=EDGE_CURVE('',#6269,#6289,#1164,.T.);
#7773=EDGE_CURVE('',#6244,#6315,#796,.T.);
#7774=EDGE_CURVE('',#6315,#6239,#5546,.T.);
#7775=EDGE_CURVE('',#6316,#6238,#5547,.T.);
#7776=EDGE_CURVE('',#6315,#6316,#5548,.T.);
#7777=EDGE_CURVE('',#6316,#6244,#797,.T.);
#7778=EDGE_CURVE('',#6317,#6318,#5549,.T.);
#7779=EDGE_CURVE('',#6319,#6317,#1165,.T.);
#7780=EDGE_CURVE('',#6319,#6320,#5550,.T.);
#7781=EDGE_CURVE('',#6320,#6318,#1166,.T.);
#7782=EDGE_CURVE('',#6318,#6321,#1167,.T.);
#7783=EDGE_CURVE('',#6320,#6322,#1168,.T.);
#7784=EDGE_CURVE('',#6322,#6321,#1169,.T.);
#7785=EDGE_CURVE('',#6321,#6323,#5551,.T.);
#7786=EDGE_CURVE('',#6322,#6324,#5552,.T.);
#7787=EDGE_CURVE('',#6324,#6323,#1170,.T.);
#7788=EDGE_CURVE('',#6325,#6326,#1171,.T.);
#7789=EDGE_CURVE('',#6327,#6325,#1172,.T.);
#7790=EDGE_CURVE('',#6327,#6328,#1173,.T.);
#7791=EDGE_CURVE('',#6328,#6326,#1174,.T.);
#7792=EDGE_CURVE('',#6323,#6325,#1175,.T.);
#7793=EDGE_CURVE('',#6324,#6327,#1176,.T.);
#7794=EDGE_CURVE('',#6326,#6233,#1177,.T.);
#7795=EDGE_CURVE('',#6328,#6235,#1178,.T.);
#7796=EDGE_CURVE('',#6234,#6317,#1179,.T.);
#7797=EDGE_CURVE('',#6236,#6319,#1180,.T.);
#7798=EDGE_CURVE('',#6329,#6330,#1181,.T.);
#7799=EDGE_CURVE('',#6331,#6330,#1182,.T.);
#7800=EDGE_CURVE('',#6332,#6331,#1183,.T.);
#7801=EDGE_CURVE('',#6332,#6329,#1184,.T.);
#7802=EDGE_CURVE('',#6333,#6329,#1185,.T.);
#7803=EDGE_CURVE('',#6334,#6332,#1186,.T.);
#7804=EDGE_CURVE('',#6334,#6333,#1187,.T.);
#7805=EDGE_CURVE('',#6335,#6333,#1188,.T.);
#7806=EDGE_CURVE('',#6330,#6335,#1189,.T.);
#7807=EDGE_CURVE('',#6336,#6335,#1190,.T.);
#7808=EDGE_CURVE('',#6331,#6336,#1191,.T.);
#7809=EDGE_CURVE('',#6336,#6334,#1192,.T.);
#9833=ORIENTED_EDGE('',*,*,#7623,.T.);
#9834=ORIENTED_EDGE('',*,*,#7624,.T.);
#9835=ORIENTED_EDGE('',*,*,#7625,.T.);
#9836=ORIENTED_EDGE('',*,*,#7624,.F.);
#9837=ORIENTED_EDGE('',*,*,#7623,.F.);
#9838=ORIENTED_EDGE('',*,*,#7626,.T.);
#9839=ORIENTED_EDGE('',*,*,#7627,.T.);
#9840=ORIENTED_EDGE('',*,*,#7626,.F.);
#9841=ORIENTED_EDGE('',*,*,#7628,.T.);
#9842=ORIENTED_EDGE('',*,*,#7629,.T.);
#9843=ORIENTED_EDGE('',*,*,#7625,.F.);
#9844=ORIENTED_EDGE('',*,*,#7629,.F.);
#9845=ORIENTED_EDGE('',*,*,#7630,.F.);
#9846=ORIENTED_EDGE('',*,*,#7631,.T.);
#9847=ORIENTED_EDGE('',*,*,#7632,.F.);
#9848=ORIENTED_EDGE('',*,*,#7631,.F.);
#9849=ORIENTED_EDGE('',*,*,#7633,.F.);
#9850=ORIENTED_EDGE('',*,*,#7634,.T.);
#9851=ORIENTED_EDGE('',*,*,#7635,.T.);
#9852=ORIENTED_EDGE('',*,*,#7634,.F.);
#9853=ORIENTED_EDGE('',*,*,#7636,.T.);
#9854=ORIENTED_EDGE('',*,*,#7637,.T.);
#9855=ORIENTED_EDGE('',*,*,#7638,.F.);
#9856=ORIENTED_EDGE('',*,*,#7639,.T.);
#9857=ORIENTED_EDGE('',*,*,#7640,.F.);
#9858=ORIENTED_EDGE('',*,*,#7637,.F.);
#9859=ORIENTED_EDGE('',*,*,#7641,.F.);
#9860=ORIENTED_EDGE('',*,*,#7642,.F.);
#9861=ORIENTED_EDGE('',*,*,#7643,.T.);
#9862=ORIENTED_EDGE('',*,*,#7644,.T.);
#9863=ORIENTED_EDGE('',*,*,#7638,.T.);
#9864=ORIENTED_EDGE('',*,*,#7640,.T.);
#9865=ORIENTED_EDGE('',*,*,#7645,.T.);
#9866=ORIENTED_EDGE('',*,*,#7646,.T.);
#9867=ORIENTED_EDGE('',*,*,#7647,.T.);
#9868=ORIENTED_EDGE('',*,*,#7648,.T.);
#9869=ORIENTED_EDGE('',*,*,#7649,.T.);
#9870=ORIENTED_EDGE('',*,*,#7650,.T.);
#9871=ORIENTED_EDGE('',*,*,#7651,.T.);
#9872=ORIENTED_EDGE('',*,*,#7652,.T.);
#9873=ORIENTED_EDGE('',*,*,#7651,.F.);
#9874=ORIENTED_EDGE('',*,*,#7653,.F.);
#9875=ORIENTED_EDGE('',*,*,#7654,.T.);
#9876=ORIENTED_EDGE('',*,*,#7655,.F.);
#9877=ORIENTED_EDGE('',*,*,#7646,.F.);
#9878=ORIENTED_EDGE('',*,*,#7645,.F.);
#9879=ORIENTED_EDGE('',*,*,#7639,.F.);
#9880=ORIENTED_EDGE('',*,*,#7649,.F.);
#9881=ORIENTED_EDGE('',*,*,#7648,.F.);
#9882=ORIENTED_EDGE('',*,*,#7656,.F.);
#9883=ORIENTED_EDGE('',*,*,#7654,.F.);
#9884=ORIENTED_EDGE('',*,*,#7657,.T.);
#9885=ORIENTED_EDGE('',*,*,#7658,.T.);
#9886=ORIENTED_EDGE('',*,*,#7659,.F.);
#9887=ORIENTED_EDGE('',*,*,#7658,.F.);
#9888=ORIENTED_EDGE('',*,*,#7657,.F.);
#9889=ORIENTED_EDGE('',*,*,#7660,.T.);
#9890=ORIENTED_EDGE('',*,*,#7661,.T.);
#9891=ORIENTED_EDGE('',*,*,#7660,.F.);
#9892=ORIENTED_EDGE('',*,*,#7662,.F.);
#9893=ORIENTED_EDGE('',*,*,#7663,.T.);
#9894=ORIENTED_EDGE('',*,*,#7664,.T.);
#9895=ORIENTED_EDGE('',*,*,#7663,.F.);
#9896=ORIENTED_EDGE('',*,*,#7665,.T.);
#9897=ORIENTED_EDGE('',*,*,#7666,.T.);
#9898=ORIENTED_EDGE('',*,*,#7667,.F.);
#9899=ORIENTED_EDGE('',*,*,#7666,.F.);
#9900=ORIENTED_EDGE('',*,*,#7668,.T.);
#9901=ORIENTED_EDGE('',*,*,#7669,.T.);
#9902=ORIENTED_EDGE('',*,*,#7670,.F.);
#9903=ORIENTED_EDGE('',*,*,#7669,.F.);
#9904=ORIENTED_EDGE('',*,*,#7671,.F.);
#9905=ORIENTED_EDGE('',*,*,#7672,.T.);
#9906=ORIENTED_EDGE('',*,*,#7673,.T.);
#9907=ORIENTED_EDGE('',*,*,#7672,.F.);
#9908=ORIENTED_EDGE('',*,*,#7674,.T.);
#9909=ORIENTED_EDGE('',*,*,#7675,.T.);
#9910=ORIENTED_EDGE('',*,*,#7676,.F.);
#9911=ORIENTED_EDGE('',*,*,#7675,.F.);
#9912=ORIENTED_EDGE('',*,*,#7677,.F.);
#9913=ORIENTED_EDGE('',*,*,#7678,.T.);
#9914=ORIENTED_EDGE('',*,*,#7676,.T.);
#9915=ORIENTED_EDGE('',*,*,#7678,.F.);
#9916=ORIENTED_EDGE('',*,*,#7679,.T.);
#9917=ORIENTED_EDGE('',*,*,#7680,.T.);
#9918=ORIENTED_EDGE('',*,*,#7681,.F.);
#9919=ORIENTED_EDGE('',*,*,#7680,.F.);
#9920=ORIENTED_EDGE('',*,*,#7679,.F.);
#9921=ORIENTED_EDGE('',*,*,#7677,.T.);
#9922=ORIENTED_EDGE('',*,*,#7671,.T.);
#9923=ORIENTED_EDGE('',*,*,#7674,.F.);
#9924=ORIENTED_EDGE('',*,*,#7673,.F.);
#9925=ORIENTED_EDGE('',*,*,#7670,.T.);
#9926=ORIENTED_EDGE('',*,*,#7667,.T.);
#9927=ORIENTED_EDGE('',*,*,#7664,.F.);
#9928=ORIENTED_EDGE('',*,*,#7682,.F.);
#9929=ORIENTED_EDGE('',*,*,#7683,.F.);
#9930=ORIENTED_EDGE('',*,*,#7684,.F.);
#9931=ORIENTED_EDGE('',*,*,#7685,.F.);
#9932=ORIENTED_EDGE('',*,*,#7686,.F.);
#9933=ORIENTED_EDGE('',*,*,#7687,.F.);
#9934=ORIENTED_EDGE('',*,*,#7683,.T.);
#9935=ORIENTED_EDGE('',*,*,#7688,.T.);
#9936=ORIENTED_EDGE('',*,*,#7689,.F.);
#9937=ORIENTED_EDGE('',*,*,#7690,.F.);
#9938=ORIENTED_EDGE('',*,*,#7684,.T.);
#9939=ORIENTED_EDGE('',*,*,#7687,.T.);
#9940=ORIENTED_EDGE('',*,*,#7691,.F.);
#9941=ORIENTED_EDGE('',*,*,#7692,.F.);
#9942=ORIENTED_EDGE('',*,*,#7685,.T.);
#9943=ORIENTED_EDGE('',*,*,#7690,.T.);
#9944=ORIENTED_EDGE('',*,*,#7693,.F.);
#9945=ORIENTED_EDGE('',*,*,#7694,.F.);
#9946=ORIENTED_EDGE('',*,*,#7695,.F.);
#9947=ORIENTED_EDGE('',*,*,#7696,.F.);
#9948=ORIENTED_EDGE('',*,*,#7697,.F.);
#9949=ORIENTED_EDGE('',*,*,#7698,.T.);
#9950=ORIENTED_EDGE('',*,*,#7699,.F.);
#9951=ORIENTED_EDGE('',*,*,#7695,.T.);
#9952=ORIENTED_EDGE('',*,*,#7700,.T.);
#9953=ORIENTED_EDGE('',*,*,#7699,.T.);
#9954=ORIENTED_EDGE('',*,*,#7701,.T.);
#9955=ORIENTED_EDGE('',*,*,#7702,.F.);
#9956=ORIENTED_EDGE('',*,*,#7696,.T.);
#9957=ORIENTED_EDGE('',*,*,#7703,.F.);
#9958=ORIENTED_EDGE('',*,*,#7704,.T.);
#9959=ORIENTED_EDGE('',*,*,#7705,.T.);
#9960=ORIENTED_EDGE('',*,*,#7706,.F.);
#9961=ORIENTED_EDGE('',*,*,#7707,.F.);
#9962=ORIENTED_EDGE('',*,*,#7708,.T.);
#9963=ORIENTED_EDGE('',*,*,#7703,.T.);
#9964=ORIENTED_EDGE('',*,*,#7709,.F.);
#9965=ORIENTED_EDGE('',*,*,#7710,.F.);
#9966=ORIENTED_EDGE('',*,*,#7711,.T.);
#9967=ORIENTED_EDGE('',*,*,#7707,.T.);
#9968=ORIENTED_EDGE('',*,*,#7712,.F.);
#9969=ORIENTED_EDGE('',*,*,#7713,.T.);
#9970=ORIENTED_EDGE('',*,*,#7714,.T.);
#9971=ORIENTED_EDGE('',*,*,#7715,.F.);
#9972=ORIENTED_EDGE('',*,*,#7709,.T.);
#9973=ORIENTED_EDGE('',*,*,#7716,.T.);
#9974=ORIENTED_EDGE('',*,*,#7717,.T.);
#9975=ORIENTED_EDGE('',*,*,#7713,.F.);
#9976=ORIENTED_EDGE('',*,*,#7706,.T.);
#9977=ORIENTED_EDGE('',*,*,#7700,.F.);
#9978=ORIENTED_EDGE('',*,*,#7718,.T.);
#9979=ORIENTED_EDGE('',*,*,#7710,.T.);
#9980=ORIENTED_EDGE('',*,*,#7719,.F.);
#9981=ORIENTED_EDGE('',*,*,#7720,.T.);
#9982=ORIENTED_EDGE('',*,*,#7716,.F.);
#9983=ORIENTED_EDGE('',*,*,#7721,.T.);
#9984=ORIENTED_EDGE('',*,*,#7722,.F.);
#9985=ORIENTED_EDGE('',*,*,#7719,.T.);
#9986=ORIENTED_EDGE('',*,*,#7723,.T.);
#9987=ORIENTED_EDGE('',*,*,#7715,.T.);
#9988=ORIENTED_EDGE('',*,*,#7724,.T.);
#9989=ORIENTED_EDGE('',*,*,#7723,.F.);
#9990=ORIENTED_EDGE('',*,*,#7712,.T.);
#9991=ORIENTED_EDGE('',*,*,#7725,.T.);
#9992=ORIENTED_EDGE('',*,*,#7726,.F.);
#9993=ORIENTED_EDGE('',*,*,#7714,.F.);
#9994=ORIENTED_EDGE('',*,*,#7727,.T.);
#9995=ORIENTED_EDGE('',*,*,#7728,.T.);
#9996=ORIENTED_EDGE('',*,*,#7727,.F.);
#9997=ORIENTED_EDGE('',*,*,#7717,.F.);
#9998=ORIENTED_EDGE('',*,*,#7729,.T.);
#9999=ORIENTED_EDGE('',*,*,#7730,.T.);
#10000=ORIENTED_EDGE('',*,*,#7729,.F.);
#10001=ORIENTED_EDGE('',*,*,#7720,.F.);
#10002=ORIENTED_EDGE('',*,*,#7731,.T.);
#10003=ORIENTED_EDGE('',*,*,#7732,.T.);
#10004=ORIENTED_EDGE('',*,*,#7731,.F.);
#10005=ORIENTED_EDGE('',*,*,#7724,.F.);
#10006=ORIENTED_EDGE('',*,*,#7726,.T.);
#10007=ORIENTED_EDGE('',*,*,#7659,.T.);
#10008=ORIENTED_EDGE('',*,*,#7650,.F.);
#10009=ORIENTED_EDGE('',*,*,#7733,.T.);
#10010=ORIENTED_EDGE('',*,*,#7734,.T.);
#10011=ORIENTED_EDGE('',*,*,#7735,.T.);
#10012=ORIENTED_EDGE('',*,*,#7736,.T.);
#10013=ORIENTED_EDGE('',*,*,#7737,.T.);
#10014=ORIENTED_EDGE('',*,*,#7738,.T.);
#10015=ORIENTED_EDGE('',*,*,#7739,.F.);
#10016=ORIENTED_EDGE('',*,*,#7740,.F.);
#10017=ORIENTED_EDGE('',*,*,#7741,.T.);
#10018=ORIENTED_EDGE('',*,*,#7742,.T.);
#10019=ORIENTED_EDGE('',*,*,#7743,.T.);
#10020=ORIENTED_EDGE('',*,*,#7744,.F.);
#10021=ORIENTED_EDGE('',*,*,#7745,.F.);
#10022=ORIENTED_EDGE('',*,*,#7739,.T.);
#10023=ORIENTED_EDGE('',*,*,#7746,.F.);
#10024=ORIENTED_EDGE('',*,*,#7688,.F.);
#10025=ORIENTED_EDGE('',*,*,#7682,.T.);
#10026=ORIENTED_EDGE('',*,*,#7692,.T.);
#10027=ORIENTED_EDGE('',*,*,#7747,.F.);
#10028=ORIENTED_EDGE('',*,*,#7748,.F.);
#10029=ORIENTED_EDGE('',*,*,#7749,.F.);
#10030=ORIENTED_EDGE('',*,*,#7742,.F.);
#10031=ORIENTED_EDGE('',*,*,#7744,.T.);
#10032=ORIENTED_EDGE('',*,*,#7750,.T.);
#10033=ORIENTED_EDGE('',*,*,#7751,.F.);
#10034=ORIENTED_EDGE('',*,*,#7752,.F.);
#10035=ORIENTED_EDGE('',*,*,#7753,.F.);
#10036=ORIENTED_EDGE('',*,*,#7754,.T.);
#10037=ORIENTED_EDGE('',*,*,#7755,.T.);
#10038=ORIENTED_EDGE('',*,*,#7747,.T.);
#10039=ORIENTED_EDGE('',*,*,#7741,.F.);
#10040=ORIENTED_EDGE('',*,*,#7738,.F.);
#10041=ORIENTED_EDGE('',*,*,#7743,.F.);
#10042=ORIENTED_EDGE('',*,*,#7749,.T.);
#10043=ORIENTED_EDGE('',*,*,#7756,.T.);
#10044=ORIENTED_EDGE('',*,*,#7757,.T.);
#10045=ORIENTED_EDGE('',*,*,#7758,.F.);
#10046=ORIENTED_EDGE('',*,*,#7750,.F.);
#10047=ORIENTED_EDGE('',*,*,#7759,.T.);
#10048=ORIENTED_EDGE('',*,*,#7760,.T.);
#10049=ORIENTED_EDGE('',*,*,#7697,.T.);
#10050=ORIENTED_EDGE('',*,*,#7722,.T.);
#10051=ORIENTED_EDGE('',*,*,#7758,.T.);
#10052=ORIENTED_EDGE('',*,*,#7761,.T.);
#10053=ORIENTED_EDGE('',*,*,#7753,.T.);
#10054=ORIENTED_EDGE('',*,*,#7737,.F.);
#10055=ORIENTED_EDGE('',*,*,#7762,.F.);
#10056=ORIENTED_EDGE('',*,*,#7751,.T.);
#10057=ORIENTED_EDGE('',*,*,#7763,.F.);
#10058=ORIENTED_EDGE('',*,*,#7701,.F.);
#10059=ORIENTED_EDGE('',*,*,#7698,.F.);
#10060=ORIENTED_EDGE('',*,*,#7760,.F.);
#10061=ORIENTED_EDGE('',*,*,#7764,.T.);
#10062=ORIENTED_EDGE('',*,*,#7748,.T.);
#10063=ORIENTED_EDGE('',*,*,#7765,.T.);
#10064=ORIENTED_EDGE('',*,*,#7766,.T.);
#10065=ORIENTED_EDGE('',*,*,#7767,.F.);
#10066=ORIENTED_EDGE('',*,*,#7766,.F.);
#10067=ORIENTED_EDGE('',*,*,#7768,.F.);
#10068=ORIENTED_EDGE('',*,*,#7704,.F.);
#10069=ORIENTED_EDGE('',*,*,#7768,.T.);
#10070=ORIENTED_EDGE('',*,*,#7765,.F.);
#10071=ORIENTED_EDGE('',*,*,#7755,.F.);
#10072=ORIENTED_EDGE('',*,*,#7733,.F.);
#10073=ORIENTED_EDGE('',*,*,#7769,.F.);
#10074=ORIENTED_EDGE('',*,*,#7718,.F.);
#10075=ORIENTED_EDGE('',*,*,#7694,.T.);
#10076=ORIENTED_EDGE('',*,*,#7770,.F.);
#10077=ORIENTED_EDGE('',*,*,#7767,.T.);
#10078=ORIENTED_EDGE('',*,*,#7708,.F.);
#10079=ORIENTED_EDGE('',*,*,#7771,.F.);
#10080=ORIENTED_EDGE('',*,*,#7735,.F.);
#10081=ORIENTED_EDGE('',*,*,#7756,.F.);
#10082=ORIENTED_EDGE('',*,*,#7764,.F.);
#10083=ORIENTED_EDGE('',*,*,#7702,.T.);
#10084=ORIENTED_EDGE('',*,*,#7763,.T.);
#10085=ORIENTED_EDGE('',*,*,#7759,.F.);
#10086=ORIENTED_EDGE('',*,*,#7772,.F.);
#10087=ORIENTED_EDGE('',*,*,#7693,.T.);
#10088=ORIENTED_EDGE('',*,*,#7769,.T.);
#10089=ORIENTED_EDGE('',*,*,#7736,.F.);
#10090=ORIENTED_EDGE('',*,*,#7771,.T.);
#10091=ORIENTED_EDGE('',*,*,#7711,.F.);
#10092=ORIENTED_EDGE('',*,*,#7653,.T.);
#10093=ORIENTED_EDGE('',*,*,#7652,.F.);
#10094=ORIENTED_EDGE('',*,*,#7773,.F.);
#10095=ORIENTED_EDGE('',*,*,#7656,.T.);
#10096=ORIENTED_EDGE('',*,*,#7774,.F.);
#10097=ORIENTED_EDGE('',*,*,#7774,.T.);
#10098=ORIENTED_EDGE('',*,*,#7647,.F.);
#10099=ORIENTED_EDGE('',*,*,#7775,.F.);
#10100=ORIENTED_EDGE('',*,*,#7776,.F.);
#10101=ORIENTED_EDGE('',*,*,#7655,.T.);
#10102=ORIENTED_EDGE('',*,*,#7777,.F.);
#10103=ORIENTED_EDGE('',*,*,#7775,.T.);
#10104=ORIENTED_EDGE('',*,*,#7778,.F.);
#10105=ORIENTED_EDGE('',*,*,#7779,.F.);
#10106=ORIENTED_EDGE('',*,*,#7780,.T.);
#10107=ORIENTED_EDGE('',*,*,#7781,.T.);
#10108=ORIENTED_EDGE('',*,*,#7782,.F.);
#10109=ORIENTED_EDGE('',*,*,#7781,.F.);
#10110=ORIENTED_EDGE('',*,*,#7783,.T.);
#10111=ORIENTED_EDGE('',*,*,#7784,.T.);
#10112=ORIENTED_EDGE('',*,*,#7785,.F.);
#10113=ORIENTED_EDGE('',*,*,#7784,.F.);
#10114=ORIENTED_EDGE('',*,*,#7786,.T.);
#10115=ORIENTED_EDGE('',*,*,#7787,.T.);
#10116=ORIENTED_EDGE('',*,*,#7770,.T.);
#10117=ORIENTED_EDGE('',*,*,#7772,.T.);
#10118=ORIENTED_EDGE('',*,*,#7721,.F.);
#10119=ORIENTED_EDGE('',*,*,#7705,.F.);
#10120=ORIENTED_EDGE('',*,*,#7788,.F.);
#10121=ORIENTED_EDGE('',*,*,#7789,.F.);
#10122=ORIENTED_EDGE('',*,*,#7790,.T.);
#10123=ORIENTED_EDGE('',*,*,#7791,.T.);
#10124=ORIENTED_EDGE('',*,*,#7730,.F.);
#10125=ORIENTED_EDGE('',*,*,#7732,.F.);
#10126=ORIENTED_EDGE('',*,*,#7725,.F.);
#10127=ORIENTED_EDGE('',*,*,#7728,.F.);
#10128=ORIENTED_EDGE('',*,*,#7792,.F.);
#10129=ORIENTED_EDGE('',*,*,#7787,.F.);
#10130=ORIENTED_EDGE('',*,*,#7793,.T.);
#10131=ORIENTED_EDGE('',*,*,#7789,.T.);
#10132=ORIENTED_EDGE('',*,*,#7794,.F.);
#10133=ORIENTED_EDGE('',*,*,#7791,.F.);
#10134=ORIENTED_EDGE('',*,*,#7795,.T.);
#10135=ORIENTED_EDGE('',*,*,#7642,.T.);
#10136=ORIENTED_EDGE('',*,*,#7777,.T.);
#10137=ORIENTED_EDGE('',*,*,#7773,.T.);
#10138=ORIENTED_EDGE('',*,*,#7776,.T.);
#10139=ORIENTED_EDGE('',*,*,#7796,.F.);
#10140=ORIENTED_EDGE('',*,*,#7644,.F.);
#10141=ORIENTED_EDGE('',*,*,#7797,.T.);
#10142=ORIENTED_EDGE('',*,*,#7779,.T.);
#10143=ORIENTED_EDGE('',*,*,#7778,.T.);
#10144=ORIENTED_EDGE('',*,*,#7782,.T.);
#10145=ORIENTED_EDGE('',*,*,#7785,.T.);
#10146=ORIENTED_EDGE('',*,*,#7792,.T.);
#10147=ORIENTED_EDGE('',*,*,#7788,.T.);
#10148=ORIENTED_EDGE('',*,*,#7794,.T.);
#10149=ORIENTED_EDGE('',*,*,#7641,.T.);
#10150=ORIENTED_EDGE('',*,*,#7796,.T.);
#10151=ORIENTED_EDGE('',*,*,#7632,.T.);
#10152=ORIENTED_EDGE('',*,*,#7627,.F.);
#10153=ORIENTED_EDGE('',*,*,#7635,.F.);
#10154=ORIENTED_EDGE('',*,*,#7668,.F.);
#10155=ORIENTED_EDGE('',*,*,#7662,.T.);
#10156=ORIENTED_EDGE('',*,*,#7665,.F.);
#10157=ORIENTED_EDGE('',*,*,#7780,.F.);
#10158=ORIENTED_EDGE('',*,*,#7797,.F.);
#10159=ORIENTED_EDGE('',*,*,#7643,.F.);
#10160=ORIENTED_EDGE('',*,*,#7795,.F.);
#10161=ORIENTED_EDGE('',*,*,#7790,.F.);
#10162=ORIENTED_EDGE('',*,*,#7793,.F.);
#10163=ORIENTED_EDGE('',*,*,#7786,.F.);
#10164=ORIENTED_EDGE('',*,*,#7783,.F.);
#10165=ORIENTED_EDGE('',*,*,#7630,.T.);
#10166=ORIENTED_EDGE('',*,*,#7636,.F.);
#10167=ORIENTED_EDGE('',*,*,#7661,.F.);
#10168=ORIENTED_EDGE('',*,*,#7633,.T.);
#10169=ORIENTED_EDGE('',*,*,#7798,.T.);
#10170=ORIENTED_EDGE('',*,*,#7799,.F.);
#10171=ORIENTED_EDGE('',*,*,#7800,.F.);
#10172=ORIENTED_EDGE('',*,*,#7801,.T.);
#10173=ORIENTED_EDGE('',*,*,#7802,.T.);
#10174=ORIENTED_EDGE('',*,*,#7801,.F.);
#10175=ORIENTED_EDGE('',*,*,#7803,.F.);
#10176=ORIENTED_EDGE('',*,*,#7804,.T.);
#10177=ORIENTED_EDGE('',*,*,#7762,.T.);
#10178=ORIENTED_EDGE('',*,*,#7740,.T.);
#10179=ORIENTED_EDGE('',*,*,#7745,.T.);
#10180=ORIENTED_EDGE('',*,*,#7752,.T.);
#10181=ORIENTED_EDGE('',*,*,#7805,.F.);
#10182=ORIENTED_EDGE('',*,*,#7806,.F.);
#10183=ORIENTED_EDGE('',*,*,#7798,.F.);
#10184=ORIENTED_EDGE('',*,*,#7802,.F.);
#10185=ORIENTED_EDGE('',*,*,#7746,.T.);
#10186=ORIENTED_EDGE('',*,*,#7691,.T.);
#10187=ORIENTED_EDGE('',*,*,#7689,.T.);
#10188=ORIENTED_EDGE('',*,*,#7686,.T.);
#10189=ORIENTED_EDGE('',*,*,#7628,.F.);
#10190=ORIENTED_EDGE('',*,*,#7681,.T.);
#10191=ORIENTED_EDGE('',*,*,#7806,.T.);
#10192=ORIENTED_EDGE('',*,*,#7807,.F.);
#10193=ORIENTED_EDGE('',*,*,#7808,.F.);
#10194=ORIENTED_EDGE('',*,*,#7799,.T.);
#10195=ORIENTED_EDGE('',*,*,#7808,.T.);
#10196=ORIENTED_EDGE('',*,*,#7809,.T.);
#10197=ORIENTED_EDGE('',*,*,#7803,.T.);
#10198=ORIENTED_EDGE('',*,*,#7800,.T.);
#10199=ORIENTED_EDGE('',*,*,#7805,.T.);
#10200=ORIENTED_EDGE('',*,*,#7804,.F.);
#10201=ORIENTED_EDGE('',*,*,#7809,.F.);
#10202=ORIENTED_EDGE('',*,*,#7807,.T.);
#10203=ORIENTED_EDGE('',*,*,#7757,.F.);
#10204=ORIENTED_EDGE('',*,*,#7734,.F.);
#10205=ORIENTED_EDGE('',*,*,#7754,.F.);
#10206=ORIENTED_EDGE('',*,*,#7761,.F.);
#14253=TOROIDAL_SURFACE('',#15339,6.25,1.);
#14254=TOROIDAL_SURFACE('',#15387,4.5,0.75);
#14325=ADVANCED_FACE('',(#3690),#14253,.F.);
#14326=ADVANCED_FACE('',(#3691),#3443,.T.);
#14327=ADVANCED_FACE('',(#3692),#3444,.T.);
#14328=ADVANCED_FACE('',(#3693),#3445,.F.);
#14329=ADVANCED_FACE('',(#3694),#3446,.F.);
#14330=ADVANCED_FACE('',(#3695),#1032,.T.);
#14331=ADVANCED_FACE('',(#3696),#3447,.T.);
#14332=ADVANCED_FACE('',(#3697),#3448,.T.);
#14333=ADVANCED_FACE('',(#3698),#3449,.T.);
#14334=ADVANCED_FACE('',(#3699),#3450,.T.);
#14335=ADVANCED_FACE('',(#3700),#3451,.T.);
#14336=ADVANCED_FACE('',(#3701),#1033,.T.);
#14337=ADVANCED_FACE('',(#3702),#3452,.F.);
#14338=ADVANCED_FACE('',(#3703),#3453,.F.);
#14339=ADVANCED_FACE('',(#3704),#3454,.F.);
#14340=ADVANCED_FACE('',(#3705),#14254,.T.);
#14341=ADVANCED_FACE('',(#3706),#3455,.T.);
#14342=ADVANCED_FACE('',(#3707),#1034,.T.);
#14343=ADVANCED_FACE('',(#3708),#3456,.F.);
#14344=ADVANCED_FACE('',(#3709,#194),#279,.F.);
#14345=ADVANCED_FACE('',(#3710,#195),#280,.F.);
#14346=ADVANCED_FACE('',(#3711,#196),#281,.F.);
#14347=ADVANCED_FACE('',(#3712),#282,.T.);
#14348=ADVANCED_FACE('',(#3713),#283,.F.);
#14349=ADVANCED_FACE('',(#3714),#284,.F.);
#14350=ADVANCED_FACE('',(#3715),#285,.T.);
#14351=ADVANCED_FACE('',(#3716),#286,.T.);
#14352=ADVANCED_FACE('',(#3717),#287,.T.);
#14353=ADVANCED_FACE('',(#3718),#288,.F.);
#14354=ADVANCED_FACE('',(#3719),#289,.T.);
#14355=ADVANCED_FACE('',(#3720),#290,.T.);
#14356=ADVANCED_FACE('',(#3721),#291,.T.);
#14357=ADVANCED_FACE('',(#3722),#292,.T.);
#14358=ADVANCED_FACE('',(#3723),#293,.T.);
#14359=ADVANCED_FACE('',(#3724),#294,.T.);
#14360=ADVANCED_FACE('',(#3725),#295,.T.);
#14361=ADVANCED_FACE('',(#3726),#296,.T.);
#14362=ADVANCED_FACE('',(#3727),#297,.T.);
#14363=ADVANCED_FACE('',(#3728),#298,.T.);
#14364=ADVANCED_FACE('',(#3729),#299,.F.);
#14365=ADVANCED_FACE('',(#3730),#300,.F.);
#14366=ADVANCED_FACE('',(#3731),#301,.F.);
#14367=ADVANCED_FACE('',(#3732),#302,.F.);
#14368=ADVANCED_FACE('',(#3733,#197),#303,.T.);
#14369=ADVANCED_FACE('',(#3734),#304,.F.);
#14370=ADVANCED_FACE('',(#3735),#305,.F.);
#14371=ADVANCED_FACE('',(#3736),#306,.F.);
#14372=ADVANCED_FACE('',(#3737),#307,.T.);
#14373=ADVANCED_FACE('',(#3738),#308,.F.);
#14374=ADVANCED_FACE('',(#3739),#309,.F.);
#14375=ADVANCED_FACE('',(#3740),#310,.F.);
#14376=ADVANCED_FACE('',(#3741),#311,.F.);
#14377=ADVANCED_FACE('',(#3742),#312,.T.);
#14378=ADVANCED_FACE('',(#3743),#313,.F.);
#14379=ADVANCED_FACE('',(#3744),#314,.F.);
#14380=ADVANCED_FACE('',(#3745),#315,.F.);
#14381=ADVANCED_FACE('',(#3746),#316,.T.);
#14382=ADVANCED_FACE('',(#3747),#317,.T.);
#14383=ADVANCED_FACE('',(#3748),#318,.T.);
#14384=ADVANCED_FACE('',(#3749),#319,.T.);
#14385=ADVANCED_FACE('',(#3750),#320,.T.);
#14386=ADVANCED_FACE('',(#3751,#198),#321,.T.);
#14387=ADVANCED_FACE('',(#3752),#192,.T.);
#14388=ADVANCED_FACE('',(#3753),#146,.F.);
#14389=ADVANCED_FACE('',(#3754),#193,.T.);
#14390=ADVANCED_FACE('',(#3755),#3457,.T.);
#14391=ADVANCED_FACE('',(#3756),#322,.T.);
#14392=ADVANCED_FACE('',(#3757),#3458,.T.);
#14393=ADVANCED_FACE('',(#3758),#323,.T.);
#14394=ADVANCED_FACE('',(#3759,#199),#324,.T.);
#14395=ADVANCED_FACE('',(#3760),#325,.T.);
#14396=ADVANCED_FACE('',(#3761),#326,.T.);
#14397=ADVANCED_FACE('',(#3762),#327,.F.);
#14398=ADVANCED_FACE('',(#3763),#328,.T.);
#14399=ADVANCED_FACE('',(#3764,#200,#201),#329,.T.);
#14400=ADVANCED_FACE('',(#3765),#330,.F.);
#14401=ADVANCED_FACE('',(#3766,#202,#203),#331,.F.);
#14402=ADVANCED_FACE('',(#3767,#204,#205),#332,.F.);
#14403=ADVANCED_FACE('',(#3768,#206),#333,.T.);
#14404=ADVANCED_FACE('',(#3769),#334,.F.);
#14405=ADVANCED_FACE('',(#3770),#335,.F.);
#14406=ADVANCED_FACE('',(#3771,#207,#208),#336,.T.);
#14407=ADVANCED_FACE('',(#3772,#209),#337,.F.);
#14408=ADVANCED_FACE('',(#3773),#338,.F.);
#14409=ADVANCED_FACE('',(#3774),#339,.T.);
#14410=ADVANCED_FACE('',(#3775),#340,.F.);
#14411=ADVANCED_FACE('',(#3776),#341,.F.);
#15192=CLOSED_SHELL('',(#14325,#14326,#14327,#14328,#14329,#14330,#14331,
#14332,#14333,#14334,#14335,#14336,#14337,#14338,#14339,#14340,#14341,#14342,
#14343,#14344,#14345,#14346,#14347,#14348,#14349,#14350,#14351,#14352,#14353,
#14354,#14355,#14356,#14357,#14358,#14359,#14360,#14361,#14362,#14363,#14364,
#14365,#14366,#14367,#14368,#14369,#14370,#14371,#14372,#14373,#14374,#14375,
#14376,#14377,#14378,#14379,#14380,#14381,#14382,#14383,#14384,#14385,#14386,
#14387,#14388,#14389,#14390,#14391,#14392,#14393,#14394,#14395,#14396,#14397,
#14398,#14399,#14400,#14401,#14402,#14403,#14404,#14405,#14406,#14407,#14408,
#14409,#14410,#14411));
#15338=AXIS2_PLACEMENT_3D('',#21388,#16958,#16959);
#15339=AXIS2_PLACEMENT_3D('',#21389,#16960,#16961);
#15340=AXIS2_PLACEMENT_3D('',#21391,#16962,#16963);
#15341=AXIS2_PLACEMENT_3D('',#21393,#16964,#16965);
#15342=AXIS2_PLACEMENT_3D('',#21394,#16966,#16967);
#15343=AXIS2_PLACEMENT_3D('',#21395,#16968,#16969);
#15344=AXIS2_PLACEMENT_3D('',#21398,#16971,#16972);
#15345=AXIS2_PLACEMENT_3D('',#21399,#16973,#16974);
#15346=AXIS2_PLACEMENT_3D('',#21401,#16975,#16976);
#15347=AXIS2_PLACEMENT_3D('',#21403,#16978,#16979);
#15348=AXIS2_PLACEMENT_3D('',#21405,#16980,#16981);
#15349=AXIS2_PLACEMENT_3D('',#21408,#16983,#16984);
#15350=AXIS2_PLACEMENT_3D('',#21409,#16985,#16986);
#15351=AXIS2_PLACEMENT_3D('',#21411,#16987,#16988);
#15352=AXIS2_PLACEMENT_3D('',#21414,#16990,#16991);
#15353=AXIS2_PLACEMENT_3D('',#21415,#16992,#16993);
#15354=AXIS2_PLACEMENT_3D('',#21417,#16994,#16995);
#15355=AXIS2_PLACEMENT_3D('',#21421,#16997,#16998);
#15356=AXIS2_PLACEMENT_3D('',#21445,#16999,#17000);
#15357=AXIS2_PLACEMENT_3D('',#21446,#17001,#17002);
#15358=AXIS2_PLACEMENT_3D('',#21449,#17003,#17004);
#15359=AXIS2_PLACEMENT_3D('',#21453,#17006,#17007);
#15360=AXIS2_PLACEMENT_3D('',#21455,#17009,#17010);
#15361=AXIS2_PLACEMENT_3D('',#21457,#17011,#17012);
#15362=AXIS2_PLACEMENT_3D('',#21459,#17013,#17014);
#15363=AXIS2_PLACEMENT_3D('',#21461,#17015,#17016);
#15364=AXIS2_PLACEMENT_3D('',#21463,#17017,#17018);
#15365=AXIS2_PLACEMENT_3D('',#21464,#17019,#17020);
#15366=AXIS2_PLACEMENT_3D('',#21465,#17021,#17022);
#15367=AXIS2_PLACEMENT_3D('',#21467,#17023,#17024);
#15368=AXIS2_PLACEMENT_3D('',#21470,#17026,#17027);
#15369=AXIS2_PLACEMENT_3D('',#21471,#17028,#17029);
#15370=AXIS2_PLACEMENT_3D('',#21473,#17030,#17031);
#15371=AXIS2_PLACEMENT_3D('',#21476,#17033,#17034);
#15372=AXIS2_PLACEMENT_3D('',#21477,#17035,#17036);
#15373=AXIS2_PLACEMENT_3D('',#21478,#17037,#17038);
#15374=AXIS2_PLACEMENT_3D('',#21480,#17039,#17040);
#15375=AXIS2_PLACEMENT_3D('',#21483,#17042,#17043);
#15376=AXIS2_PLACEMENT_3D('',#21484,#17044,#17045);
#15377=AXIS2_PLACEMENT_3D('',#21487,#17047,#17048);
#15378=AXIS2_PLACEMENT_3D('',#21488,#17049,#17050);
#15379=AXIS2_PLACEMENT_3D('',#21490,#17051,#17052);
#15380=AXIS2_PLACEMENT_3D('',#21493,#17054,#17055);
#15381=AXIS2_PLACEMENT_3D('',#21494,#17056,#17057);
#15382=AXIS2_PLACEMENT_3D('',#21496,#17058,#17059);
#15383=AXIS2_PLACEMENT_3D('',#21499,#17061,#17062);
#15384=AXIS2_PLACEMENT_3D('',#21500,#17063,#17064);
#15385=AXIS2_PLACEMENT_3D('',#21502,#17065,#17066);
#15386=AXIS2_PLACEMENT_3D('',#21505,#17068,#17069);
#15387=AXIS2_PLACEMENT_3D('',#21506,#17070,#17071);
#15388=AXIS2_PLACEMENT_3D('',#21508,#17072,#17073);
#15389=AXIS2_PLACEMENT_3D('',#21510,#17074,#17075);
#15390=AXIS2_PLACEMENT_3D('',#21511,#17076,#17077);
#15391=AXIS2_PLACEMENT_3D('',#21512,#17078,#17079);
#15392=AXIS2_PLACEMENT_3D('',#21514,#17080,#17081);
#15393=AXIS2_PLACEMENT_3D('',#21517,#17083,#17084);
#15394=AXIS2_PLACEMENT_3D('',#21518,#17085,#17086);
#15395=AXIS2_PLACEMENT_3D('',#21520,#17087,#17088);
#15396=AXIS2_PLACEMENT_3D('',#21522,#17090,#17091);
#15397=AXIS2_PLACEMENT_3D('',#21524,#17092,#17093);
#15398=AXIS2_PLACEMENT_3D('',#21527,#17095,#17096);
#15399=AXIS2_PLACEMENT_3D('',#21528,#17097,#17098);
#15400=AXIS2_PLACEMENT_3D('',#21529,#17099,#17100);
#15401=AXIS2_PLACEMENT_3D('',#21530,#17101,#17102);
#15402=AXIS2_PLACEMENT_3D('',#21531,#17103,#17104);
#15403=AXIS2_PLACEMENT_3D('',#21532,#17105,#17106);
#15404=AXIS2_PLACEMENT_3D('',#21533,#17107,#17108);
#15405=AXIS2_PLACEMENT_3D('',#21542,#17113,#17114);
#15406=AXIS2_PLACEMENT_3D('',#21548,#17118,#17119);
#15407=AXIS2_PLACEMENT_3D('',#21552,#17122,#17123);
#15408=AXIS2_PLACEMENT_3D('',#21556,#17126,#17127);
#15409=AXIS2_PLACEMENT_3D('',#21565,#17132,#17133);
#15410=AXIS2_PLACEMENT_3D('',#21573,#17138,#17139);
#15411=AXIS2_PLACEMENT_3D('',#21577,#17142,#17143);
#15412=AXIS2_PLACEMENT_3D('',#21586,#17148,#17149);
#15413=AXIS2_PLACEMENT_3D('',#21592,#17153,#17154);
#15414=AXIS2_PLACEMENT_3D('',#21598,#17158,#17159);
#15415=AXIS2_PLACEMENT_3D('',#21604,#17163,#17164);
#15416=AXIS2_PLACEMENT_3D('',#21608,#17167,#17168);
#15417=AXIS2_PLACEMENT_3D('',#21611,#17171,#17172);
#15418=AXIS2_PLACEMENT_3D('',#21618,#17177,#17178);
#15419=AXIS2_PLACEMENT_3D('',#21620,#17180,#17181);
#15420=AXIS2_PLACEMENT_3D('',#21626,#17185,#17186);
#15421=AXIS2_PLACEMENT_3D('',#21630,#17189,#17190);
#15422=AXIS2_PLACEMENT_3D('',#21634,#17193,#17194);
#15423=AXIS2_PLACEMENT_3D('',#21636,#17196,#17197);
#15424=AXIS2_PLACEMENT_3D('',#21637,#17198,#17199);
#15425=AXIS2_PLACEMENT_3D('',#21646,#17204,#17205);
#15426=AXIS2_PLACEMENT_3D('',#21655,#17210,#17211);
#15427=AXIS2_PLACEMENT_3D('',#21665,#17217,#17218);
#15428=AXIS2_PLACEMENT_3D('',#21667,#17220,#17221);
#15429=AXIS2_PLACEMENT_3D('',#21673,#17225,#17226);
#15430=AXIS2_PLACEMENT_3D('',#21679,#17230,#17231);
#15431=AXIS2_PLACEMENT_3D('',#21684,#17235,#17236);
#15432=AXIS2_PLACEMENT_3D('',#21689,#17240,#17241);
#15433=AXIS2_PLACEMENT_3D('',#21693,#17244,#17245);
#15434=AXIS2_PLACEMENT_3D('',#21696,#17248,#17249);
#15435=AXIS2_PLACEMENT_3D('',#21698,#17251,#17252);
#15436=AXIS2_PLACEMENT_3D('',#21704,#17256,#17257);
#15437=AXIS2_PLACEMENT_3D('',#21707,#17260,#17261);
#15438=AXIS2_PLACEMENT_3D('',#21710,#17264,#17265);
#15439=AXIS2_PLACEMENT_3D('',#21712,#17267,#17268);
#15440=AXIS2_PLACEMENT_3D('',#21714,#17270,#17271);
#15441=AXIS2_PLACEMENT_3D('',#21715,#17272,#17273);
#15442=AXIS2_PLACEMENT_3D('',#27767,#17274,#17275);
#15443=AXIS2_PLACEMENT_3D('',#27790,#17276,#17277);
#15444=AXIS2_PLACEMENT_3D('',#27791,#17278,#17279);
#15445=AXIS2_PLACEMENT_3D('',#33842,#17280,#17281);
#15446=AXIS2_PLACEMENT_3D('',#33845,#17282,#17283);
#15447=AXIS2_PLACEMENT_3D('',#33849,#17285,#17286);
#15448=AXIS2_PLACEMENT_3D('',#33851,#17288,#17289);
#15449=AXIS2_PLACEMENT_3D('',#33857,#17293,#17294);
#15450=AXIS2_PLACEMENT_3D('',#33859,#17295,#17296);
#15451=AXIS2_PLACEMENT_3D('',#33861,#17297,#17298);
#15452=AXIS2_PLACEMENT_3D('',#33863,#17300,#17301);
#15453=AXIS2_PLACEMENT_3D('',#33864,#17302,#17303);
#15454=AXIS2_PLACEMENT_3D('',#33873,#17308,#17309);
#15455=AXIS2_PLACEMENT_3D('',#33876,#17312,#17313);
#15456=AXIS2_PLACEMENT_3D('',#33879,#17316,#17317);
#15457=AXIS2_PLACEMENT_3D('',#33880,#17318,#17319);
#15458=AXIS2_PLACEMENT_3D('',#33883,#17322,#17323);
#15459=AXIS2_PLACEMENT_3D('',#33884,#17324,#17325);
#15460=AXIS2_PLACEMENT_3D('',#33885,#17326,#17327);
#15461=AXIS2_PLACEMENT_3D('',#33886,#17328,#17329);
#15462=AXIS2_PLACEMENT_3D('',#33887,#17330,#17331);
#15463=AXIS2_PLACEMENT_3D('',#33888,#17332,#17333);
#15464=AXIS2_PLACEMENT_3D('',#33897,#17338,#17339);
#15465=AXIS2_PLACEMENT_3D('',#33903,#17343,#17344);
#15466=AXIS2_PLACEMENT_3D('',#33907,#17347,#17348);
#15467=AXIS2_PLACEMENT_3D('',#33908,#17349,#17350);
#15468=AXIS2_PLACEMENT_3D('',#33912,#17353,#17354);
#15469=AXIS2_PLACEMENT_3D('',#33914,#17356,#17357);
#15470=AXIS2_PLACEMENT_3D('',#33915,#17358,#17359);
#16958=DIRECTION('axis',(0.,0.,1.));
#16959=DIRECTION('refdir',(1.,0.,0.));
#16960=DIRECTION('center_axis',(-0.430981504924197,-0.768119965562791,0.473546894105632));
#16961=DIRECTION('ref_axis',(-0.513559013416071,0.640299002836773,0.571204277562193));
#16962=DIRECTION('center_axis',(0.430981504924197,0.768119965562791,-0.473546894105632));
#16963=DIRECTION('ref_axis',(0.51355901341607,-0.640299002836773,-0.571204277562193));
#16964=DIRECTION('center_axis',(-0.741965014102678,0.00298420341975994,
-0.670431959543668));
#16965=DIRECTION('ref_axis',(0.51355901341607,-0.640299002836773,-0.571204277562193));
#16966=DIRECTION('center_axis',(-0.430981504924197,-0.768119965562791,0.473546894105632));
#16967=DIRECTION('ref_axis',(-0.51355901341607,0.640299002836773,0.571204277562193));
#16968=DIRECTION('center_axis',(0.430981504924197,0.768119965562791,-0.473546894105632));
#16969=DIRECTION('ref_axis',(-0.51355901341607,0.640299002836773,0.571204277562193));
#16970=DIRECTION('',(-0.430981504924197,-0.768119965562791,0.473546894105632));
#16971=DIRECTION('center_axis',(0.430981504924197,0.768119965562791,-0.473546894105632));
#16972=DIRECTION('ref_axis',(0.51355901341607,-0.640299002836773,-0.571204277562193));
#16973=DIRECTION('center_axis',(0.430981504924197,0.768119965562791,-0.473546894105632));
#16974=DIRECTION('ref_axis',(-0.51355901341607,0.640299002836773,0.571204277562193));
#16975=DIRECTION('center_axis',(-0.430981504924197,-0.768119965562791,0.473546894105632));
#16976=DIRECTION('ref_axis',(-0.51355901341607,0.640299002836773,0.571204277562193));
#16977=DIRECTION('',(-0.430981504924197,-0.768119965562791,0.473546894105632));
#16978=DIRECTION('center_axis',(0.430981504924197,0.768119965562791,-0.473546894105632));
#16979=DIRECTION('ref_axis',(-0.51355901341607,0.640299002836773,0.571204277562193));
#16980=DIRECTION('center_axis',(0.430981504924197,0.768119965562791,-0.473546894105632));
#16981=DIRECTION('ref_axis',(-0.51355901341607,0.640299002836773,0.571204277562193));
#16982=DIRECTION('',(0.430981504924197,0.768119965562791,-0.473546894105632));
#16983=DIRECTION('center_axis',(-0.430981504924197,-0.768119965562791,0.473546894105632));
#16984=DIRECTION('ref_axis',(0.51355901341607,-0.640299002836773,-0.571204277562193));
#16985=DIRECTION('center_axis',(0.741965014102678,-0.00298420341976004,
0.670431959543668));
#16986=DIRECTION('ref_axis',(0.51355901341607,-0.640299002836774,-0.571204277562193));
#16987=DIRECTION('center_axis',(0.741965014102678,-0.00298420341976,0.670431959543668));
#16988=DIRECTION('ref_axis',(0.51355901341607,-0.640299002836774,-0.571204277562193));
#16989=DIRECTION('',(0.741965014102678,-0.00298420341976004,0.670431959543668));
#16990=DIRECTION('center_axis',(0.741965014102678,-0.00298420341976,0.670431959543668));
#16991=DIRECTION('ref_axis',(0.51355901341607,-0.640299002836774,-0.571204277562193));
#16992=DIRECTION('center_axis',(0.430981504924197,0.768119965562791,-0.473546894105632));
#16993=DIRECTION('ref_axis',(0.51355901341607,-0.640299002836773,-0.571204277562193));
#16994=DIRECTION('center_axis',(-0.430981504924197,-0.768119965562791,0.473546894105632));
#16995=DIRECTION('ref_axis',(-0.51355901341607,0.640299002836773,0.571204277562193));
#16996=DIRECTION('',(-0.307737294542031,-0.889938771903478,0.336610665028428));
#16997=DIRECTION('center_axis',(-0.430981504924197,-0.768119965562791,0.473546894105632));
#16998=DIRECTION('ref_axis',(-0.51355901341607,0.640299002836773,0.571204277562193));
#16999=DIRECTION('center_axis',(-0.430981504924197,-0.768119965562791,0.473546894105632));
#17000=DIRECTION('ref_axis',(-0.51355901341607,0.640299002836773,0.571204277562193));
#17001=DIRECTION('center_axis',(-0.430981504924197,-0.768119965562791,0.473546894105632));
#17002=DIRECTION('ref_axis',(0.51355901341607,-0.640299002836773,-0.571204277562193));
#17003=DIRECTION('center_axis',(0.430981504924197,0.768119965562791,-0.473546894105632));
#17004=DIRECTION('ref_axis',(-0.51355901341607,0.640299002836773,0.571204277562193));
#17005=DIRECTION('',(0.430981504924197,0.768119965562791,-0.473546894105632));
#17006=DIRECTION('center_axis',(0.430981504924197,0.768119965562791,-0.473546894105632));
#17007=DIRECTION('ref_axis',(-0.51355901341607,0.640299002836773,0.571204277562193));
#17008=DIRECTION('',(0.430981504924197,0.768119965562791,-0.473546894105632));
#17009=DIRECTION('center_axis',(-0.430981504924197,-0.768119965562791,0.473546894105632));
#17010=DIRECTION('ref_axis',(0.741965014102678,-0.00298420341976045,0.670431959543668));
#17011=DIRECTION('center_axis',(0.829398437573064,0.541032685939668,0.139218764885589));
#17012=DIRECTION('ref_axis',(0.219898548181541,-0.545252986894079,0.808915204944706));
#17013=DIRECTION('center_axis',(0.219898548176702,-0.54525298688807,0.808915204950072));
#17014=DIRECTION('ref_axis',(-0.541205761680708,0.621711011172037,0.566190552827446));
#17015=DIRECTION('center_axis',(0.430981504924197,0.768119965562791,-0.473546894105632));
#17016=DIRECTION('ref_axis',(0.51355901341607,-0.640299002836773,-0.571204277562193));
#17017=DIRECTION('center_axis',(0.219898548178344,-0.545252986890155,0.80891520494822));
#17018=DIRECTION('ref_axis',(0.513561985737025,-0.64029706392645,-0.571203778640348));
#17019=DIRECTION('center_axis',(0.829398437573076,0.541032685939656,0.139218764885566));
#17020=DIRECTION('ref_axis',(0.219898548177576,-0.545252986889121,0.808915204949126));
#17021=DIRECTION('center_axis',(-0.741965014102678,0.00298420341976004,
-0.670431959543668));
#17022=DIRECTION('ref_axis',(-0.51355901341607,0.640299002836773,0.571204277562193));
#17023=DIRECTION('center_axis',(0.741965014102678,-0.00298420341976004,
0.670431959543668));
#17024=DIRECTION('ref_axis',(-0.51355901341607,0.640299002836773,0.571204277562193));
#17025=DIRECTION('',(0.741965014102678,-0.00298420341976004,0.670431959543668));
#17026=DIRECTION('center_axis',(-0.741965014102678,0.00298420341976,-0.670431959543668));
#17027=DIRECTION('ref_axis',(-0.430981504924197,-0.768119965562791,0.473546894105632));
#17028=DIRECTION('center_axis',(-0.741965014102678,0.00298420341976,-0.670431959543668));
#17029=DIRECTION('ref_axis',(0.430981504924197,0.768119965562791,-0.473546894105632));
#17030=DIRECTION('center_axis',(-0.741965014102678,0.00298420341976,-0.670431959543668));
#17031=DIRECTION('ref_axis',(-0.51355901341607,0.640299002836773,0.571204277562193));
#17032=DIRECTION('',(0.741965014102678,-0.00298420341976,0.670431959543668));
#17033=DIRECTION('center_axis',(0.219900418845594,-0.545253383109838,0.808914429342689));
#17034=DIRECTION('ref_axis',(0.829406037148494,0.541023543918342,0.139209017192382));
#17035=DIRECTION('center_axis',(0.219898716470999,-0.545251260610337,0.808916322803073));
#17036=DIRECTION('ref_axis',(0.829390297200403,0.541043168290232,0.139226523896475));
#17037=DIRECTION('center_axis',(-0.741965014102678,0.00298420341976004,
-0.670431959543668));
#17038=DIRECTION('ref_axis',(-0.51355901341607,0.640299002836773,0.571204277562193));
#17039=DIRECTION('center_axis',(0.741965014102678,-0.00298420341976004,
0.670431959543668));
#17040=DIRECTION('ref_axis',(-0.51355901341607,0.640299002836773,0.571204277562193));
#17041=DIRECTION('',(0.741965014102678,-0.00298420341976004,0.670431959543668));
#17042=DIRECTION('center_axis',(0.741965014102678,-0.00298420341976004,
0.670431959543668));
#17043=DIRECTION('ref_axis',(-0.51355901341607,0.640299002836773,0.571204277562193));
#17044=DIRECTION('center_axis',(0.741965014102678,-0.00298420341976004,
0.670431959543668));
#17045=DIRECTION('ref_axis',(-0.51355901341607,0.640299002836773,0.571204277562193));
#17046=DIRECTION('',(-0.902360417214314,0.367323754862617,-0.225430558173548));
#17047=DIRECTION('center_axis',(0.741965014102678,-0.00298420341976004,
0.670431959543668));
#17048=DIRECTION('ref_axis',(-0.51355901341607,0.640299002836773,0.571204277562193));
#17049=DIRECTION('center_axis',(-0.430981504924197,-0.768119965562791,0.473546894105632));
#17050=DIRECTION('ref_axis',(0.513559013416073,-0.640299002836773,-0.57120427756219));
#17051=DIRECTION('center_axis',(-0.430981504924197,-0.768119965562791,0.473546894105632));
#17052=DIRECTION('ref_axis',(-0.513559013416073,0.640299002836773,0.57120427756219));
#17053=DIRECTION('',(-0.430981504924197,-0.768119965562791,0.473546894105632));
#17054=DIRECTION('center_axis',(-0.430981504924197,-0.768119965562791,0.473546894105632));
#17055=DIRECTION('ref_axis',(-0.513559013416073,0.640299002836773,0.57120427756219));
#17056=DIRECTION('center_axis',(-0.430981504924197,-0.768119965562791,0.473546894105632));
#17057=DIRECTION('ref_axis',(0.513559013416073,-0.640299002836773,-0.57120427756219));
#17058=DIRECTION('center_axis',(0.430981504924197,0.768119965562791,-0.473546894105632));
#17059=DIRECTION('ref_axis',(-0.513559013416073,0.640299002836773,0.57120427756219));
#17060=DIRECTION('',(-0.430981504924197,-0.768119965562791,0.473546894105632));
#17061=DIRECTION('center_axis',(0.430981504924197,0.768119965562791,-0.473546894105632));
#17062=DIRECTION('ref_axis',(-0.513559013416073,0.640299002836773,0.57120427756219));
#17063=DIRECTION('center_axis',(0.430981504924197,0.768119965562791,-0.473546894105632));
#17064=DIRECTION('ref_axis',(-0.51355901341607,0.640299002836773,0.571204277562193));
#17065=DIRECTION('center_axis',(-0.430981504924197,-0.768119965562791,0.473546894105632));
#17066=DIRECTION('ref_axis',(-0.51355901341607,0.640299002836773,0.571204277562193));
#17067=DIRECTION('',(0.430981504924197,0.768119965562791,-0.473546894105632));
#17068=DIRECTION('center_axis',(-0.430981504924197,-0.768119965562791,0.473546894105632));
#17069=DIRECTION('ref_axis',(-0.51355901341607,0.640299002836773,0.571204277562193));
#17070=DIRECTION('center_axis',(-0.430981504924197,-0.768119965562791,0.473546894105632));
#17071=DIRECTION('ref_axis',(-0.51355901341607,0.640299002836774,0.571204277562193));
#17072=DIRECTION('center_axis',(-0.430981504924197,-0.768119965562791,0.473546894105632));
#17073=DIRECTION('ref_axis',(-0.51355901341607,0.640299002836773,0.571204277562193));
#17074=DIRECTION('center_axis',(0.741965014102678,-0.00298420341976022,
0.670431959543668));
#17075=DIRECTION('ref_axis',(0.51355901341607,-0.640299002836773,-0.571204277562193));
#17076=DIRECTION('center_axis',(-0.430981504924197,-0.768119965562791,0.473546894105632));
#17077=DIRECTION('ref_axis',(-0.51355901341607,0.640299002836773,0.571204277562193));
#17078=DIRECTION('center_axis',(0.430981504924197,0.768119965562791,-0.473546894105632));
#17079=DIRECTION('ref_axis',(-0.51355901341607,0.640299002836773,0.571204277562193));
#17080=DIRECTION('center_axis',(-0.430981504924197,-0.768119965562791,0.473546894105632));
#17081=DIRECTION('ref_axis',(-0.51355901341607,0.640299002836773,0.571204277562193));
#17082=DIRECTION('',(-0.430981504924197,-0.768119965562791,0.473546894105632));
#17083=DIRECTION('center_axis',(-0.430981504924197,-0.768119965562791,0.473546894105632));
#17084=DIRECTION('ref_axis',(-0.51355901341607,0.640299002836773,0.571204277562193));
#17085=DIRECTION('center_axis',(-0.430981504924197,-0.768119965562791,0.473546894105632));
#17086=DIRECTION('ref_axis',(-0.51355901341607,0.640299002836773,0.571204277562193));
#17087=DIRECTION('center_axis',(-0.430981504924197,-0.768119965562791,0.473546894105632));
#17088=DIRECTION('ref_axis',(-0.51355901341607,0.640299002836773,0.571204277562193));
#17089=DIRECTION('',(-0.0583911162280923,0.995902603307094,0.0690541980750679));
#17090=DIRECTION('center_axis',(0.430981504924197,0.768119965562791,-0.473546894105632));
#17091=DIRECTION('ref_axis',(-0.51355901341607,0.640299002836773,0.571204277562193));
#17092=DIRECTION('center_axis',(-0.430981504924197,-0.768119965562791,0.473546894105632));
#17093=DIRECTION('ref_axis',(-0.51355901341607,0.640299002836773,0.571204277562193));
#17094=DIRECTION('',(0.430981504924197,0.768119965562791,-0.473546894105632));
#17095=DIRECTION('center_axis',(-0.430981504924197,-0.768119965562791,0.473546894105632));
#17096=DIRECTION('ref_axis',(-0.51355901341607,0.640299002836773,0.571204277562193));
#17097=DIRECTION('center_axis',(-0.430981504924197,-0.768119965562791,0.473546894105632));
#17098=DIRECTION('ref_axis',(-0.51355901341607,0.640299002836773,0.571204277562193));
#17099=DIRECTION('center_axis',(0.430981504924197,0.768119965562791,-0.473546894105632));
#17100=DIRECTION('ref_axis',(0.741965014102678,-0.00298420341976002,0.670431959543668));
#17101=DIRECTION('center_axis',(-0.430981504924197,-0.768119965562791,0.473546894105632));
#17102=DIRECTION('ref_axis',(-0.51355901341607,0.640299002836773,0.571204277562193));
#17103=DIRECTION('center_axis',(0.430981504924197,0.768119965562791,-0.473546894105632));
#17104=DIRECTION('ref_axis',(0.741965014102678,-0.00298420341976002,0.670431959543668));
#17105=DIRECTION('center_axis',(-0.430981504924197,-0.768119965562791,0.473546894105632));
#17106=DIRECTION('ref_axis',(-0.51355901341607,0.640299002836773,0.571204277562193));
#17107=DIRECTION('center_axis',(-0.741965014102678,0.00298420341976008,
-0.670431959543668));
#17108=DIRECTION('ref_axis',(-0.51355901341607,0.640299002836773,0.571204277562193));
#17109=DIRECTION('',(-0.430981504924197,-0.768119965562791,0.473546894105632));
#17110=DIRECTION('',(0.51355901341607,-0.640299002836773,-0.571204277562193));
#17111=DIRECTION('',(0.430981504924197,0.768119965562791,-0.473546894105632));
#17112=DIRECTION('',(-0.51355901341607,0.640299002836773,0.571204277562193));
#17113=DIRECTION('center_axis',(0.430981504924197,0.768119965562791,-0.473546894105632));
#17114=DIRECTION('ref_axis',(0.741965014102678,-0.00298420341976002,0.670431959543668));
#17115=DIRECTION('',(0.51355901341607,-0.640299002836773,-0.571204277562193));
#17116=DIRECTION('',(-0.741965014102678,0.00298420341976,-0.670431959543668));
#17117=DIRECTION('',(-0.741965014102678,0.00298420341976,-0.670431959543668));
#17118=DIRECTION('center_axis',(-0.51355901341607,0.640299002836773,0.571204277562193));
#17119=DIRECTION('ref_axis',(-0.741965014102678,0.00298420341975993,-0.670431959543668));
#17120=DIRECTION('',(0.430981504924197,0.768119965562791,-0.473546894105632));
#17121=DIRECTION('',(-0.741965014102678,0.00298420341976,-0.670431959543668));
#17122=DIRECTION('center_axis',(-0.430981504924197,-0.768119965562791,0.473546894105632));
#17123=DIRECTION('ref_axis',(-0.51355901341607,0.640299002836773,0.571204277562193));
#17124=DIRECTION('',(-0.51355901341607,0.640299002836773,0.571204277562193));
#17125=DIRECTION('',(-0.741965014102678,0.00298420341976,-0.670431959543668));
#17126=DIRECTION('center_axis',(-0.741965014102678,0.00298420341976008,
-0.670431959543668));
#17127=DIRECTION('ref_axis',(-0.51355901341607,0.640299002836773,0.571204277562193));
#17128=DIRECTION('',(-0.430981504924197,-0.768119965562791,0.473546894105632));
#17129=DIRECTION('',(0.51355901341607,-0.640299002836773,-0.571204277562193));
#17130=DIRECTION('',(0.430981504924197,0.768119965562791,-0.473546894105632));
#17131=DIRECTION('',(-0.51355901341607,0.640299002836773,0.571204277562193));
#17132=DIRECTION('center_axis',(-0.51355901341607,0.640299002836773,0.571204277562193));
#17133=DIRECTION('ref_axis',(0.430981504924197,0.768119965562791,-0.473546894105632));
#17134=DIRECTION('',(0.430981504924197,0.768119965562791,-0.473546894105632));
#17135=DIRECTION('',(0.219898548177292,-0.545252986888779,0.808915204949433));
#17136=DIRECTION('',(-0.741965014102678,0.00298420341976,-0.670431959543668));
#17137=DIRECTION('',(-0.741965014102678,0.00298420341976,-0.670431959543668));
#17138=DIRECTION('center_axis',(-0.430981504924197,-0.768119965562791,0.473546894105632));
#17139=DIRECTION('ref_axis',(-0.51355901341607,0.640299002836773,0.571204277562193));
#17140=DIRECTION('',(0.51355901341607,-0.640299002836773,-0.571204277562193));
#17141=DIRECTION('',(-0.741965014102678,0.00298420341976,-0.670431959543668));
#17142=DIRECTION('center_axis',(0.51355901341607,-0.640299002836773,-0.571204277562193));
#17143=DIRECTION('ref_axis',(-0.430981504924197,-0.768119965562791,0.473546894105632));
#17144=DIRECTION('',(-0.741965014102678,0.00298420341976,-0.670431959543668));
#17145=DIRECTION('',(-0.430981504924197,-0.768119965562791,0.473546894105632));
#17146=DIRECTION('',(-0.741965014102678,0.00298420341976,-0.670431959543668));
#17147=DIRECTION('',(-0.430981504924197,-0.768119965562791,0.473546894105632));
#17148=DIRECTION('center_axis',(0.430981504924197,0.768119965562791,-0.473546894105632));
#17149=DIRECTION('ref_axis',(0.741965014102678,-0.00298420341976002,0.670431959543668));
#17150=DIRECTION('',(-0.741965014102678,0.00298420341976,-0.670431959543668));
#17151=DIRECTION('',(0.51355901341607,-0.640299002836773,-0.571204277562193));
#17152=DIRECTION('',(0.51355901341607,-0.640299002836773,-0.571204277562193));
#17153=DIRECTION('center_axis',(-0.51355901341607,0.640299002836773,0.571204277562193));
#17154=DIRECTION('ref_axis',(-0.741965014102678,0.00298420341975993,-0.670431959543668));
#17155=DIRECTION('',(-0.741965014102678,0.00298420341976,-0.670431959543668));
#17156=DIRECTION('',(0.430981504924197,0.768119965562791,-0.473546894105632));
#17157=DIRECTION('',(0.430981504924197,0.768119965562791,-0.473546894105632));
#17158=DIRECTION('center_axis',(-0.164240744208196,0.580034296524335,-0.79786289097655));
#17159=DIRECTION('ref_axis',(0.51355901341607,-0.640299002836773,-0.571204277562193));
#17160=DIRECTION('',(-0.981729594100533,-0.0173310113105418,0.18949047499586));
#17161=DIRECTION('',(-0.51355901341607,0.640299002836773,0.571204277562193));
#17162=DIRECTION('',(-0.364106245973748,-0.787376134856833,-0.497459007256696));
#17163=DIRECTION('center_axis',(-0.1615074319492,-0.450649616418314,-0.877969403024502));
#17164=DIRECTION('ref_axis',(-0.430981504924197,-0.768119965562791,0.473546894105632));
#17165=DIRECTION('',(-0.528205843253997,0.790965038292377,-0.308825023842745));
#17166=DIRECTION('',(0.430981504924197,0.768119965562791,-0.473546894105632));
#17167=DIRECTION('center_axis',(-0.430981504924197,-0.768119965562791,0.473546894105632));
#17168=DIRECTION('ref_axis',(-0.51355901341607,0.640299002836773,0.571204277562193));
#17169=DIRECTION('',(-0.51355901341607,0.640299002836773,0.571204277562193));
#17170=DIRECTION('',(-0.51355901341607,0.640299002836773,0.571204277562193));
#17171=DIRECTION('center_axis',(-0.812934017119492,-0.576104073118877,-0.0851021782671007));
#17172=DIRECTION('ref_axis',(-0.51355901341607,0.640299002836773,0.571204277562193));
#17173=DIRECTION('',(0.51355901341607,-0.640299002836773,-0.571204277562193));
#17174=DIRECTION('',(-0.51355901341607,0.640299002836773,0.571204277562193));
#17175=DIRECTION('',(0.51355901341607,-0.640299002836773,-0.571204277562193));
#17176=DIRECTION('',(0.0894175048727878,0.0209199147460851,-0.995774506095301));
#17177=DIRECTION('center_axis',(-0.887789553801152,0.454869917367419,-0.0701645668105232));
#17178=DIRECTION('ref_axis',(0.430981504924197,0.768119965562791,-0.473546894105632));
#17179=DIRECTION('',(-0.430981504924197,-0.768119965562791,0.473546894105632));
#17180=DIRECTION('center_axis',(-0.430981504924197,-0.768119965562791,0.473546894105632));
#17181=DIRECTION('ref_axis',(-0.51355901341607,0.640299002836773,0.571204277562193));
#17182=DIRECTION('',(-0.51355901341607,0.640299002836773,0.571204277562193));
#17183=DIRECTION('',(-0.741965014102678,0.00298420341976007,-0.670431959543668));
#17184=DIRECTION('',(-0.741965014102678,0.00298420341976007,-0.670431959543668));
#17185=DIRECTION('center_axis',(-0.51355901341607,0.640299002836773,0.571204277562193));
#17186=DIRECTION('ref_axis',(0.741965014102678,-0.00298420341976001,0.670431959543668));
#17187=DIRECTION('',(0.430981504924197,0.768119965562791,-0.473546894105632));
#17188=DIRECTION('',(-0.741965014102678,0.00298420341976007,-0.670431959543668));
#17189=DIRECTION('center_axis',(0.430981504924197,0.768119965562791,-0.473546894105632));
#17190=DIRECTION('ref_axis',(0.741965014102678,-0.00298420341976002,0.670431959543668));
#17191=DIRECTION('',(0.51355901341607,-0.640299002836773,-0.571204277562193));
#17192=DIRECTION('',(-0.741965014102678,0.00298420341976007,-0.670431959543668));
#17193=DIRECTION('center_axis',(0.51355901341607,-0.640299002836773,-0.571204277562193));
#17194=DIRECTION('ref_axis',(-0.430981504924197,-0.768119965562791,0.473546894105632));
#17195=DIRECTION('',(-0.430981504924197,-0.768119965562791,0.473546894105632));
#17196=DIRECTION('center_axis',(0.741965014102678,-0.00298420341976011,
0.670431959543668));
#17197=DIRECTION('ref_axis',(0.51355901341607,-0.640299002836773,-0.571204277562193));
#17198=DIRECTION('center_axis',(-0.741965014102678,0.00298420341976008,
-0.670431959543668));
#17199=DIRECTION('ref_axis',(-0.51355901341607,0.640299002836773,0.571204277562193));
#17200=DIRECTION('',(0.51355901341607,-0.640299002836773,-0.571204277562193));
#17201=DIRECTION('',(0.430981504924197,0.768119965562791,-0.473546894105632));
#17202=DIRECTION('',(-0.51355901341607,0.640299002836773,0.571204277562193));
#17203=DIRECTION('',(-0.430981504924197,-0.768119965562791,0.473546894105632));
#17204=DIRECTION('center_axis',(-0.430981504924197,-0.768119965562791,0.473546894105632));
#17205=DIRECTION('ref_axis',(-0.51355901341607,0.640299002836773,0.571204277562193));
#17206=DIRECTION('',(0.741965014102678,-0.00298420341976,0.670431959543668));
#17207=DIRECTION('',(0.51355901341607,-0.640299002836773,-0.571204277562193));
#17208=DIRECTION('',(0.741965014102678,-0.00298420341976,0.670431959543668));
#17209=DIRECTION('',(0.51355901341607,-0.640299002836773,-0.571204277562193));
#17210=DIRECTION('center_axis',(0.51355901341607,-0.640299002836773,-0.571204277562193));
#17211=DIRECTION('ref_axis',(-0.430981504924197,-0.768119965562791,0.473546894105632));
#17212=DIRECTION('',(0.219898548177293,-0.545252986888779,0.808915204949433));
#17213=DIRECTION('',(0.430981504924197,0.768119965562791,-0.473546894105632));
#17214=DIRECTION('',(-0.829398437573059,-0.541032685939674,-0.139218764885593));
#17215=DIRECTION('',(0.741965014102678,-0.00298420341976,0.670431959543668));
#17216=DIRECTION('',(0.430981504924197,0.768119965562791,-0.473546894105632));
#17217=DIRECTION('center_axis',(0.51355901341607,-0.640299002836773,-0.571204277562193));
#17218=DIRECTION('ref_axis',(-0.430981504924197,-0.768119965562791,0.473546894105632));
#17219=DIRECTION('',(-0.430981504924197,-0.768119965562791,0.473546894105632));
#17220=DIRECTION('center_axis',(-0.1615074319492,-0.450649616418314,-0.877969403024502));
#17221=DIRECTION('ref_axis',(-0.430981504924197,-0.768119965562791,0.473546894105632));
#17222=DIRECTION('',(-0.476049847378258,0.814874001184978,-0.330691555688864));
#17223=DIRECTION('',(-0.430981504924197,-0.768119965562791,0.473546894105632));
#17224=DIRECTION('',(0.973704423145728,0.0720745365902279,-0.21611329788273));
#17225=DIRECTION('center_axis',(0.430981504924197,0.768119965562791,-0.473546894105632));
#17226=DIRECTION('ref_axis',(0.741965014102678,-0.00298420341976002,0.670431959543668));
#17227=DIRECTION('',(-0.51355901341607,0.640299002836773,0.571204277562193));
#17228=DIRECTION('',(0.741965014102678,-0.00298420341976,0.670431959543668));
#17229=DIRECTION('',(-0.51355901341607,0.640299002836773,0.571204277562193));
#17230=DIRECTION('center_axis',(-0.829398437573059,-0.541032685939675,-0.139218764885592));
#17231=DIRECTION('ref_axis',(-0.51355901341607,0.640299002836773,0.571204277562193));
#17232=DIRECTION('',(-0.219898548177293,0.545252986888779,-0.808915204949433));
#17233=DIRECTION('',(-0.116957021902796,-0.0755203978856573,0.990261442514461));
#17234=DIRECTION('',(0.51355901341607,-0.640299002836773,-0.571204277562193));
#17235=DIRECTION('center_axis',(-0.219898548177292,0.54525298688878,-0.808915204949433));
#17236=DIRECTION('ref_axis',(0.51355901341607,-0.640299002836773,-0.571204277562193));
#17237=DIRECTION('',(-0.51355901341607,0.640299002836773,0.571204277562193));
#17238=DIRECTION('',(-0.380697553864674,-0.811428139889548,-0.443456588942866));
#17239=DIRECTION('',(0.829398437573059,0.541032685939674,0.139218764885593));
#17240=DIRECTION('center_axis',(-0.741965014102678,0.00298420341976008,
-0.670431959543668));
#17241=DIRECTION('ref_axis',(-0.51355901341607,0.640299002836773,0.571204277562193));
#17242=DIRECTION('',(-0.430981504924197,-0.768119965562791,0.473546894105632));
#17243=DIRECTION('',(-0.51355901341607,0.640299002836773,0.571204277562193));
#17244=DIRECTION('center_axis',(-0.51355901341607,0.640299002836773,0.571204277562193));
#17245=DIRECTION('ref_axis',(-0.741965014102678,0.00298420341975993,-0.670431959543668));
#17246=DIRECTION('',(-0.430981504924197,-0.768119965562791,0.473546894105632));
#17247=DIRECTION('',(-0.430981504924197,-0.768119965562791,0.473546894105632));
#17248=DIRECTION('center_axis',(0.829398437573059,0.541032685939674,0.139218764885593));
#17249=DIRECTION('ref_axis',(-0.219898548177292,0.54525298688878,-0.808915204949433));
#17250=DIRECTION('',(-0.219898548177292,0.54525298688878,-0.808915204949433));
#17251=DIRECTION('center_axis',(-0.741965014102678,0.00298420341976008,
-0.670431959543668));
#17252=DIRECTION('ref_axis',(-0.51355901341607,0.640299002836773,0.571204277562193));
#17253=DIRECTION('',(-0.51355901341607,0.640299002836773,0.571204277562193));
#17254=DIRECTION('',(0.51355901341607,-0.640299002836773,-0.571204277562193));
#17255=DIRECTION('',(0.430981504924197,0.768119965562791,-0.473546894105632));
#17256=DIRECTION('center_axis',(0.887789553801152,-0.454869917367419,0.0701645668105237));
#17257=DIRECTION('ref_axis',(-0.161507431949199,-0.450649616418315,-0.877969403024502));
#17258=DIRECTION('',(0.116957021902797,0.0755203978856587,-0.990261442514461));
#17259=DIRECTION('',(0.380697553864674,0.811428139889549,0.443456588942865));
#17260=DIRECTION('center_axis',(0.219898548177294,-0.545252986888779,0.808915204949433));
#17261=DIRECTION('ref_axis',(0.51355901341607,-0.640299002836773,-0.571204277562193));
#17262=DIRECTION('',(0.973704423145727,0.0720745365902286,-0.216113297882731));
#17263=DIRECTION('',(-0.51355901341607,0.640299002836773,0.571204277562193));
#17264=DIRECTION('center_axis',(0.829398437573059,0.541032685939674,0.139218764885593));
#17265=DIRECTION('ref_axis',(-0.219898548177292,0.54525298688878,-0.808915204949433));
#17266=DIRECTION('',(-0.476049847378257,0.814874001184979,-0.330691555688864));
#17267=DIRECTION('center_axis',(0.51355901341607,-0.640299002836773,-0.571204277562193));
#17268=DIRECTION('ref_axis',(-0.430981504924197,-0.768119965562791,0.473546894105632));
#17269=DIRECTION('',(-0.741965014102678,0.00298420341976,-0.670431959543668));
#17270=DIRECTION('center_axis',(0.1615074319492,0.450649616418314,0.877969403024502));
#17271=DIRECTION('ref_axis',(0.430981504924197,0.768119965562791,-0.473546894105632));
#17272=DIRECTION('center_axis',(-0.741965014102678,0.00298420341976008,
-0.670431959543668));
#17273=DIRECTION('ref_axis',(-0.51355901341607,0.640299002836773,0.571204277562193));
#17274=DIRECTION('center_axis',(0.765578497613709,-0.033471246755464,0.642471197511742));
#17275=DIRECTION('ref_axis',(0.477644749164911,-0.63943052331309,-0.602481617521014));
#17276=DIRECTION('center_axis',(-0.716668115383597,-0.0275096106575757,
-0.69687160489863));
#17277=DIRECTION('ref_axis',(0.548308083841373,-0.639714733162591,-0.538630954707318));
#17278=DIRECTION('center_axis',(-0.430981504924197,-0.768119965562791,0.473546894105632));
#17279=DIRECTION('ref_axis',(0.513559013416073,-0.640299002836773,-0.57120427756219));
#17280=DIRECTION('center_axis',(-0.430981504924197,-0.768119965562791,0.473546894105632));
#17281=DIRECTION('ref_axis',(-0.513559013416071,0.640299002836773,0.571204277562192));
#17282=DIRECTION('center_axis',(0.430981504924197,0.768119965562791,-0.473546894105632));
#17283=DIRECTION('ref_axis',(0.51355901341607,-0.640299002836773,-0.571204277562193));
#17284=DIRECTION('',(0.430981504924197,0.768119965562791,-0.473546894105632));
#17285=DIRECTION('center_axis',(0.430981504924197,0.768119965562791,-0.473546894105632));
#17286=DIRECTION('ref_axis',(0.513559013416071,-0.640299002836773,-0.571204277562193));
#17287=DIRECTION('',(0.430981504924197,0.768119965562791,-0.473546894105632));
#17288=DIRECTION('center_axis',(0.741965014102679,-0.00298420341976144,
0.670431959543667));
#17289=DIRECTION('ref_axis',(0.513559013416068,-0.640299002836773,-0.571204277562195));
#17290=DIRECTION('',(0.513559013416069,-0.640299002836773,-0.571204277562194));
#17291=DIRECTION('',(0.513559013416069,-0.640299002836773,-0.571204277562194));
#17292=DIRECTION('',(0.430981504924197,0.768119965562791,-0.473546894105632));
#17293=DIRECTION('center_axis',(-0.430981504924197,-0.768119965562791,0.473546894105632));
#17294=DIRECTION('ref_axis',(0.51355901341607,-0.640299002836773,-0.571204277562193));
#17295=DIRECTION('center_axis',(0.430981504924197,0.768119965562791,-0.473546894105632));
#17296=DIRECTION('ref_axis',(-0.51355901341607,0.640299002836773,0.571204277562193));
#17297=DIRECTION('center_axis',(0.430981504924197,0.768119965562791,-0.473546894105632));
#17298=DIRECTION('ref_axis',(-0.51355901341607,0.640299002836773,0.571204277562193));
#17299=DIRECTION('',(0.430981504924197,0.768119965562791,-0.473546894105632));
#17300=DIRECTION('center_axis',(-0.430981504924197,-0.768119965562791,0.473546894105632));
#17301=DIRECTION('ref_axis',(-0.51355901341607,0.640299002836773,0.571204277562193));
#17302=DIRECTION('center_axis',(0.741965014102678,-0.00298420341976019,
0.670431959543668));
#17303=DIRECTION('ref_axis',(0.51355901341607,-0.640299002836773,-0.571204277562193));
#17304=DIRECTION('',(0.51355901341607,-0.640299002836773,-0.571204277562193));
#17305=DIRECTION('',(0.430981504924197,0.768119965562791,-0.473546894105632));
#17306=DIRECTION('',(0.51355901341607,-0.640299002836773,-0.571204277562193));
#17307=DIRECTION('',(0.430981504924197,0.768119965562791,-0.473546894105632));
#17308=DIRECTION('center_axis',(-0.51355901341607,0.640299002836773,0.571204277562193));
#17309=DIRECTION('ref_axis',(-0.741965014102678,0.00298420341975993,-0.670431959543668));
#17310=DIRECTION('',(0.741965014102678,-0.00298420341976,0.670431959543668));
#17311=DIRECTION('',(0.741965014102678,-0.00298420341976,0.670431959543668));
#17312=DIRECTION('center_axis',(0.51355901341607,-0.640299002836773,-0.571204277562193));
#17313=DIRECTION('ref_axis',(-0.741965014102678,0.00298420341975985,-0.670431959543668));
#17314=DIRECTION('',(-0.741965014102678,0.00298420341975983,-0.670431959543668));
#17315=DIRECTION('',(-0.741965014102678,0.00298420341975983,-0.670431959543668));
#17316=DIRECTION('center_axis',(0.430981504924197,0.768119965562791,-0.473546894105632));
#17317=DIRECTION('ref_axis',(0.741965014102678,-0.00298420341976002,0.670431959543668));
#17318=DIRECTION('center_axis',(-0.741965014102677,0.00298420341975833,
-0.67043195954367));
#17319=DIRECTION('ref_axis',(-0.513559013416072,0.640299002836773,0.571204277562191));
#17320=DIRECTION('',(-0.513559013416072,0.640299002836773,0.571204277562191));
#17321=DIRECTION('',(-0.513559013416072,0.640299002836773,0.571204277562191));
#17322=DIRECTION('center_axis',(0.430981504924197,0.768119965562791,-0.473546894105632));
#17323=DIRECTION('ref_axis',(0.741965014102678,-0.00298420341976002,0.670431959543668));
#17324=DIRECTION('center_axis',(0.741965014102678,-0.00298420341976016,
0.670431959543668));
#17325=DIRECTION('ref_axis',(0.430981504924197,0.768119965562791,-0.473546894105632));
#17326=DIRECTION('center_axis',(-0.430981504924197,-0.768119965562791,0.473546894105632));
#17327=DIRECTION('ref_axis',(-0.51355901341607,0.640299002836773,0.571204277562193));
#17328=DIRECTION('center_axis',(0.430981504924197,0.768119965562791,-0.473546894105632));
#17329=DIRECTION('ref_axis',(0.741965014102678,-0.00298420341976002,0.670431959543668));
#17330=DIRECTION('center_axis',(-0.741965014102678,0.00298420341976011,
-0.670431959543668));
#17331=DIRECTION('ref_axis',(-0.51355901341607,0.640299002836773,0.571204277562193));
#17332=DIRECTION('center_axis',(-0.430981504924197,-0.768119965562791,0.473546894105632));
#17333=DIRECTION('ref_axis',(-0.51355901341607,0.640299002836773,0.571204277562193));
#17334=DIRECTION('',(-0.51355901341607,0.640299002836773,0.571204277562193));
#17335=DIRECTION('',(-0.741965014102678,0.00298420341976,-0.670431959543668));
#17336=DIRECTION('',(-0.51355901341607,0.640299002836773,0.571204277562193));
#17337=DIRECTION('',(-0.741965014102678,0.00298420341976,-0.670431959543668));
#17338=DIRECTION('center_axis',(-0.51355901341607,0.640299002836773,0.571204277562193));
#17339=DIRECTION('ref_axis',(-0.741965014102678,0.00298420341975993,-0.670431959543668));
#17340=DIRECTION('',(0.430981504924197,0.768119965562791,-0.473546894105632));
#17341=DIRECTION('',(0.430981504924197,0.768119965562791,-0.473546894105632));
#17342=DIRECTION('',(-0.741965014102678,0.00298420341976,-0.670431959543668));
#17343=DIRECTION('center_axis',(0.741965014102678,-0.00298420341976016,
0.670431959543668));
#17344=DIRECTION('ref_axis',(0.430981504924197,0.768119965562791,-0.473546894105632));
#17345=DIRECTION('',(0.51355901341607,-0.640299002836773,-0.571204277562193));
#17346=DIRECTION('',(-0.430981504924197,-0.768119965562791,0.473546894105632));
#17347=DIRECTION('center_axis',(-0.430981504924197,-0.768119965562791,0.473546894105632));
#17348=DIRECTION('ref_axis',(-0.51355901341607,0.640299002836773,0.571204277562193));
#17349=DIRECTION('center_axis',(0.51355901341607,-0.640299002836773,-0.571204277562193));
#17350=DIRECTION('ref_axis',(-0.430981504924197,-0.768119965562791,0.473546894105632));
#17351=DIRECTION('',(-0.741965014102678,0.00298420341976,-0.670431959543668));
#17352=DIRECTION('',(-0.430981504924197,-0.768119965562791,0.473546894105632));
#17353=DIRECTION('center_axis',(0.741965014102678,-0.00298420341976016,
0.670431959543668));
#17354=DIRECTION('ref_axis',(0.430981504924197,0.768119965562791,-0.473546894105632));
#17355=DIRECTION('',(0.51355901341607,-0.640299002836773,-0.571204277562193));
#17356=DIRECTION('center_axis',(0.430981504924197,0.768119965562791,-0.473546894105632));
#17357=DIRECTION('ref_axis',(0.741965014102678,-0.00298420341976002,0.670431959543668));
#17358=DIRECTION('center_axis',(-0.887789553801152,0.454869917367419,-0.0701645668105238));
#17359=DIRECTION('ref_axis',(0.430981504924197,0.768119965562791,-0.473546894105632));
#21388=CARTESIAN_POINT('',(0.,0.,0.));
#21389=CARTESIAN_POINT('Origin',(-21.1807292643367,67.0504890645402,23.2726194591173));
#21390=CARTESIAN_POINT('',(-18.4019669354104,62.2805003312476,20.1761396184593));
#21391=CARTESIAN_POINT('Origin',(-21.6117107692609,66.2823690989774,23.746166353223));
#21392=CARTESIAN_POINT('',(-17.540003925562,63.8167402623731,19.229045830248));
#21393=CARTESIAN_POINT('Origin',(-17.9709854304862,63.0486202968104,19.7025927243536));
#21394=CARTESIAN_POINT('Origin',(-20.7497477594125,67.818609030103,22.7990725650117));
#21395=CARTESIAN_POINT('Origin',(-19.370606943655,70.2765929199039,21.2837225038737));
#21396=CARTESIAN_POINT('',(-20.4706781590466,58.5935244965462,22.4491647101663));
#21397=CARTESIAN_POINT('',(-16.1608631098046,66.2747241521741,17.71369576911));
#21398=CARTESIAN_POINT('Origin',(-23.680421992897,62.595393264276,26.01919144493));
#21399=CARTESIAN_POINT('Origin',(-19.370606943655,70.2765929199039,21.2837225038737));
#21400=CARTESIAN_POINT('',(-16.0315686583273,66.5051601418429,17.5716317008783));
#21401=CARTESIAN_POINT('Origin',(-19.2413124921778,70.5070289095728,21.141658435642));
#21402=CARTESIAN_POINT('',(-16.1608631098046,66.2747241521741,17.71369576911));
#21403=CARTESIAN_POINT('Origin',(-26.7094064904571,75.8640834081228,29.4304205240279));
#21404=CARTESIAN_POINT('',(-35.1523449475666,57.3165090584927,38.6916365627459));
#21405=CARTESIAN_POINT('Origin',(-36.3078527277528,58.7571818148754,39.9768461872608));
#21406=CARTESIAN_POINT('',(-28.6876223737037,68.8383085419345,31.5884331511614));
#21407=CARTESIAN_POINT('',(-25.5538987102709,74.42341065174,28.145210899513));
#21408=CARTESIAN_POINT('Origin',(-29.8431301538898,70.2789812983173,32.8736427756763));
#21409=CARTESIAN_POINT('Origin',(-44.6514843000067,41.123844669555,31.2333209653637));
#21410=CARTESIAN_POINT('',(-56.5796715376924,43.0865205259419,23.5608863644389));
#21411=CARTESIAN_POINT('Origin',(-55.0389944974442,41.1656235174316,21.8472735317523));
#21412=CARTESIAN_POINT('',(-46.1921613402549,43.0447416780653,32.9469337980503));
#21413=CARTESIAN_POINT('',(-46.1921613402549,43.0447416780653,32.9469337980503));
#21414=CARTESIAN_POINT('Origin',(-44.6514843000067,41.123844669555,31.2333209653637));
#21415=CARTESIAN_POINT('Origin',(-30.14514456676,51.0735937808341,33.1223948565145));
#21416=CARTESIAN_POINT('',(-33.9968371673805,55.8758363021099,37.4064269382309));
#21417=CARTESIAN_POINT('Origin',(-30.14514456676,51.0735937808341,33.1223948565145));
#21418=CARTESIAN_POINT('',(-37.1511444364363,46.7539638900993,40.8566862547723));
#21419=CARTESIAN_POINT('',(-33.9968371673805,55.8758363021099,37.4064269382309));
#21420=CARTESIAN_POINT('',(-34.1986576758722,40.5370964920739,33.4596727214903));
#21421=CARTESIAN_POINT('Origin',(-34.4549596160019,43.3923941252062,37.8578637975708));
#21422=CARTESIAN_POINT('',(-38.7920691336964,46.2641048771473,38.5686790961612));
#21423=CARTESIAN_POINT('Ctrl Pts',(-34.1986576758724,40.5370964920741,33.45967272149));
#21424=CARTESIAN_POINT('Ctrl Pts',(-34.4388615494162,40.8333519186998,33.1851139522211));
#21425=CARTESIAN_POINT('Ctrl Pts',(-34.6772423136203,41.1581168909091,32.9429616455856));
#21426=CARTESIAN_POINT('Ctrl Pts',(-35.1372914510471,41.801250072958,32.5593008372811));
#21427=CARTESIAN_POINT('Ctrl Pts',(-35.3897505951037,42.1636734305047,32.3895385975851));
#21428=CARTESIAN_POINT('Ctrl Pts',(-35.909488224246,42.9090203866848,32.1640747104879));
#21429=CARTESIAN_POINT('Ctrl Pts',(-36.1772556001164,43.2919128390833,32.1093985180926));
#21430=CARTESIAN_POINT('Ctrl Pts',(-36.6333809306673,43.9313791060147,32.1273079452342));
#21431=CARTESIAN_POINT('Ctrl Pts',(-36.8589905041216,44.2427361852693,32.1806242970088));
#21432=CARTESIAN_POINT('Ctrl Pts',(-37.2963729868296,44.8287243856034,32.4038996940975));
#21433=CARTESIAN_POINT('Ctrl Pts',(-37.508133475892,45.1030694943354,32.5746329487417));
#21434=CARTESIAN_POINT('Ctrl Pts',(-37.8722215204345,45.5570099486458,32.9795886461766));
#21435=CARTESIAN_POINT('Ctrl Pts',(-38.0527564083383,45.7717738461373,33.2451845991546));
#21436=CARTESIAN_POINT('Ctrl Pts',(-38.3624638742306,46.1172481196795,33.8528574732792));
#21437=CARTESIAN_POINT('Ctrl Pts',(-38.4919084454301,46.2485681404971,34.1944488943104));
#21438=CARTESIAN_POINT('Ctrl Pts',(-38.7074431493876,46.4465192669056,34.9235910712811));
#21439=CARTESIAN_POINT('Ctrl Pts',(-38.8006550994683,46.5136913570681,35.3797652993612));
#21440=CARTESIAN_POINT('Ctrl Pts',(-38.912980144043,46.5563922963369,36.3082387598139));
#21441=CARTESIAN_POINT('Ctrl Pts',(-38.93244337546,46.5329983810086,36.7804457429138));
#21442=CARTESIAN_POINT('Ctrl Pts',(-38.9129366855058,46.4391280537729,37.6540984000036));
#21443=CARTESIAN_POINT('Ctrl Pts',(-38.8718148058301,46.3603030101108,38.1156512344973));
#21444=CARTESIAN_POINT('Ctrl Pts',(-38.7920691336965,46.2641048771474,38.5686790961607));
#21445=CARTESIAN_POINT('Origin',(-34.4549596160019,43.3923941252062,37.8578637975708));
#21446=CARTESIAN_POINT('Origin',(-30.14514456676,51.0735937808341,33.1223948565145));
#21447=CARTESIAN_POINT('',(-15.2504730073405,57.296061780678,25.0955865772773));
#21448=CARTESIAN_POINT('',(-31.8377985837207,68.1554663069955,27.6138057991849));
#21449=CARTESIAN_POINT('Origin',(-23.680421992897,62.595393264276,26.01919144493));
#21450=CARTESIAN_POINT('',(-21.7151955812034,45.7742622972361,32.1987899888618));
#21451=CARTESIAN_POINT('',(-21.7151955812034,45.7742622972361,32.1987899888618));
#21452=CARTESIAN_POINT('',(-38.3025211575837,56.6336668235536,34.7170092107694));
#21453=CARTESIAN_POINT('Origin',(-30.14514456676,51.0735937808341,33.1223948565145));
#21454=CARTESIAN_POINT('',(-38.3025211575837,56.6336668235536,34.7170092107694));
#21455=CARTESIAN_POINT('Origin',(-37.9028116553955,37.2474344007039,41.6462389504159));
#21456=CARTESIAN_POINT('',(-38.3363435749778,44.6416339848016,42.1589402135628));
#21457=CARTESIAN_POINT('Origin',(-35.6401587544779,41.2800642198147,39.1601177563349));
#21458=CARTESIAN_POINT('',(-38.6265215709417,44.4465365776215,42.1063169921011));
#21459=CARTESIAN_POINT('Origin',(-32.946681053115,37.9218104167842,36.1642663517435));
#21460=CARTESIAN_POINT('',(-33.2402691976586,37.7310239811241,36.1154759879024));
#21461=CARTESIAN_POINT('Origin',(-35.7479041307745,41.0880342285179,39.2785044798877));
#21462=CARTESIAN_POINT('',(-32.9439739341091,37.9184944550155,36.1612952991598));
#21463=CARTESIAN_POINT('Origin',(-38.3336988439063,44.6382773263309,42.1559586889937));
#21464=CARTESIAN_POINT('Origin',(-35.6401587545408,41.2800642199063,39.1601177563553));
#21465=CARTESIAN_POINT('Origin',(-40.1823782592027,41.1368009396544,35.2368865760798));
#21466=CARTESIAN_POINT('',(-48.8866349100272,38.6188758778939,23.2308060524478));
#21467=CARTESIAN_POINT('Origin',(-50.9408709636915,41.1800718892409,25.5156231626966));
#21468=CARTESIAN_POINT('',(-38.1281422055384,38.5756049283073,32.952069465831));
#21469=CARTESIAN_POINT('',(-38.1281422055384,38.5756049283073,32.952069465831));
#21470=CARTESIAN_POINT('Origin',(-40.1823782592027,41.1368009396544,35.2368865760798));
#21471=CARTESIAN_POINT('Origin',(-40.0919488391595,41.2979694404271,35.1375259990993));
#21472=CARTESIAN_POINT('',(-42.3546017400116,37.2653396212225,37.6236471931538));
#21473=CARTESIAN_POINT('Origin',(-40.0919488391595,41.2979694404271,35.1375259990993));
#21474=CARTESIAN_POINT('',(-41.7981279794346,37.2631014686576,38.1264711628116));
#21475=CARTESIAN_POINT('',(-42.3546017400116,37.2653396212225,37.6236471931539));
#21476=CARTESIAN_POINT('Origin',(-35.6400470347534,41.2800655852767,39.1600770240352));
#21477=CARTESIAN_POINT('Origin',(-35.6401289648185,41.2801677346543,39.1601681504663));
#21478=CARTESIAN_POINT('Origin',(-40.1823782592027,41.1368009396544,35.2368865760798));
#21479=CARTESIAN_POINT('',(-51.320302201284,37.9647877832075,19.9549241160537));
#21480=CARTESIAN_POINT('Origin',(-53.9087310201022,41.19200870292,22.8338953245219));
#21481=CARTESIAN_POINT('',(-48.3524421448733,37.9528509695284,22.6366519542284));
#21482=CARTESIAN_POINT('',(-37.5939494403844,37.9095800199419,32.3579153676115));
#21483=CARTESIAN_POINT('Origin',(-50.9408709636915,41.1800718892409,25.5156231626966));
#21484=CARTESIAN_POINT('Origin',(-53.9087310201022,41.19200870292,22.8338953245219));
#21485=CARTESIAN_POINT('',(-52.967442487592,38.6352889967025,19.5434302749577));
#21486=CARTESIAN_POINT('',(-51.320302201284,37.9647877832074,19.9549241160537));
#21487=CARTESIAN_POINT('Origin',(-55.0216785412562,41.1964850080496,21.8282473852064));
#21488=CARTESIAN_POINT('Origin',(-17.0720934772965,71.2619488126406,18.7443506111377));
#21489=CARTESIAN_POINT('',(-17.2046121060751,71.4924445117698,18.892034549701));
#21490=CARTESIAN_POINT('Origin',(-17.0505444020503,71.3003548109187,18.7206732664324));
#21491=CARTESIAN_POINT('',(-17.2261611813213,71.4540385134916,18.9157118944063));
#21492=CARTESIAN_POINT('',(-17.2261611813213,71.4540385134916,18.9157118944063));
#21493=CARTESIAN_POINT('Origin',(-17.0720934772965,71.2619488126406,18.7443506111377));
#21494=CARTESIAN_POINT('Origin',(-19.1263295309608,73.8231448239877,21.0291677213865));
#21495=CARTESIAN_POINT('',(-19.2588481597394,74.0536405231169,21.1768516599498));
#21496=CARTESIAN_POINT('Origin',(-19.1047804557146,73.8615508222658,21.0054903766812));
#21497=CARTESIAN_POINT('',(-19.2803972349856,74.0152345248387,21.2005290046551));
#21498=CARTESIAN_POINT('',(-19.2803972349856,74.0152345248387,21.2005290046551));
#21499=CARTESIAN_POINT('Origin',(-19.1263295309608,73.8231448239877,21.0291677213865));
#21500=CARTESIAN_POINT('Origin',(-19.370606943655,70.2765929199039,21.2837225038737));
#21501=CARTESIAN_POINT('',(-16.0234263752182,70.0197568052452,17.578264711308));
#21502=CARTESIAN_POINT('Origin',(-18.0776624288824,72.5809528165923,19.8630818215568));
#21503=CARTESIAN_POINT('',(-15.8079356227561,70.4038167880266,17.3414912642552));
#21504=CARTESIAN_POINT('',(-17.3163708899908,67.7153969085568,18.9989053936249));
#21505=CARTESIAN_POINT('Origin',(-17.8621716764203,72.9650127993737,19.626308374504));
#21506=CARTESIAN_POINT('Origin',(-18.1854078051135,72.3889228252016,19.9814685450832));
#21507=CARTESIAN_POINT('',(-16.1976283734343,68.931487338264,17.7662094666325));
#21508=CARTESIAN_POINT('Origin',(-18.5086439338066,71.8128328510295,20.3366287156624));
#21509=CARTESIAN_POINT('',(-15.551156116048,70.0836672866082,17.0558891254741));
#21510=CARTESIAN_POINT('Origin',(-15.8743922447412,69.5075773124361,17.4110492960533));
#21511=CARTESIAN_POINT('Origin',(-17.8621716764203,72.9650127993737,19.626308374504));
#21512=CARTESIAN_POINT('Origin',(-19.370606943655,70.2765929199039,21.2837225038737));
#21513=CARTESIAN_POINT('',(-16.3516960774591,69.123577039115,17.9375707499012));
#21514=CARTESIAN_POINT('Origin',(-18.5086439338066,71.8128328510295,20.3366287156624));
#21515=CARTESIAN_POINT('',(-16.9981683348454,67.9713970907709,18.6478910910597));
#21516=CARTESIAN_POINT('',(-17.2136590873075,67.5873371079895,18.8846645381125));
#21517=CARTESIAN_POINT('Origin',(-19.1551161911929,70.6606529026853,21.0469490568209));
#21518=CARTESIAN_POINT('Origin',(-19.1551161911929,70.6606529026853,21.0469490568209));
#21519=CARTESIAN_POINT('',(-16.9733950822979,67.548871400251,18.6185938760227));
#21520=CARTESIAN_POINT('Origin',(-19.2844106426702,70.4302169130165,21.1890131250526));
#21521=CARTESIAN_POINT('',(-16.9981683348454,67.9713970907709,18.6478910910597));
#21522=CARTESIAN_POINT('Origin',(-19.370606943655,70.2765929199039,21.2837225038737));
#21523=CARTESIAN_POINT('',(-16.305768364857,66.7164826965632,17.8760283151918));
#21524=CARTESIAN_POINT('Origin',(-19.2844106426702,70.4302169130165,21.1890131250526));
#21525=CARTESIAN_POINT('',(-16.2626702143646,66.7932946931195,17.8286736257813));
#21526=CARTESIAN_POINT('',(-16.3919646658418,66.5628587034506,17.970737694013));
#21527=CARTESIAN_POINT('Origin',(-19.2413124921778,70.5070289095728,21.141658435642));
#21528=CARTESIAN_POINT('Origin',(-16.9733950822979,67.548871400251,18.6185938760227));
#21529=CARTESIAN_POINT('Origin',(-16.3516960774591,69.123577039115,17.9375707499012));
#21530=CARTESIAN_POINT('Origin',(-15.8079356227561,70.4038167880266,17.3414912642552));
#21531=CARTESIAN_POINT('Origin',(-19.1263295309608,73.8231448239877,21.0291677213865));
#21532=CARTESIAN_POINT('Origin',(-17.0720934772965,71.2619488126406,18.7443506111377));
#21533=CARTESIAN_POINT('Origin',(-5.87326165443273,62.5237723822018,42.109558473978));
#21534=CARTESIAN_POINT('',(-10.1675813678396,57.8258167527581,46.8411576859596));
#21535=CARTESIAN_POINT('',(-10.4261702707941,57.3649447734205,47.125285822423));
#21536=CARTESIAN_POINT('',(-10.1675813678396,57.8258167527581,46.8411576859596));
#21537=CARTESIAN_POINT('',(-11.2974111973549,59.234474558999,48.0978070965964));
#21538=CARTESIAN_POINT('',(-11.2974111973549,59.234474558999,48.0978070965964));
#21539=CARTESIAN_POINT('',(-11.5560001003095,58.7736025796614,48.3819352330598));
#21540=CARTESIAN_POINT('',(-11.5560001003095,58.7736025796614,48.3819352330598));
#21541=CARTESIAN_POINT('',(-10.4261702707941,57.3649447734205,47.125285822423));
#21542=CARTESIAN_POINT('Origin',(-11.2974111973549,59.234474558999,48.0978070965964));
#21543=CARTESIAN_POINT('',(-17.975096324279,59.2613323897769,42.0639194607034));
#21544=CARTESIAN_POINT('',(-16.8452664947637,57.852674583536,40.8072700500666));
#21545=CARTESIAN_POINT('',(-17.975096324279,59.2613323897769,42.0639194607034));
#21546=CARTESIAN_POINT('',(-11.2974111973549,59.234474558999,48.0978070965964));
#21547=CARTESIAN_POINT('',(-10.1675813678396,57.8258167527581,46.8411576859596));
#21548=CARTESIAN_POINT('Origin',(-11.5560001003095,58.7736025796614,48.3819352330598));
#21549=CARTESIAN_POINT('',(-18.2336852272336,58.8004604104392,42.3480475971668));
#21550=CARTESIAN_POINT('',(-18.2336852272336,58.8004604104392,42.3480475971668));
#21551=CARTESIAN_POINT('',(-11.5560001003095,58.7736025796614,48.3819352330598));
#21552=CARTESIAN_POINT('Origin',(-10.4261702707941,57.3649447734205,47.125285822423));
#21553=CARTESIAN_POINT('',(-17.1038553977182,57.3918026041983,41.0913981865299));
#21554=CARTESIAN_POINT('',(-17.1038553977182,57.3918026041983,41.0913981865299));
#21555=CARTESIAN_POINT('',(-10.4261702707941,57.3649447734205,47.125285822423));
#21556=CARTESIAN_POINT('Origin',(-5.13129664033005,62.520788178782,42.7799904335217));
#21557=CARTESIAN_POINT('',(-10.3946991891447,50.8066601566478,48.5528405346573));
#21558=CARTESIAN_POINT('',(-10.9118769950537,49.8849161979724,49.121096807584));
#21559=CARTESIAN_POINT('',(-10.3946991891447,50.8066601566478,48.5528405346573));
#21560=CARTESIAN_POINT('',(-11.9353762293929,52.7275571651581,50.2664533673438));
#21561=CARTESIAN_POINT('',(-11.9353762293929,52.7275571651581,50.2664533673438));
#21562=CARTESIAN_POINT('',(-12.452554035302,51.8058132064827,50.8347096402706));
#21563=CARTESIAN_POINT('',(-12.452554035302,51.8058132064827,50.8347096402706));
#21564=CARTESIAN_POINT('',(-10.9118769950537,49.8849161979724,49.121096807584));
#21565=CARTESIAN_POINT('Origin',(-12.452554035302,51.8058132064827,50.8347096402706));
#21566=CARTESIAN_POINT('',(-19.4412226714045,52.6037752062431,43.6568431507283));
#21567=CARTESIAN_POINT('',(-19.3550263704197,52.7573991993557,43.5621337719072));
#21568=CARTESIAN_POINT('',(-19.8722041763287,51.8356552406803,44.1303900448339));
#21569=CARTESIAN_POINT('',(-19.1302391622261,51.8326710372606,44.8008220043776));
#21570=CARTESIAN_POINT('',(-17.7308133709229,48.3627022768391,49.9487268457994));
#21571=CARTESIAN_POINT('',(-12.452554035302,51.8058132064827,50.8347096402706));
#21572=CARTESIAN_POINT('',(-11.9353762293929,52.7275571651581,50.2664533673438));
#21573=CARTESIAN_POINT('Origin',(-10.9118769950537,49.8849161979724,49.121096807584));
#21574=CARTESIAN_POINT('',(-17.5895621219778,49.9117740287503,43.087209171691));
#21575=CARTESIAN_POINT('',(-17.5895621219778,49.9117740287503,43.087209171691));
#21576=CARTESIAN_POINT('',(-10.9118769950537,49.8849161979724,49.121096807584));
#21577=CARTESIAN_POINT('Origin',(-0.643450268341849,55.6976051691234,40.0202968711604));
#21578=CARTESIAN_POINT('',(-1.75639778949586,55.702081474253,39.0146489318449));
#21579=CARTESIAN_POINT('',(-9.17604793052264,55.7319235084507,32.3103293364082));
#21580=CARTESIAN_POINT('',(-0.643450268341849,55.6976051691234,40.0202968711604));
#21581=CARTESIAN_POINT('',(-6.92817584858623,46.4846418874996,44.6972116611125));
#21582=CARTESIAN_POINT('',(-6.92817584858623,46.4846418874996,44.6972116611125));
#21583=CARTESIAN_POINT('',(-14.347825989613,46.5144839216971,37.9928920656758));
#21584=CARTESIAN_POINT('',(-5.81522832743221,46.4801655823699,45.702859600428));
#21585=CARTESIAN_POINT('',(-9.17604793052264,55.7319235084507,32.3103293364082));
#21586=CARTESIAN_POINT('Origin',(-9.11717398970701,66.2625387159302,49.4451674509366));
#21587=CARTESIAN_POINT('',(-10.230121510861,66.2670150210598,48.4395195116211));
#21588=CARTESIAN_POINT('',(-17.6497716518878,66.2968570552574,41.7351999161844));
#21589=CARTESIAN_POINT('',(-9.11717398970701,66.2625387159302,49.4451674509366));
#21590=CARTESIAN_POINT('',(-1.75639778949586,55.702081474253,39.0146489318449));
#21591=CARTESIAN_POINT('',(-17.6497716518878,66.2968570552574,41.7351999161844));
#21592=CARTESIAN_POINT('Origin',(-14.2889520487974,57.0450991291767,55.1277301802041));
#21593=CARTESIAN_POINT('',(-15.4018995699514,57.0495754343063,54.1220822408886));
#21594=CARTESIAN_POINT('',(-22.8215497109782,57.0794174685039,47.417762645452));
#21595=CARTESIAN_POINT('',(-14.2889520487974,57.0450991291767,55.1277301802041));
#21596=CARTESIAN_POINT('',(-10.230121510861,66.2670150210598,48.4395195116211));
#21597=CARTESIAN_POINT('',(-22.8215497109782,57.0794174685039,47.417762645452));
#21598=CARTESIAN_POINT('Origin',(-21.8109151771594,55.9930238221405,35.1010433319011));
#21599=CARTESIAN_POINT('',(-12.4413136191775,55.6742799812288,32.9405810371301));
#21600=CARTESIAN_POINT('',(-9.17604793052264,55.7319235084507,32.3103293364082));
#21601=CARTESIAN_POINT('',(-18.8608012868784,63.6780175166885,40.0806345066575));
#21602=CARTESIAN_POINT('',(-12.4413136191775,55.6742799812288,32.9405810371301));
#21603=CARTESIAN_POINT('',(-17.6497716518878,66.2968570552574,41.7351999161844));
#21604=CARTESIAN_POINT('Origin',(-22.9095517405797,64.7463307123084,30.2097137451623));
#21605=CARTESIAN_POINT('',(-16.1046564110332,49.1452602739451,36.965729637028));
#21606=CARTESIAN_POINT('',(-14.347825989613,46.5144839216971,37.9928920656758));
#21607=CARTESIAN_POINT('',(-16.1046564110332,49.1452602739451,36.965729637028));
#21608=CARTESIAN_POINT('Origin',(-5.81522832743221,46.4801655823699,45.702859600428));
#21609=CARTESIAN_POINT('',(-15.4018995699514,57.0495754343063,54.1220822408886));
#21610=CARTESIAN_POINT('',(-14.347825989613,46.5144839216971,37.9928920656758));
#21611=CARTESIAN_POINT('Origin',(-24.2157427890632,62.2160260775154,25.9631512684015));
#21612=CARTESIAN_POINT('',(-22.524144078734,57.1489978094048,44.1057831065554));
#21613=CARTESIAN_POINT('',(-22.524144078734,57.1489978094048,44.1057831065554));
#21614=CARTESIAN_POINT('',(-17.8143493301715,50.8365021908454,41.8485209392206));
#21615=CARTESIAN_POINT('',(-14.347825989613,46.5144839216971,37.9928920656758));
#21616=CARTESIAN_POINT('',(-19.3550263704197,52.7573991993557,43.5621337719072));
#21617=CARTESIAN_POINT('',(-22.8215497109782,57.0794174685039,47.417762645452));
#21618=CARTESIAN_POINT('Origin',(-19.4430284000212,60.4243124431602,26.3540848716175));
#21619=CARTESIAN_POINT('',(-18.8608012868784,63.6780175166885,40.0806345066575));
#21620=CARTESIAN_POINT('Origin',(-12.4413136191775,55.6742799812288,32.9405810371301));
#21621=CARTESIAN_POINT('',(-13.1832786332802,55.6772641846486,32.2701490775864));
#21622=CARTESIAN_POINT('',(-19.602766300981,63.6810017201083,39.4102025471138));
#21623=CARTESIAN_POINT('',(-13.1832786332802,55.6772641846486,32.2701490775864));
#21624=CARTESIAN_POINT('',(-18.8608012868784,63.6780175166885,40.0806345066575));
#21625=CARTESIAN_POINT('',(-12.4413136191775,55.6742799812288,32.9405810371301));
#21626=CARTESIAN_POINT('Origin',(-16.1046564110332,49.1452602739451,36.965729637028));
#21627=CARTESIAN_POINT('',(-16.8466214251358,49.1482444773649,36.2952976774843));
#21628=CARTESIAN_POINT('',(-16.8466214251358,49.1482444773649,36.2952976774843));
#21629=CARTESIAN_POINT('',(-16.1046564110332,49.1452602739451,36.965729637028));
#21630=CARTESIAN_POINT('Origin',(-22.524144078734,57.1489978094048,44.1057831065554));
#21631=CARTESIAN_POINT('',(-23.2661090928367,57.1519820128245,43.4353511470117));
#21632=CARTESIAN_POINT('',(-23.2661090928367,57.1519820128245,43.4353511470117));
#21633=CARTESIAN_POINT('',(-22.524144078734,57.1489978094048,44.1057831065554));
#21634=CARTESIAN_POINT('Origin',(-18.8608012868784,63.6780175166885,40.0806345066575));
#21635=CARTESIAN_POINT('',(-19.602766300981,63.6810017201083,39.4102025471138));
#21636=CARTESIAN_POINT('Origin',(-49.2169449439947,44.2525517514921,23.6214355862741));
#21637=CARTESIAN_POINT('Origin',(-4.01834911917603,62.5163118736524,43.7856383728372));
#21638=CARTESIAN_POINT('',(-12.872141271287,57.2368305732657,53.5606034227024));
#21639=CARTESIAN_POINT('',(-12.8464633206162,57.2048156231239,53.5320432088243));
#21640=CARTESIAN_POINT('',(-5.16875607004592,47.6323455307141,44.9925392592695));
#21641=CARTESIAN_POINT('',(-8.96762977629839,64.117895313189,49.2701211618736));
#21642=CARTESIAN_POINT('',(-7.4591945090637,66.8063151926587,47.6127070325039));
#21643=CARTESIAN_POINT('',(-8.9933077269692,64.1499102633308,49.2986813757517));
#21644=CARTESIAN_POINT('',(-9.7636462470933,65.110358767586,50.155487792095));
#21645=CARTESIAN_POINT('',(-13.5186135286733,56.0846506249215,54.2709237638608));
#21646=CARTESIAN_POINT('Origin',(-20.5885881684815,57.5590446260281,44.948685785673));
#21647=CARTESIAN_POINT('',(-20.5885881684815,57.5590446260281,44.948685785673));
#21648=CARTESIAN_POINT('',(-12.7979555204034,57.5277104901207,51.9882213608815));
#21649=CARTESIAN_POINT('',(-20.5885881684815,57.5590446260281,44.948685785673));
#21650=CARTESIAN_POINT('',(-6.63524735941056,49.8441224560794,45.1337700301351));
#21651=CARTESIAN_POINT('',(-12.7979555204034,57.5277104901207,51.9882213608815));
#21652=CARTESIAN_POINT('',(-14.4258800074887,49.8754565919869,38.0942344549266));
#21653=CARTESIAN_POINT('',(-14.4258800074887,49.8754565919869,38.0942344549266));
#21654=CARTESIAN_POINT('',(-20.5885881684815,57.5590446260281,44.948685785673));
#21655=CARTESIAN_POINT('Origin',(-14.4258800074887,49.8754565919869,38.0942344549266));
#21656=CARTESIAN_POINT('',(-6.54195230665701,49.6127912053846,45.4769636862299));
#21657=CARTESIAN_POINT('',(-8.26791078259758,53.8924193432378,39.1278810484763));
#21658=CARTESIAN_POINT('',(-3.26649286923312,55.4505029436618,41.8780072910271));
#21659=CARTESIAN_POINT('',(-6.41265785517975,49.8432271950535,45.3348996179982));
#21660=CARTESIAN_POINT('',(-3.61837682494118,55.2209622150189,41.8189417713957));
#21661=CARTESIAN_POINT('',(-13.8816588664263,48.5260242962674,40.0961974488129));
#21662=CARTESIAN_POINT('',(-11.4090094730193,55.2522963509264,34.7794061961872));
#21663=CARTESIAN_POINT('',(-11.4090094730193,55.2522963509264,34.7794061961872));
#21664=CARTESIAN_POINT('',(-14.4258800074887,49.8754565919869,38.0942344549266));
#21665=CARTESIAN_POINT('Origin',(-10.1675813678396,57.8258167527581,46.8411576859596));
#21666=CARTESIAN_POINT('',(-16.8452664947637,57.852674583536,40.8072700500666));
#21667=CARTESIAN_POINT('Origin',(-6.41265785517975,49.8432271950535,45.3348996179982));
#21668=CARTESIAN_POINT('',(-5.96477254084083,48.6248089851111,45.8779058894909));
#21669=CARTESIAN_POINT('',(-6.62440655891647,49.7539315225666,45.4196862286212));
#21670=CARTESIAN_POINT('',(-2.08593899652305,55.5378886751762,41.6159838425402));
#21671=CARTESIAN_POINT('',(-0.577503729288366,58.226308554646,39.9585697131705));
#21672=CARTESIAN_POINT('',(-7.37032299817759,55.1467334960166,42.7888507071959));
#21673=CARTESIAN_POINT('Origin',(-11.4090094730193,55.2522963509264,34.7794061961872));
#21674=CARTESIAN_POINT('',(-9.78108498593402,62.9045502490602,48.673393102142));
#21675=CARTESIAN_POINT('',(-3.61837682494118,55.2209622150189,41.8189417713957));
#21676=CARTESIAN_POINT('',(-17.5717176340121,62.9358843849677,41.6338575269335));
#21677=CARTESIAN_POINT('',(-17.5717176340121,62.9358843849677,41.6338575269335));
#21678=CARTESIAN_POINT('',(-11.4090094730193,55.2522963509264,34.7794061961872));
#21679=CARTESIAN_POINT('Origin',(-12.7979555204034,57.5277104901207,51.9882213608815));
#21680=CARTESIAN_POINT('',(-12.7046604676499,57.2963792394259,52.3314150169762));
#21681=CARTESIAN_POINT('',(-15.5190612257151,64.274871968718,41.9784063914501));
#21682=CARTESIAN_POINT('',(-12.2117267406717,57.6146718103806,48.1578027310283));
#21683=CARTESIAN_POINT('',(-5.16875607004592,47.6323455307141,44.9925392592695));
#21684=CARTESIAN_POINT('Origin',(-3.61837682494118,55.2209622150189,41.8189417713957));
#21685=CARTESIAN_POINT('',(-9.7636462470933,65.110358767586,50.155487792095));
#21686=CARTESIAN_POINT('',(-9.42920103022596,63.1340909777031,48.7324586217735));
#21687=CARTESIAN_POINT('',(-9.49513978078704,62.9935475012051,48.6556496874734));
#21688=CARTESIAN_POINT('',(-15.9390542108251,58.8875874978093,47.6397465085924));
#21689=CARTESIAN_POINT('Origin',(-12.5509467813568,62.5506302129796,36.075670838085));
#21690=CARTESIAN_POINT('',(-17.9005456311563,50.6828781977328,41.9432303180417));
#21691=CARTESIAN_POINT('',(-17.8143493301715,50.8365021908454,41.8485209392206));
#21692=CARTESIAN_POINT('',(-18.6708841512804,51.643326701988,42.800036734385));
#21693=CARTESIAN_POINT('Origin',(-17.5717176340121,62.9358843849677,41.6338575269335));
#21694=CARTESIAN_POINT('',(-9.55849548170321,62.9036549880343,48.8745226900051));
#21695=CARTESIAN_POINT('',(-17.5717176340121,62.9358843849677,41.6338575269335));
#21696=CARTESIAN_POINT('Origin',(-18.6708841512804,51.643326701988,42.800036734385));
#21697=CARTESIAN_POINT('',(-16.3767264361818,46.9044677697183,47.5487267009233));
#21698=CARTESIAN_POINT('Origin',(-4.01834911917603,62.5163118736524,43.7856383728372));
#21699=CARTESIAN_POINT('',(-2.06026104585225,55.5058737250344,41.5874236286621));
#21700=CARTESIAN_POINT('',(-9.7636462470933,65.110358767586,50.155487792095));
#21701=CARTESIAN_POINT('',(-5.93909459017002,48.5927940349693,45.8493456756128));
#21702=CARTESIAN_POINT('',(-5.16875607004592,47.6323455307141,44.9925392592695));
#21703=CARTESIAN_POINT('',(-1.41378878846595,56.6580536733786,40.8771032875037));
#21704=CARTESIAN_POINT('Origin',(-1.75639778949586,55.702081474253,39.0146489318449));
#21705=CARTESIAN_POINT('',(-1.75639778949586,55.702081474253,39.0146489318449));
#21706=CARTESIAN_POINT('',(-6.92817584858623,46.4846418874996,44.6972116611125));
#21707=CARTESIAN_POINT('Origin',(-6.92817584858623,46.4846418874996,44.6972116611125));
#21708=CARTESIAN_POINT('',(-6.12611914151519,57.7361776104907,52.0633265742058));
#21709=CARTESIAN_POINT('',(-15.4018995699514,57.0495754343063,54.1220822408886));
#21710=CARTESIAN_POINT('Origin',(-10.230121510861,66.2670150210598,48.4395195116211));
#21711=CARTESIAN_POINT('',(-10.230121510861,66.2670150210598,48.4395195116211));
#21712=CARTESIAN_POINT('Origin',(-10.3946991891447,50.8066601566478,48.5528405346573));
#21713=CARTESIAN_POINT('',(-10.3946991891447,50.8066601566478,48.5528405346573));
#21714=CARTESIAN_POINT('Origin',(-15.4018995699514,57.0495754343063,54.1220822408886));
#21715=CARTESIAN_POINT('Origin',(-40.0919488391595,41.2979694404271,35.1375259990993));
#21716=CARTESIAN_POINT('Ctrl Pts',(-41.7981279794346,37.2631014686576,38.1264711628116));
#21717=CARTESIAN_POINT('Ctrl Pts',(-41.7981279794346,37.2631014686576,38.1264711628116));
#21718=CARTESIAN_POINT('Ctrl Pts',(-41.7981279794346,37.2631014686576,38.1264711628116));
#21719=CARTESIAN_POINT('Ctrl Pts',(-41.7981279794346,37.2631014686576,38.1264711628116));
#21720=CARTESIAN_POINT('Ctrl Pts',(-41.7981279794346,37.2631014686576,38.1264711628116));
#21721=CARTESIAN_POINT('Ctrl Pts',(-41.7981279794346,37.2631014686576,38.1264711628116));
#21722=CARTESIAN_POINT('Ctrl Pts',(-41.7981279794346,37.2631014686576,38.1264711628116));
#21723=CARTESIAN_POINT('Ctrl Pts',(-41.7981279794346,37.2631014686576,38.1264711628116));
#21724=CARTESIAN_POINT('Ctrl Pts',(-41.7981279794346,37.2631014686576,38.1264711628116));
#21725=CARTESIAN_POINT('Ctrl Pts',(-41.7981279794346,37.2631014686576,38.1264711628116));
#21726=CARTESIAN_POINT('Ctrl Pts',(-41.7981279794346,37.2631014686576,38.1264711628116));
#21727=CARTESIAN_POINT('Ctrl Pts',(-41.7981279794346,37.2631014686576,38.1264711628116));
#21728=CARTESIAN_POINT('Ctrl Pts',(-41.7981279794346,37.2631014686576,38.1264711628116));
#21729=CARTESIAN_POINT('Ctrl Pts',(-41.7981279794346,37.2631014686576,38.1264711628116));
#21730=CARTESIAN_POINT('Ctrl Pts',(-41.7981279794346,37.2631014686576,38.1264711628116));
#21731=CARTESIAN_POINT('Ctrl Pts',(-41.7981279794346,37.2631014686576,38.1264711628116));
#21732=CARTESIAN_POINT('Ctrl Pts',(-41.7981279794346,37.2631014686576,38.1264711628116));
#21733=CARTESIAN_POINT('Ctrl Pts',(-41.7981279794346,37.2631014686576,38.1264711628116));
#21734=CARTESIAN_POINT('Ctrl Pts',(-41.7981279794346,37.2631014686576,38.1264711628116));
#21735=CARTESIAN_POINT('Ctrl Pts',(-41.7981279794346,37.2631014686576,38.1264711628116));
#21736=CARTESIAN_POINT('Ctrl Pts',(-41.7981279794346,37.2631014686576,38.1264711628116));
#21737=CARTESIAN_POINT('Ctrl Pts',(-41.7981279794346,37.2631014686576,38.1264711628116));
#21738=CARTESIAN_POINT('Ctrl Pts',(-41.7981279794346,37.2631014686576,38.1264711628116));
#21739=CARTESIAN_POINT('Ctrl Pts',(-41.7981279794346,37.2631014686576,38.1264711628116));
#21740=CARTESIAN_POINT('Ctrl Pts',(-41.7981279794346,37.2631014686576,38.1264711628116));
#21741=CARTESIAN_POINT('Ctrl Pts',(-41.7981279794346,37.2631014686576,38.1264711628116));
#21742=CARTESIAN_POINT('Ctrl Pts',(-41.7981279794346,37.2631014686576,38.1264711628116));
#21743=CARTESIAN_POINT('Ctrl Pts',(-41.7981279794346,37.2631014686576,38.1264711628116));
#21744=CARTESIAN_POINT('Ctrl Pts',(-41.7981279794346,37.2631014686576,38.1264711628116));
#21745=CARTESIAN_POINT('Ctrl Pts',(-41.7981279794346,37.2631014686576,38.1264711628116));
#21746=CARTESIAN_POINT('Ctrl Pts',(-41.7981279794346,37.2631014686576,38.1264711628116));
#21747=CARTESIAN_POINT('Ctrl Pts',(-41.7981279794346,37.2631014686576,38.1264711628116));
#21748=CARTESIAN_POINT('Ctrl Pts',(-41.7981279794346,37.2631014686576,38.1264711628116));
#21749=CARTESIAN_POINT('Ctrl Pts',(-41.7981279794346,37.2631014686576,38.1264711628116));
#21750=CARTESIAN_POINT('Ctrl Pts',(-41.7981279794346,37.2631014686576,38.1264711628116));
#21751=CARTESIAN_POINT('Ctrl Pts',(-41.7981279794346,37.2631014686576,38.1264711628116));
#21752=CARTESIAN_POINT('Ctrl Pts',(-41.7981279794346,37.2631014686576,38.1264711628116));
#21753=CARTESIAN_POINT('Ctrl Pts',(-41.7981279794346,37.2631014686576,38.1264711628116));
#21754=CARTESIAN_POINT('Ctrl Pts',(-41.7981279794346,37.2631014686576,38.1264711628116));
#21755=CARTESIAN_POINT('Ctrl Pts',(-41.7981279794346,37.2631014686576,38.1264711628116));
#21756=CARTESIAN_POINT('Ctrl Pts',(-41.7981279794346,37.2631014686576,38.1264711628116));
#21757=CARTESIAN_POINT('Ctrl Pts',(-41.7981279794346,37.2631014686576,38.1264711628116));
#21758=CARTESIAN_POINT('Ctrl Pts',(-41.7981279794346,37.2631014686576,38.1264711628116));
#21759=CARTESIAN_POINT('Ctrl Pts',(-41.7981279794346,37.2631014686576,38.1264711628116));
#21760=CARTESIAN_POINT('Ctrl Pts',(-41.7981279794346,37.2631014686576,38.1264711628116));
#21761=CARTESIAN_POINT('Ctrl Pts',(-41.7981279794346,37.2631014686576,38.1264711628116));
#21762=CARTESIAN_POINT('Ctrl Pts',(-41.7981279794346,37.2631014686576,38.1264711628116));
#21763=CARTESIAN_POINT('Ctrl Pts',(-41.7981279794346,37.2631014686576,38.1264711628116));
#21764=CARTESIAN_POINT('Ctrl Pts',(-41.7981279794346,37.2631014686576,38.1264711628116));
#21765=CARTESIAN_POINT('Ctrl Pts',(-41.7903142026293,37.2533591778441,38.1177800387672));
#21766=CARTESIAN_POINT('Ctrl Pts',(-41.7904177506121,37.2535524312197,38.1179992662862));
#21767=CARTESIAN_POINT('Ctrl Pts',(-41.790521298595,37.2537456845954,38.1182184938053));
#21768=CARTESIAN_POINT('Ctrl Pts',(-41.7906248465778,37.253938937971,38.1184377213244));
#21769=CARTESIAN_POINT('Ctrl Pts',(-41.7907283026149,37.2541320197466,38.1186567541796));
#21770=CARTESIAN_POINT('Ctrl Pts',(-41.790831758652,37.2543251015223,38.1188757870348));
#21771=CARTESIAN_POINT('Ctrl Pts',(-41.790935214689,37.2545181832979,38.1190948198901));
#21772=CARTESIAN_POINT('Ctrl Pts',(-41.7910386707261,37.2547112650735,38.1193138527453));
#21773=CARTESIAN_POINT('Ctrl Pts',(-41.7911421267631,37.2549043468491,38.1195328856005));
#21774=CARTESIAN_POINT('Ctrl Pts',(-41.7912455828002,37.2550974286247,38.1197519184557));
#21775=CARTESIAN_POINT('Ctrl Pts',(-41.7913490388372,37.2552905104004,38.1199709513109));
#21776=CARTESIAN_POINT('Ctrl Pts',(-41.7914524948743,37.255483592176,38.1201899841661));
#21777=CARTESIAN_POINT('Ctrl Pts',(-41.7915559509113,37.2556766739516,38.1204090170214));
#21778=CARTESIAN_POINT('Ctrl Pts',(-41.7916594069484,37.2558697557272,38.1206280498766));
#21779=CARTESIAN_POINT('Ctrl Pts',(-41.7917628629855,37.2560628375028,38.1208470827318));
#21780=CARTESIAN_POINT('Ctrl Pts',(-41.7918663190225,37.2562559192784,38.121066115587));
#21781=CARTESIAN_POINT('Ctrl Pts',(-41.7919697750596,37.2564490010541,38.1212851484422));
#21782=CARTESIAN_POINT('Ctrl Pts',(-41.7920732310966,37.2566420828297,38.1215041812975));
#21783=CARTESIAN_POINT('Ctrl Pts',(-41.7921766871337,37.2568351646053,38.1217232141527));
#21784=CARTESIAN_POINT('Ctrl Pts',(-41.7922801431707,37.2570282463809,38.1219422470079));
#21785=CARTESIAN_POINT('Ctrl Pts',(-41.7923835992078,37.2572213281565,38.1221612798631));
#21786=CARTESIAN_POINT('Ctrl Pts',(-41.7924870552448,37.2574144099322,38.1223803127183));
#21787=CARTESIAN_POINT('Ctrl Pts',(-41.7925905112819,37.2576074917078,38.1225993455735));
#21788=CARTESIAN_POINT('Ctrl Pts',(-41.792693967319,37.2578005734834,38.1228183784288));
#21789=CARTESIAN_POINT('Ctrl Pts',(-41.792797423356,37.257993655259,38.123037411284));
#21790=CARTESIAN_POINT('Ctrl Pts',(-41.7929008793931,37.2581867370346,38.1232564441392));
#21791=CARTESIAN_POINT('Ctrl Pts',(-41.7930043354301,37.2583798188103,38.1234754769944));
#21792=CARTESIAN_POINT('Ctrl Pts',(-41.7931077914672,37.2585729005859,38.1236945098496));
#21793=CARTESIAN_POINT('Ctrl Pts',(-41.7932112475042,37.2587659823615,38.1239135427048));
#21794=CARTESIAN_POINT('Ctrl Pts',(-41.7933147035413,37.2589590641371,38.1241325755601));
#21795=CARTESIAN_POINT('Ctrl Pts',(-41.7934181595783,37.2591521459127,38.1243516084153));
#21796=CARTESIAN_POINT('Ctrl Pts',(-41.7935216156154,37.2593452276883,38.1245706412705));
#21797=CARTESIAN_POINT('Ctrl Pts',(-41.7936250716524,37.259538309464,38.1247896741257));
#21798=CARTESIAN_POINT('Ctrl Pts',(-41.7937285276895,37.2597313912396,38.1250087069809));
#21799=CARTESIAN_POINT('Ctrl Pts',(-41.7938319837265,37.2599244730152,38.1252277398362));
#21800=CARTESIAN_POINT('Ctrl Pts',(-41.7939354397636,37.2601175547908,38.1254467726914));
#21801=CARTESIAN_POINT('Ctrl Pts',(-41.7940388958007,37.2603106365664,38.1256658055466));
#21802=CARTESIAN_POINT('Ctrl Pts',(-41.7941423518377,37.2605037183421,38.1258848384018));
#21803=CARTESIAN_POINT('Ctrl Pts',(-41.7942458078748,37.2606968001177,38.126103871257));
#21804=CARTESIAN_POINT('Ctrl Pts',(-41.7943492639118,37.2608898818933,38.1263229041122));
#21805=CARTESIAN_POINT('Ctrl Pts',(-41.7944527199489,37.2610829636689,38.1265419369675));
#21806=CARTESIAN_POINT('Ctrl Pts',(-41.7945561759859,37.2612760454445,38.1267609698227));
#21807=CARTESIAN_POINT('Ctrl Pts',(-41.794659632023,37.2614691272201,38.1269800026779));
#21808=CARTESIAN_POINT('Ctrl Pts',(-41.7947630880601,37.2616622089958,38.1271990355331));
#21809=CARTESIAN_POINT('Ctrl Pts',(-41.7948665440971,37.2618552907714,38.1274180683883));
#21810=CARTESIAN_POINT('Ctrl Pts',(-41.7949700001342,37.262048372547,38.1276371012436));
#21811=CARTESIAN_POINT('Ctrl Pts',(-41.7950734561712,37.2622414543226,38.1278561340988));
#21812=CARTESIAN_POINT('Ctrl Pts',(-41.7951769122083,37.2624345360982,38.128075166954));
#21813=CARTESIAN_POINT('Ctrl Pts',(-41.7952803682453,37.2626276178739,38.1282941998092));
#21814=CARTESIAN_POINT('Ctrl Pts',(-41.7821095414117,37.2432764801138,38.1087531709748));
#21815=CARTESIAN_POINT('Ctrl Pts',(-41.7823253824494,37.2436690259226,38.1091992802783));
#21816=CARTESIAN_POINT('Ctrl Pts',(-41.7825411862613,37.2440616379331,38.1096453486643));
#21817=CARTESIAN_POINT('Ctrl Pts',(-41.7827569528505,37.244454316149,38.1100913761369));
#21818=CARTESIAN_POINT('Ctrl Pts',(-41.7829725278491,37.2448466456847,38.1105370075579));
#21819=CARTESIAN_POINT('Ctrl Pts',(-41.783188065691,37.2452390413084,38.1109825981382));
#21820=CARTESIAN_POINT('Ctrl Pts',(-41.7834035663794,37.2456315030234,38.111428147882));
#21821=CARTESIAN_POINT('Ctrl Pts',(-41.7836190670678,37.2460239647385,38.1118736976259));
#21822=CARTESIAN_POINT('Ctrl Pts',(-41.7838345306026,37.246416492545,38.1123192065333));
#21823=CARTESIAN_POINT('Ctrl Pts',(-41.7840499569867,37.2468090864466,38.1127646746086));
#21824=CARTESIAN_POINT('Ctrl Pts',(-41.7842653833709,37.2472016803483,38.1132101426838));
#21825=CARTESIAN_POINT('Ctrl Pts',(-41.7844807726045,37.247594340345,38.1136555699269));
#21826=CARTESIAN_POINT('Ctrl Pts',(-41.7846961246904,37.2479870664405,38.114100956342));
#21827=CARTESIAN_POINT('Ctrl Pts',(-41.7849114767764,37.248379792536,38.1145463427572));
#21828=CARTESIAN_POINT('Ctrl Pts',(-41.7851267917147,37.2487725847303,38.1149916883443));
#21829=CARTESIAN_POINT('Ctrl Pts',(-41.7853420695084,37.2491654430271,38.1154369931077));
#21830=CARTESIAN_POINT('Ctrl Pts',(-41.7855573473021,37.2495583013238,38.1158822978712));
#21831=CARTESIAN_POINT('Ctrl Pts',(-41.7857725879511,37.2499512257232,38.1163275618108));
#21832=CARTESIAN_POINT('Ctrl Pts',(-41.7859877914583,37.2503442162287,38.1167727849309));
#21833=CARTESIAN_POINT('Ctrl Pts',(-41.7862029949656,37.2507372067343,38.117218008051));
#21834=CARTESIAN_POINT('Ctrl Pts',(-41.7864181613311,37.251130263346,38.1176631903516));
#21835=CARTESIAN_POINT('Ctrl Pts',(-41.7866332905579,37.2515233860677,38.1181083318368));
#21836=CARTESIAN_POINT('Ctrl Pts',(-41.7868484197847,37.2519165087895,38.1185534733219));
#21837=CARTESIAN_POINT('Ctrl Pts',(-41.7870635118726,37.2523096976213,38.1189985739917));
#21838=CARTESIAN_POINT('Ctrl Pts',(-41.7872785668247,37.2527029525669,38.1194436338503));
#21839=CARTESIAN_POINT('Ctrl Pts',(-41.7874936217768,37.2530962075124,38.1198886937088));
#21840=CARTESIAN_POINT('Ctrl Pts',(-41.787708639593,37.2534895285718,38.1203337127562));
#21841=CARTESIAN_POINT('Ctrl Pts',(-41.7879236202762,37.2538829157488,38.1207786909964));
#21842=CARTESIAN_POINT('Ctrl Pts',(-41.7881386009594,37.2542763029258,38.1212236692367));
#21843=CARTESIAN_POINT('Ctrl Pts',(-41.7883535445096,37.2546697562204,38.1216686066698));
#21844=CARTESIAN_POINT('Ctrl Pts',(-41.7885684509297,37.2550632756365,38.1221135033));
#21845=CARTESIAN_POINT('Ctrl Pts',(-41.7887833573499,37.2554567950526,38.1225583999302));
#21846=CARTESIAN_POINT('Ctrl Pts',(-41.7889982266399,37.2558503805902,38.1230032557575));
#21847=CARTESIAN_POINT('Ctrl Pts',(-41.7892130588027,37.2562440322531,38.1234480707859));
#21848=CARTESIAN_POINT('Ctrl Pts',(-41.7894278909654,37.2566376839161,38.1238928858142));
#21849=CARTESIAN_POINT('Ctrl Pts',(-41.789642686001,37.2570314017044,38.1243376600438));
#21850=CARTESIAN_POINT('Ctrl Pts',(-41.7898574439121,37.2574251856219,38.1247823934785));
#21851=CARTESIAN_POINT('Ctrl Pts',(-41.7900722018233,37.2578189695394,38.1252271269133));
#21852=CARTESIAN_POINT('Ctrl Pts',(-41.79028692261,37.2582128195863,38.1256718195533));
#21853=CARTESIAN_POINT('Ctrl Pts',(-41.7905016062752,37.2586067357663,38.1261164714026));
#21854=CARTESIAN_POINT('Ctrl Pts',(-41.7907162899404,37.2590006519463,38.1265611232519));
#21855=CARTESIAN_POINT('Ctrl Pts',(-41.7909309364841,37.2593946342595,38.1270057343105));
#21856=CARTESIAN_POINT('Ctrl Pts',(-41.791145545909,37.2597886827099,38.1274503045824));
#21857=CARTESIAN_POINT('Ctrl Pts',(-41.7913601553339,37.2601827311602,38.1278948748544));
#21858=CARTESIAN_POINT('Ctrl Pts',(-41.7915747276401,37.2605768457478,38.1283394043397));
#21859=CARTESIAN_POINT('Ctrl Pts',(-41.7917892628303,37.2609710264765,38.1287838930424));
#21860=CARTESIAN_POINT('Ctrl Pts',(-41.7920037980206,37.2613652072052,38.1292283817452));
#21861=CARTESIAN_POINT('Ctrl Pts',(-41.7922182960949,37.2617594540751,38.1296728296653));
#21862=CARTESIAN_POINT('Ctrl Pts',(-41.7924327570561,37.2621537670901,38.1301172368068));
#21863=CARTESIAN_POINT('Ctrl Pts',(-41.7734797039072,37.2328485512714,38.0993780694756));
#21864=CARTESIAN_POINT('Ctrl Pts',(-41.7738174367737,37.2334462429607,38.1000591182637));
#21865=CARTESIAN_POINT('Ctrl Pts',(-41.7741550496373,37.2340441517543,38.100740036031));
#21866=CARTESIAN_POINT('Ctrl Pts',(-41.7744925424411,37.2346422775518,38.1014208226628));
#21867=CARTESIAN_POINT('Ctrl Pts',(-41.7748297355669,37.2352398722414,38.1021010047876));
#21868=CARTESIAN_POINT('Ctrl Pts',(-41.775166808846,37.2358376835495,38.1027810560098));
#21869=CARTESIAN_POINT('Ctrl Pts',(-41.7755037622217,37.2364357113757,38.103460976215));
#21870=CARTESIAN_POINT('Ctrl Pts',(-41.7758407155975,37.2370337392019,38.1041408964203));
#21871=CARTESIAN_POINT('Ctrl Pts',(-41.7761775490699,37.2376319835463,38.1048206856085));
#21872=CARTESIAN_POINT('Ctrl Pts',(-41.7765142625823,37.2382304443082,38.1055003436656));
#21873=CARTESIAN_POINT('Ctrl Pts',(-41.7768509760948,37.2388289050702,38.1061800017226));
#21874=CARTESIAN_POINT('Ctrl Pts',(-41.7771875696473,37.2394275822497,38.1068595286485));
#21875=CARTESIAN_POINT('Ctrl Pts',(-41.7775240431833,37.2400264757463,38.1075389243291));
#21876=CARTESIAN_POINT('Ctrl Pts',(-41.7778605167192,37.2406253692429,38.1082183200096));
#21877=CARTESIAN_POINT('Ctrl Pts',(-41.7781968702387,37.2412244790565,38.1088975844447));
#21878=CARTESIAN_POINT('Ctrl Pts',(-41.7785331036852,37.2418238050864,38.1095767175204));
#21879=CARTESIAN_POINT('Ctrl Pts',(-41.7788693371317,37.2424231311163,38.1102558505961));
#21880=CARTESIAN_POINT('Ctrl Pts',(-41.7792054505051,37.2430226733626,38.1109348523123));
#21881=CARTESIAN_POINT('Ctrl Pts',(-41.7795414437491,37.2436224317244,38.1116137225549));
#21882=CARTESIAN_POINT('Ctrl Pts',(-41.779877436993,37.2442221900863,38.1122925927975));
#21883=CARTESIAN_POINT('Ctrl Pts',(-41.7802133101075,37.2448221645638,38.1129713315665));
#21884=CARTESIAN_POINT('Ctrl Pts',(-41.7805490630361,37.245422355056,38.113649938748));
#21885=CARTESIAN_POINT('Ctrl Pts',(-41.7808848159646,37.2460225455484,38.1143285459293));
#21886=CARTESIAN_POINT('Ctrl Pts',(-41.7812204487072,37.2466229520555,38.1150070215231));
#21887=CARTESIAN_POINT('Ctrl Pts',(-41.7815559612075,37.2472235744765,38.1156853654153));
#21888=CARTESIAN_POINT('Ctrl Pts',(-41.7818914737078,37.2478241968974,38.1163637093074));
#21889=CARTESIAN_POINT('Ctrl Pts',(-41.7822268659657,37.2484250352323,38.117041921498));
#21890=CARTESIAN_POINT('Ctrl Pts',(-41.782562137925,37.2490260893802,38.1177200018729));
#21891=CARTESIAN_POINT('Ctrl Pts',(-41.7828974098843,37.2496271435281,38.1183980822478));
#21892=CARTESIAN_POINT('Ctrl Pts',(-41.7832325615449,37.250228413489,38.1190760308072));
#21893=CARTESIAN_POINT('Ctrl Pts',(-41.7835675928505,37.2508298991617,38.1197538474371));
#21894=CARTESIAN_POINT('Ctrl Pts',(-41.7839026241561,37.2514313848345,38.120431664067));
#21895=CARTESIAN_POINT('Ctrl Pts',(-41.7842375351068,37.2520330862192,38.1211093487674));
#21896=CARTESIAN_POINT('Ctrl Pts',(-41.7845723256461,37.2526350032147,38.1217869014244));
#21897=CARTESIAN_POINT('Ctrl Pts',(-41.7849071161855,37.2532369202102,38.1224644540814));
#21898=CARTESIAN_POINT('Ctrl Pts',(-41.7852417863136,37.2538390528166,38.1231418746951));
#21899=CARTESIAN_POINT('Ctrl Pts',(-41.7855763359742,37.2544414009326,38.1238191631516));
#21900=CARTESIAN_POINT('Ctrl Pts',(-41.7859108856348,37.2550437490486,38.1244964516081));
#21901=CARTESIAN_POINT('Ctrl Pts',(-41.7862453148279,37.2556463126744,38.1251736079073));
#21902=CARTESIAN_POINT('Ctrl Pts',(-41.7865796234973,37.2562490917085,38.1258506319357));
#21903=CARTESIAN_POINT('Ctrl Pts',(-41.7869139321667,37.2568518707426,38.126527655964));
#21904=CARTESIAN_POINT('Ctrl Pts',(-41.7872481203125,37.257454865185,38.1272045477214));
#21905=CARTESIAN_POINT('Ctrl Pts',(-41.7875821878784,37.2580580749346,38.1278813070941));
#21906=CARTESIAN_POINT('Ctrl Pts',(-41.7879162554443,37.2586612846843,38.1285580664668));
#21907=CARTESIAN_POINT('Ctrl Pts',(-41.7882502024303,37.259264709741,38.1292346934548));
#21908=CARTESIAN_POINT('Ctrl Pts',(-41.7885840287804,37.2598683500034,38.1299111879444));
#21909=CARTESIAN_POINT('Ctrl Pts',(-41.7889178551305,37.2604719902658,38.130587682434));
#21910=CARTESIAN_POINT('Ctrl Pts',(-41.7892515608447,37.2610758457339,38.1312640444252));
#21911=CARTESIAN_POINT('Ctrl Pts',(-41.7895851458668,37.2616799163063,38.1319402738044));
#21912=CARTESIAN_POINT('Ctrl Pts',(-41.771322244531,37.2302415690607,38.0970342941008));
#21913=CARTESIAN_POINT('Ctrl Pts',(-41.7716904503549,37.2308905472201,38.0977740777601));
#21914=CARTESIAN_POINT('Ctrl Pts',(-41.7720585154814,37.2315397802096,38.0985137078727));
#21915=CARTESIAN_POINT('Ctrl Pts',(-41.7724264398387,37.2321892679025,38.0992531842943));
#21916=CARTESIAN_POINT('Ctrl Pts',(-41.7727940374963,37.2328381788805,38.0999920040951));
#21917=CARTESIAN_POINT('Ctrl Pts',(-41.7731614946347,37.2334873441097,38.1007306704778));
#21918=CARTESIAN_POINT('Ctrl Pts',(-41.7735288111823,37.2341367634638,38.1014691832983));
#21919=CARTESIAN_POINT('Ctrl Pts',(-41.7738961277299,37.2347861828177,38.1022076961189));
#21920=CARTESIAN_POINT('Ctrl Pts',(-41.7742633036867,37.2354358562966,38.1029460553773));
#21921=CARTESIAN_POINT('Ctrl Pts',(-41.7746303389812,37.2360857837736,38.1036842609298));
#21922=CARTESIAN_POINT('Ctrl Pts',(-41.7749973742757,37.2367357112507,38.1044224664823));
#21923=CARTESIAN_POINT('Ctrl Pts',(-41.7753642689079,37.2373858927259,38.1051605183289));
#21924=CARTESIAN_POINT('Ctrl Pts',(-41.7757310228065,37.2380363280728,38.1058984163258));
#21925=CARTESIAN_POINT('Ctrl Pts',(-41.776097776705,37.2386867634196,38.1066363143227));
#21926=CARTESIAN_POINT('Ctrl Pts',(-41.7764643898697,37.239337452638,38.1073740584699));
#21927=CARTESIAN_POINT('Ctrl Pts',(-41.7768308622294,37.2399883956012,38.1081116486236));
#21928=CARTESIAN_POINT('Ctrl Pts',(-41.7771973345891,37.2406393385644,38.1088492387774));
#21929=CARTESIAN_POINT('Ctrl Pts',(-41.7775636661437,37.2412905352724,38.1095866749377));
#21930=CARTESIAN_POINT('Ctrl Pts',(-41.7779298568218,37.2419419855984,38.1103239569609));
#21931=CARTESIAN_POINT('Ctrl Pts',(-41.7782960474999,37.2425934359243,38.1110612389841));
#21932=CARTESIAN_POINT('Ctrl Pts',(-41.7786620973016,37.2432451398683,38.1117983668703));
#21933=CARTESIAN_POINT('Ctrl Pts',(-41.7790280061556,37.2438970973032,38.1125353404757));
#21934=CARTESIAN_POINT('Ctrl Pts',(-41.7793939150096,37.2445490547381,38.1132723140812));
#21935=CARTESIAN_POINT('Ctrl Pts',(-41.7797596829158,37.245201265664,38.114009133406));
#21936=CARTESIAN_POINT('Ctrl Pts',(-41.7801253098032,37.2458537299538,38.1147457983065));
#21937=CARTESIAN_POINT('Ctrl Pts',(-41.7804909366905,37.2465061942437,38.1154824632071));
#21938=CARTESIAN_POINT('Ctrl Pts',(-41.7808564225589,37.2471589118975,38.1162189736834));
#21939=CARTESIAN_POINT('Ctrl Pts',(-41.7812217673372,37.247811882788,38.1169553295921));
#21940=CARTESIAN_POINT('Ctrl Pts',(-41.7815871121155,37.2484648536787,38.1176916855007));
#21941=CARTESIAN_POINT('Ctrl Pts',(-41.7819523158038,37.249118077806,38.1184278868416));
#21942=CARTESIAN_POINT('Ctrl Pts',(-41.7823173783307,37.249771555043,38.1191639334714));
#21943=CARTESIAN_POINT('Ctrl Pts',(-41.7826824408577,37.2504250322799,38.1198999801012));
#21944=CARTESIAN_POINT('Ctrl Pts',(-41.7830473622235,37.2510787626264,38.1206358720198));
#21945=CARTESIAN_POINT('Ctrl Pts',(-41.783412142357,37.2517327459551,38.121371609084));
#21946=CARTESIAN_POINT('Ctrl Pts',(-41.7837769224905,37.2523867292838,38.1221073461482));
#21947=CARTESIAN_POINT('Ctrl Pts',(-41.7841415613918,37.2530409655946,38.1228429283579));
#21948=CARTESIAN_POINT('Ctrl Pts',(-41.7845060589897,37.2536954547603,38.1235783555698));
#21949=CARTESIAN_POINT('Ctrl Pts',(-41.7848705565877,37.254349943926,38.1243137827817));
#21950=CARTESIAN_POINT('Ctrl Pts',(-41.7852349128824,37.2550046859463,38.1250490549959));
#21951=CARTESIAN_POINT('Ctrl Pts',(-41.7855991278029,37.255659680694,38.125784172069));
#21952=CARTESIAN_POINT('Ctrl Pts',(-41.7859633427234,37.2563146754416,38.1265192891421));
#21953=CARTESIAN_POINT('Ctrl Pts',(-41.7863274162696,37.2569699229165,38.1272542510741));
#21954=CARTESIAN_POINT('Ctrl Pts',(-41.7866913483708,37.2576254229908,38.127989057722));
#21955=CARTESIAN_POINT('Ctrl Pts',(-41.7870552804719,37.2582809230653,38.1287238643699));
#21956=CARTESIAN_POINT('Ctrl Pts',(-41.7874190711279,37.2589366757393,38.1294585157335));
#21957=CARTESIAN_POINT('Ctrl Pts',(-41.787782720268,37.2595926808851,38.1301930116699));
#21958=CARTESIAN_POINT('Ctrl Pts',(-41.788146369408,37.260248686031,38.1309275076062));
#21959=CARTESIAN_POINT('Ctrl Pts',(-41.7885098770322,37.2609049436486,38.1316618481152));
#21960=CARTESIAN_POINT('Ctrl Pts',(-41.7888732430695,37.2615614536103,38.1323960330538));
#21961=CARTESIAN_POINT('Ctrl Pts',(-41.7691382140772,37.2276131212637,38.0946687739682));
#21962=CARTESIAN_POINT('Ctrl Pts',(-41.7695374927977,37.2283137491982,38.095467795755));
#21963=CARTESIAN_POINT('Ctrl Pts',(-41.7699366072763,37.2290146749967,38.0962666383926));
#21964=CARTESIAN_POINT('Ctrl Pts',(-41.7703355574223,37.2297158984997,38.097065301699));
#21965=CARTESIAN_POINT('Ctrl Pts',(-41.770734153319,37.2304164993487,38.0978632558295));
#21966=CARTESIAN_POINT('Ctrl Pts',(-41.7711325851747,37.2311173973738,38.0986610309469));
#21967=CARTESIAN_POINT('Ctrl Pts',(-41.7715308528989,37.2318185924153,38.0994586268701));
#21968=CARTESIAN_POINT('Ctrl Pts',(-41.7719291206231,37.2325197874568,38.1002562227932));
#21969=CARTESIAN_POINT('Ctrl Pts',(-41.7723272242156,37.2332212795149,38.1010536395219));
#21970=CARTESIAN_POINT('Ctrl Pts',(-41.7727251635862,37.2339230684298,38.1018508768749));
#21971=CARTESIAN_POINT('Ctrl Pts',(-41.7731231029567,37.2346248573449,38.1026481142279));
#21972=CARTESIAN_POINT('Ctrl Pts',(-41.7735208781052,37.2353269431168,38.1034451722051));
#21973=CARTESIAN_POINT('Ctrl Pts',(-41.7739184889412,37.236029325586,38.1042420506252));
#21974=CARTESIAN_POINT('Ctrl Pts',(-41.7743160997773,37.2367317080551,38.1050389290454));
#21975=CARTESIAN_POINT('Ctrl Pts',(-41.7747135463009,37.2374343872215,38.1058356279085));
#21976=CARTESIAN_POINT('Ctrl Pts',(-41.7751108284216,37.2381373629254,38.1066321470333));
#21977=CARTESIAN_POINT('Ctrl Pts',(-41.7755081105424,37.2388403386292,38.1074286661581));
#21978=CARTESIAN_POINT('Ctrl Pts',(-41.7759052282603,37.2395436108705,38.1082250055445));
#21979=CARTESIAN_POINT('Ctrl Pts',(-41.7763021814853,37.2402471794891,38.1090211650117));
#21980=CARTESIAN_POINT('Ctrl Pts',(-41.7766991347102,37.2409507481079,38.1098173244787));
#21981=CARTESIAN_POINT('Ctrl Pts',(-41.777095923442,37.241654613104,38.1106133040264));
#21982=CARTESIAN_POINT('Ctrl Pts',(-41.7774925475906,37.2423587743175,38.1114091034736));
#21983=CARTESIAN_POINT('Ctrl Pts',(-41.7778891717392,37.2430629355309,38.1122049029208));
#21984=CARTESIAN_POINT('Ctrl Pts',(-41.7782856313045,37.2437673929618,38.1130005222675));
#21985=CARTESIAN_POINT('Ctrl Pts',(-41.7786819261965,37.2444721464497,38.1137959613327));
#21986=CARTESIAN_POINT('Ctrl Pts',(-41.7790782210884,37.2451768999376,38.114591400398));
#21987=CARTESIAN_POINT('Ctrl Pts',(-41.7794743513071,37.2458819494826,38.1153866591818));
#21988=CARTESIAN_POINT('Ctrl Pts',(-41.7798703167622,37.2465872949244,38.1161817375032));
#21989=CARTESIAN_POINT('Ctrl Pts',(-41.7802662822174,37.2472926403662,38.1169768158246));
#21990=CARTESIAN_POINT('Ctrl Pts',(-41.7806620829091,37.2479982817048,38.1177717136837));
#21991=CARTESIAN_POINT('Ctrl Pts',(-41.7810577187476,37.2487042187795,38.1185664308996));
#21992=CARTESIAN_POINT('Ctrl Pts',(-41.7814533545859,37.2494101558543,38.1193611481155));
#21993=CARTESIAN_POINT('Ctrl Pts',(-41.7818488255709,37.2501163886654,38.1201556846882));
#21994=CARTESIAN_POINT('Ctrl Pts',(-41.7822441316126,37.250822917052,38.1209500404371));
#21995=CARTESIAN_POINT('Ctrl Pts',(-41.7826394376543,37.2515294454386,38.1217443961859));
#21996=CARTESIAN_POINT('Ctrl Pts',(-41.7830345787528,37.2522362694009,38.1225385711109));
#21997=CARTESIAN_POINT('Ctrl Pts',(-41.7834295548181,37.252943388778,38.1233325650312));
#21998=CARTESIAN_POINT('Ctrl Pts',(-41.7838245308834,37.2536505081552,38.1241265589516));
#21999=CARTESIAN_POINT('Ctrl Pts',(-41.7842193419157,37.2543579229471,38.1249203718674));
#22000=CARTESIAN_POINT('Ctrl Pts',(-41.7846139878251,37.255065632993,38.1257140035981));
#22001=CARTESIAN_POINT('Ctrl Pts',(-41.7850086337345,37.255773343039,38.1265076353288));
#22002=CARTESIAN_POINT('Ctrl Pts',(-41.785403114521,37.2564813483389,38.1273010858744));
#22003=CARTESIAN_POINT('Ctrl Pts',(-41.785797430095,37.2571896487317,38.1280943550543));
#22004=CARTESIAN_POINT('Ctrl Pts',(-41.7861917456691,37.2578979491245,38.1288876242342));
#22005=CARTESIAN_POINT('Ctrl Pts',(-41.7865858960306,37.2586065446103,38.1296807120485));
#22006=CARTESIAN_POINT('Ctrl Pts',(-41.78697988109,37.2593154350278,38.1304736183168));
#22007=CARTESIAN_POINT('Ctrl Pts',(-41.7873738661493,37.2600243254453,38.1312665245851));
#22008=CARTESIAN_POINT('Ctrl Pts',(-41.7877676859066,37.2607335107946,38.1320592493073));
#22009=CARTESIAN_POINT('Ctrl Pts',(-41.7881613402722,37.2614429909144,38.1328517923032));
#22010=CARTESIAN_POINT('Ctrl Pts',(-41.766927213444,37.2249631469137,38.0922814953632));
#22011=CARTESIAN_POINT('Ctrl Pts',(-41.7673581756058,37.2257157843197,38.0931402611643));
#22012=CARTESIAN_POINT('Ctrl Pts',(-41.7677889469959,37.2264687682492,38.0939988190038));
#22013=CARTESIAN_POINT('Ctrl Pts',(-41.7682195274985,37.2272220985005,38.0948571686514));
#22014=CARTESIAN_POINT('Ctrl Pts',(-41.7686497256657,37.2279747598295,38.0957147561243));
#22015=CARTESIAN_POINT('Ctrl Pts',(-41.7690797332845,37.2287277668655,38.0965721357748));
#22016=CARTESIAN_POINT('Ctrl Pts',(-41.7695095502396,37.2294811194068,38.0974293073736));
#22017=CARTESIAN_POINT('Ctrl Pts',(-41.7699393671947,37.2302344719482,38.0982864789723));
#22018=CARTESIAN_POINT('Ctrl Pts',(-41.7703689934863,37.2309881699949,38.0991434425192));
#22019=CARTESIAN_POINT('Ctrl Pts',(-41.7707984289993,37.2317422133453,38.1000001977849));
#22020=CARTESIAN_POINT('Ctrl Pts',(-41.7712278645123,37.2324962566957,38.1008569530506));
#22021=CARTESIAN_POINT('Ctrl Pts',(-41.7716571092468,37.2332506453498,38.101713500035));
#22022=CARTESIAN_POINT('Ctrl Pts',(-41.7720861630878,37.2340053791055,38.102569838509));
#22023=CARTESIAN_POINT('Ctrl Pts',(-41.7725152169288,37.2347601128614,38.103426176983));
#22024=CARTESIAN_POINT('Ctrl Pts',(-41.7729440798763,37.2355151917189,38.1042823069466));
#22025=CARTESIAN_POINT('Ctrl Pts',(-41.7733727518156,37.236270615476,38.1051382281704));
#22026=CARTESIAN_POINT('Ctrl Pts',(-41.7738014237548,37.2370260392332,38.1059941493943));
#22027=CARTESIAN_POINT('Ctrl Pts',(-41.7742299046859,37.23778180789,38.1068498618786));
#22028=CARTESIAN_POINT('Ctrl Pts',(-41.774658194494,37.2385379212441,38.1077053653942));
#22029=CARTESIAN_POINT('Ctrl Pts',(-41.775086484302,37.2392940345982,38.1085608689097));
#22030=CARTESIAN_POINT('Ctrl Pts',(-41.7755145829872,37.2400504926497,38.1094161634566));
#22031=CARTESIAN_POINT('Ctrl Pts',(-41.7759424904348,37.240807295196,38.1102712488059));
#22032=CARTESIAN_POINT('Ctrl Pts',(-41.7763703978824,37.2415640977423,38.1111263341552));
#22033=CARTESIAN_POINT('Ctrl Pts',(-41.7767981140925,37.2423212447835,38.1119812103068));
#22034=CARTESIAN_POINT('Ctrl Pts',(-41.7772256389506,37.2430787361169,38.1128358770321));
#22035=CARTESIAN_POINT('Ctrl Pts',(-41.7776531638086,37.2438362274503,38.1136905437573));
#22036=CARTESIAN_POINT('Ctrl Pts',(-41.7780804973147,37.2445940630758,38.1145450010561));
#22037=CARTESIAN_POINT('Ctrl Pts',(-41.7785076393544,37.2453522427908,38.1153992486998));
#22038=CARTESIAN_POINT('Ctrl Pts',(-41.7789347813941,37.2461104225057,38.1162534963434));
#22039=CARTESIAN_POINT('Ctrl Pts',(-41.7793617319673,37.24686894631,38.117107534332));
#22040=CARTESIAN_POINT('Ctrl Pts',(-41.7797884909599,37.2476278140006,38.1179613624368));
#22041=CARTESIAN_POINT('Ctrl Pts',(-41.7802152499525,37.2483866816912,38.1188151905415));
#22042=CARTESIAN_POINT('Ctrl Pts',(-41.7806418173644,37.2491458932681,38.1196688087626));
#22043=CARTESIAN_POINT('Ctrl Pts',(-41.7810681930815,37.2499054485281,38.1205222168715));
#22044=CARTESIAN_POINT('Ctrl Pts',(-41.7814945687986,37.2506650037881,38.1213756249803));
#22045=CARTESIAN_POINT('Ctrl Pts',(-41.7819207528208,37.2514249027313,38.122228822977));
#22046=CARTESIAN_POINT('Ctrl Pts',(-41.7823467450341,37.2521851451541,38.123081810633));
#22047=CARTESIAN_POINT('Ctrl Pts',(-41.7827727372475,37.2529453875769,38.123934798289));
#22048=CARTESIAN_POINT('Ctrl Pts',(-41.7831985376518,37.2537059734796,38.1247875756044));
#22049=CARTESIAN_POINT('Ctrl Pts',(-41.7836241461333,37.2544669026582,38.125640142351));
#22050=CARTESIAN_POINT('Ctrl Pts',(-41.7840497546148,37.2552278318368,38.1264927090977));
#22051=CARTESIAN_POINT('Ctrl Pts',(-41.7844751711734,37.2559891042917,38.1273450652754));
#22052=CARTESIAN_POINT('Ctrl Pts',(-41.7849003956952,37.2567507198189,38.1281972106561));
#22053=CARTESIAN_POINT('Ctrl Pts',(-41.785325620217,37.257512335346,38.1290493560369));
#22054=CARTESIAN_POINT('Ctrl Pts',(-41.7857506527021,37.2582742939455,38.1299012906207));
#22055=CARTESIAN_POINT('Ctrl Pts',(-41.7861754930366,37.2590365954135,38.1307530141794));
#22056=CARTESIAN_POINT('Ctrl Pts',(-41.7866003333711,37.2597988968814,38.1316047377382));
#22057=CARTESIAN_POINT('Ctrl Pts',(-41.7870249815551,37.2605615412178,38.1324562502719));
#22058=CARTESIAN_POINT('Ctrl Pts',(-41.7874494374749,37.2613245282184,38.1333075515526));
#22059=CARTESIAN_POINT('Ctrl Pts',(-41.7658217131275,37.2236381597387,38.0910878560607));
#22060=CARTESIAN_POINT('Ctrl Pts',(-41.7662685170099,37.2244168018805,38.091976493869));
#22061=CARTESIAN_POINT('Ctrl Pts',(-41.7667151168556,37.2251958148755,38.0928649093094));
#22062=CARTESIAN_POINT('Ctrl Pts',(-41.7671615125367,37.2259751985009,38.0937531021275));
#22063=CARTESIAN_POINT('Ctrl Pts',(-41.7676075118391,37.2267538900699,38.0946405062717));
#22064=CARTESIAN_POINT('Ctrl Pts',(-41.7680533073393,37.2275329516114,38.0955276881887));
#22065=CARTESIAN_POINT('Ctrl Pts',(-41.76849889891,37.2283123829026,38.0964146476253));
#22066=CARTESIAN_POINT('Ctrl Pts',(-41.7689444904806,37.2290918141938,38.0973016070618));
#22067=CARTESIAN_POINT('Ctrl Pts',(-41.7693898781217,37.2298716152349,38.0981883440178));
#22068=CARTESIAN_POINT('Ctrl Pts',(-41.7698350617059,37.230651785803,38.0990748582399));
#22069=CARTESIAN_POINT('Ctrl Pts',(-41.7702802452902,37.2314319563711,38.0999613724619));
#22070=CARTESIAN_POINT('Ctrl Pts',(-41.7707252248176,37.2322124964663,38.10084766395));
#22071=CARTESIAN_POINT('Ctrl Pts',(-41.771170000161,37.2329934058654,38.1017337324509));
#22072=CARTESIAN_POINT('Ctrl Pts',(-41.7716147755045,37.2337743152645,38.1026198009518));
#22073=CARTESIAN_POINT('Ctrl Pts',(-41.772059346664,37.2345555939675,38.1035056464656));
#22074=CARTESIAN_POINT('Ctrl Pts',(-41.7725037135125,37.2353372417514,38.104391268739));
#22075=CARTESIAN_POINT('Ctrl Pts',(-41.7729480803611,37.2361188895352,38.1052768910125));
#22076=CARTESIAN_POINT('Ctrl Pts',(-41.7733922428986,37.2369009063998,38.1061622900455));
#22077=CARTESIAN_POINT('Ctrl Pts',(-41.7738362009983,37.2376832921216,38.1070474655853));
#22078=CARTESIAN_POINT('Ctrl Pts',(-41.774280159098,37.2384656778434,38.1079326411252));
#22079=CARTESIAN_POINT('Ctrl Pts',(-41.7747239127597,37.2392484324226,38.1088175931717));
#22080=CARTESIAN_POINT('Ctrl Pts',(-41.7751674618569,37.2400315556353,38.109702321472));
#22081=CARTESIAN_POINT('Ctrl Pts',(-41.775611010954,37.2408146788481,38.1105870497723));
#22082=CARTESIAN_POINT('Ctrl Pts',(-41.7760543554865,37.2415981706944,38.1114715543265));
#22083=CARTESIAN_POINT('Ctrl Pts',(-41.7764974953276,37.2423820309506,38.1123558348817));
#22084=CARTESIAN_POINT('Ctrl Pts',(-41.7769406351687,37.2431658912066,38.113240115437));
#22085=CARTESIAN_POINT('Ctrl Pts',(-41.7773835703185,37.2439501198725,38.1141241719933));
#22086=CARTESIAN_POINT('Ctrl Pts',(-41.7778263006504,37.244734716724,38.1150080042981));
#22087=CARTESIAN_POINT('Ctrl Pts',(-41.7782690309824,37.2455193135755,38.1158918366028));
#22088=CARTESIAN_POINT('Ctrl Pts',(-41.7787115564964,37.2463042786126,38.1167754446561));
#22089=CARTESIAN_POINT('Ctrl Pts',(-41.7791538770661,37.2470896116111,38.1176588282053));
#22090=CARTESIAN_POINT('Ctrl Pts',(-41.7795961976358,37.2478749446096,38.1185422117546));
#22091=CARTESIAN_POINT('Ctrl Pts',(-41.7800383132612,37.2486606455695,38.1194253707998));
#22092=CARTESIAN_POINT('Ctrl Pts',(-41.780480223816,37.2494467142662,38.1203083050887));
#22093=CARTESIAN_POINT('Ctrl Pts',(-41.7809221343707,37.2502327829629,38.1211912393775));
#22094=CARTESIAN_POINT('Ctrl Pts',(-41.7813638398548,37.2510192193965,38.1220739489099));
#22095=CARTESIAN_POINT('Ctrl Pts',(-41.7818053401422,37.2518060233422,38.1229564334338));
#22096=CARTESIAN_POINT('Ctrl Pts',(-41.7822468404294,37.2525928272879,38.1238389179577));
#22097=CARTESIAN_POINT('Ctrl Pts',(-41.7826881355199,37.2533799987457,38.124721177473));
#22098=CARTESIAN_POINT('Ctrl Pts',(-41.7831292252874,37.2541675374908,38.1256032117275));
#22099=CARTESIAN_POINT('Ctrl Pts',(-41.7835703150549,37.2549550762359,38.1264852459821));
#22100=CARTESIAN_POINT('Ctrl Pts',(-41.7840111994995,37.2557429822681,38.1273670549759));
#22101=CARTESIAN_POINT('Ctrl Pts',(-41.7844518784953,37.2565312553624,38.1282486384571));
#22102=CARTESIAN_POINT('Ctrl Pts',(-41.784892557491,37.2573195284568,38.1291302219383));
#22103=CARTESIAN_POINT('Ctrl Pts',(-41.7853330310378,37.2581081686132,38.1300115799068));
#22104=CARTESIAN_POINT('Ctrl Pts',(-41.7857732990099,37.2588971756064,38.1308927121107));
#22105=CARTESIAN_POINT('Ctrl Pts',(-41.786213566982,37.2596861825995,38.1317738443147));
#22106=CARTESIAN_POINT('Ctrl Pts',(-41.7866536293793,37.2604755564294,38.1326547507541));
#22107=CARTESIAN_POINT('Ctrl Pts',(-41.7870934860762,37.2612652968705,38.1335354311773));
#22108=CARTESIAN_POINT('Ctrl Pts',(-41.7647094275776,37.222307870463,38.089888730797));
#22109=CARTESIAN_POINT('Ctrl Pts',(-41.7651722267075,37.2231126056039,38.0908073680508));
#22110=CARTESIAN_POINT('Ctrl Pts',(-41.7656348077892,37.2239177373345,38.091725767728));
#22111=CARTESIAN_POINT('Ctrl Pts',(-41.7660971706813,37.2247232654083,38.0926439295475));
#22112=CARTESIAN_POINT('Ctrl Pts',(-41.7665591230165,37.2255280782106,38.093561276082));
#22113=CARTESIAN_POINT('Ctrl Pts',(-41.7670208575494,37.2263332866526,38.0944783851809));
#22114=CARTESIAN_POINT('Ctrl Pts',(-41.7674823741388,37.2271388904882,38.0953952565644));
#22115=CARTESIAN_POINT('Ctrl Pts',(-41.7679438907283,37.2279444943239,38.0963121279478));
#22116=CARTESIAN_POINT('Ctrl Pts',(-41.7684051893743,37.2287504935532,38.0972287616156));
#22117=CARTESIAN_POINT('Ctrl Pts',(-41.7688662699361,37.2295568879302,38.0981451572879));
#22118=CARTESIAN_POINT('Ctrl Pts',(-41.7693273504978,37.2303632823071,38.0990615529601));
#22119=CARTESIAN_POINT('Ctrl Pts',(-41.7697882129753,37.2311700718315,38.0999777106368));
#22120=CARTESIAN_POINT('Ctrl Pts',(-41.7702488572277,37.231977256257,38.1008936300381));
#22121=CARTESIAN_POINT('Ctrl Pts',(-41.7707095014801,37.2327844406825,38.1018095494393));
#22122=CARTESIAN_POINT('Ctrl Pts',(-41.7711699275075,37.2335920200091,38.1027252305651));
#22123=CARTESIAN_POINT('Ctrl Pts',(-41.7716301351692,37.2343999939901,38.1036406731358));
#22124=CARTESIAN_POINT('Ctrl Pts',(-41.7720903428309,37.235207967971,38.1045561157065));
#22125=CARTESIAN_POINT('Ctrl Pts',(-41.7725503321269,37.2360163366064,38.105471319722));
#22126=CARTESIAN_POINT('Ctrl Pts',(-41.7730101029167,37.2368250996492,38.1063862849029));
#22127=CARTESIAN_POINT('Ctrl Pts',(-41.7734698737066,37.237633862692,38.1073012500838));
#22128=CARTESIAN_POINT('Ctrl Pts',(-41.7739294259903,37.2384430201423,38.1082159764299));
#22129=CARTESIAN_POINT('Ctrl Pts',(-41.7743887596274,37.2392525717529,38.1091304636619));
#22130=CARTESIAN_POINT('Ctrl Pts',(-41.7748480932646,37.2400621233635,38.110044950894));
#22131=CARTESIAN_POINT('Ctrl Pts',(-41.7753072082553,37.2408720691344,38.1109591990119));
#22132=CARTESIAN_POINT('Ctrl Pts',(-41.7757661044592,37.2416824088182,38.1118732077365));
#22133=CARTESIAN_POINT('Ctrl Pts',(-41.7762250006631,37.242492748502,38.1127872164611));
#22134=CARTESIAN_POINT('Ctrl Pts',(-41.7766836780803,37.2433034820986,38.1137009857923));
#22135=CARTESIAN_POINT('Ctrl Pts',(-41.7771421365706,37.2441146093606,38.1146145154509));
#22136=CARTESIAN_POINT('Ctrl Pts',(-41.7776005950609,37.2449257366225,38.1155280451096));
#22137=CARTESIAN_POINT('Ctrl Pts',(-41.7780588346244,37.2457372575497,38.1164413350958));
#22138=CARTESIAN_POINT('Ctrl Pts',(-41.7785168551212,37.2465491718942,38.1173543851306));
#22139=CARTESIAN_POINT('Ctrl Pts',(-41.7789748756179,37.2473610862387,38.1182674351653));
#22140=CARTESIAN_POINT('Ctrl Pts',(-41.7794326770479,37.2481733940007,38.1191802452485));
#22141=CARTESIAN_POINT('Ctrl Pts',(-41.7798902592712,37.2489860949319,38.1200928151015));
#22142=CARTESIAN_POINT('Ctrl Pts',(-41.7803478414945,37.249798795863,38.1210053849544));
#22143=CARTESIAN_POINT('Ctrl Pts',(-41.7808052045112,37.2506118899634,38.1219177145771));
#22144=CARTESIAN_POINT('Ctrl Pts',(-41.7812623481816,37.2514253769846,38.1228298036907));
#22145=CARTESIAN_POINT('Ctrl Pts',(-41.7817194918521,37.2522388640059,38.1237418928044));
#22146=CARTESIAN_POINT('Ctrl Pts',(-41.7821764161762,37.2530527439481,38.124653741409));
#22147=CARTESIAN_POINT('Ctrl Pts',(-41.7826331210144,37.2538670165625,38.1255653492261));
#22148=CARTESIAN_POINT('Ctrl Pts',(-41.7830898258527,37.2546812891769,38.1264769570433));
#22149=CARTESIAN_POINT('Ctrl Pts',(-41.7835463112051,37.2554959544635,38.1273883240729));
#22150=CARTESIAN_POINT('Ctrl Pts',(-41.7840025769323,37.2563110121736,38.1282994500366));
#22151=CARTESIAN_POINT('Ctrl Pts',(-41.7844588426594,37.2571260698838,38.1292105760003));
#22152=CARTESIAN_POINT('Ctrl Pts',(-41.7849148887613,37.2579415200173,38.1301214608981));
#22153=CARTESIAN_POINT('Ctrl Pts',(-41.7853707150985,37.2587573623252,38.1310321044517));
#22154=CARTESIAN_POINT('Ctrl Pts',(-41.7858265414359,37.259573204633,38.1319427480054));
#22155=CARTESIAN_POINT('Ctrl Pts',(-41.7862821480086,37.2603894391152,38.1328531502148));
#22156=CARTESIAN_POINT('Ctrl Pts',(-41.7867375346776,37.2612060655225,38.133763310802));
#22157=CARTESIAN_POINT('Ctrl Pts',(-41.7635903731375,37.2209721633598,38.0886841910433));
#22158=CARTESIAN_POINT('Ctrl Pts',(-41.7640693209891,37.221803081553,38.0896329539864));
#22159=CARTESIAN_POINT('Ctrl Pts',(-41.7645480360178,37.2226344235192,38.090581463325));
#22160=CARTESIAN_POINT('Ctrl Pts',(-41.7650265180668,37.223466188986,38.0915297187483));
#22161=CARTESIAN_POINT('Ctrl Pts',(-41.7655045752459,37.2242972158836,38.0924771321649));
#22162=CARTESIAN_POINT('Ctrl Pts',(-41.7659823998588,37.2251286655302,38.0934242921168));
#22163=CARTESIAN_POINT('Ctrl Pts',(-41.7664599917494,37.2259605376537,38.0943711982946));
#22164=CARTESIAN_POINT('Ctrl Pts',(-41.7669375836398,37.2267924097772,38.0953181044724));
#22165=CARTESIAN_POINT('Ctrl Pts',(-41.7674149428079,37.2276247043777,38.0962647568759));
#22166=CARTESIAN_POINT('Ctrl Pts',(-41.7678920690975,37.228457421183,38.0972111551956));
#22167=CARTESIAN_POINT('Ctrl Pts',(-41.768369195387,37.2292901379882,38.0981575535153));
#22168=CARTESIAN_POINT('Ctrl Pts',(-41.768846088798,37.2301232769982,38.0991036977512));
#22169=CARTESIAN_POINT('Ctrl Pts',(-41.7693227491746,37.2309568379406,38.1000495875938));
#22170=CARTESIAN_POINT('Ctrl Pts',(-41.7697994095511,37.231790398883,38.1009954774365));
#22171=CARTESIAN_POINT('Ctrl Pts',(-41.7702758368932,37.2326243817577,38.1019411128859));
#22172=CARTESIAN_POINT('Ctrl Pts',(-41.7707520310449,37.2334587862921,38.1028864936329));
#22173=CARTESIAN_POINT('Ctrl Pts',(-41.7712282251966,37.2342931908265,38.1038318743798));
#22174=CARTESIAN_POINT('Ctrl Pts',(-41.7717041861582,37.2351280170204,38.1047770004243));
#22175=CARTESIAN_POINT('Ctrl Pts',(-41.7721799137737,37.235963264601,38.1057218714573));
#22176=CARTESIAN_POINT('Ctrl Pts',(-41.7726556413892,37.2367985121816,38.1066667424903));
#22177=CARTESIAN_POINT('Ctrl Pts',(-41.7731311356589,37.2376341811488,38.1076113585118));
#22178=CARTESIAN_POINT('Ctrl Pts',(-41.7736063964271,37.2384702712294,38.1085557192128));
#22179=CARTESIAN_POINT('Ctrl Pts',(-41.7740816571953,37.23930636131,38.1095000799138));
#22180=CARTESIAN_POINT('Ctrl Pts',(-41.774556684462,37.2401428725039,38.1104441852944));
#22181=CARTESIAN_POINT('Ctrl Pts',(-41.7750314780721,37.2409798045376,38.1113880350459));
#22182=CARTESIAN_POINT('Ctrl Pts',(-41.7755062716821,37.2418167365713,38.1123318847973));
#22183=CARTESIAN_POINT('Ctrl Pts',(-41.7759808316353,37.2426540894449,38.1132754789196));
#22184=CARTESIAN_POINT('Ctrl Pts',(-41.7764551577767,37.2434918628844,38.1142188171042));
#22185=CARTESIAN_POINT('Ctrl Pts',(-41.776929483918,37.2443296363239,38.1151621552887));
#22186=CARTESIAN_POINT('Ctrl Pts',(-41.7774035762474,37.2451678303293,38.1161052375356));
#22187=CARTESIAN_POINT('Ctrl Pts',(-41.7778774346097,37.2460064446267,38.1170480635362));
#22188=CARTESIAN_POINT('Ctrl Pts',(-41.7783512929721,37.246845058924,38.117990889537));
#22189=CARTESIAN_POINT('Ctrl Pts',(-41.7788249173675,37.2476840935132,38.1189334592915));
#22190=CARTESIAN_POINT('Ctrl Pts',(-41.7792983076411,37.24852354812,38.1198757724917));
#22191=CARTESIAN_POINT('Ctrl Pts',(-41.7797716979146,37.2493630027266,38.120818085692));
#22192=CARTESIAN_POINT('Ctrl Pts',(-41.7802448540663,37.2502028773509,38.1217601423378));
#22193=CARTESIAN_POINT('Ctrl Pts',(-41.7807177759414,37.251043171718,38.1227019421212));
#22194=CARTESIAN_POINT('Ctrl Pts',(-41.7811906978165,37.251883466085,38.1236437419047));
#22195=CARTESIAN_POINT('Ctrl Pts',(-41.781663385415,37.2527241801949,38.1245852848257));
#22196=CARTESIAN_POINT('Ctrl Pts',(-41.7821358385823,37.2535653137728,38.1255265705763));
#22197=CARTESIAN_POINT('Ctrl Pts',(-41.7826082917497,37.2544064473506,38.126467856327));
#22198=CARTESIAN_POINT('Ctrl Pts',(-41.7830805104859,37.2552480003964,38.1274088849074));
#22199=CARTESIAN_POINT('Ctrl Pts',(-41.7835524946364,37.2560899726349,38.1283496560097));
#22200=CARTESIAN_POINT('Ctrl Pts',(-41.784024478787,37.2569319448734,38.1292904271121));
#22201=CARTESIAN_POINT('Ctrl Pts',(-41.784496228352,37.2577743363046,38.1302309407363));
#22202=CARTESIAN_POINT('Ctrl Pts',(-41.7849677431772,37.2586171466531,38.131171196575));
#22203=CARTESIAN_POINT('Ctrl Pts',(-41.7854392580023,37.2594599570016,38.1321114524136));
#22204=CARTESIAN_POINT('Ctrl Pts',(-41.7859105380876,37.2603031862673,38.1330514504667));
#22205=CARTESIAN_POINT('Ctrl Pts',(-41.7863815832789,37.2611468341745,38.1339911904267));
#22206=CARTESIAN_POINT('Ctrl Pts',(-41.7624713186973,37.2196364562566,38.0874796512896));
#22207=CARTESIAN_POINT('Ctrl Pts',(-41.7629664152707,37.2204935575021,38.088458539922));
#22208=CARTESIAN_POINT('Ctrl Pts',(-41.7634612642464,37.2213511097039,38.089437158922));
#22209=CARTESIAN_POINT('Ctrl Pts',(-41.7639558654523,37.2222091125637,38.0904155079491));
#22210=CARTESIAN_POINT('Ctrl Pts',(-41.7644500274753,37.2230663535568,38.0913929882477));
#22211=CARTESIAN_POINT('Ctrl Pts',(-41.7649439421683,37.2239240444079,38.0923701990528));
#22212=CARTESIAN_POINT('Ctrl Pts',(-41.7654376093599,37.2247821848192,38.0933471400249));
#22213=CARTESIAN_POINT('Ctrl Pts',(-41.7659312765514,37.2256403252306,38.094324080997));
#22214=CARTESIAN_POINT('Ctrl Pts',(-41.7664246962416,37.2264989152021,38.0953007521362));
#22215=CARTESIAN_POINT('Ctrl Pts',(-41.7669178682589,37.2273579544356,38.0962771531033));
#22216=CARTESIAN_POINT('Ctrl Pts',(-41.7674110402762,37.2282169936692,38.0972535540705));
#22217=CARTESIAN_POINT('Ctrl Pts',(-41.7679039646208,37.2290764821649,38.0982296848655));
#22218=CARTESIAN_POINT('Ctrl Pts',(-41.7683966411214,37.2299364196242,38.0992055451495));
#22219=CARTESIAN_POINT('Ctrl Pts',(-41.7688893176221,37.2307963570835,38.1001814054336));
#22220=CARTESIAN_POINT('Ctrl Pts',(-41.7693817462788,37.2316567435063,38.1011569952067));
#22221=CARTESIAN_POINT('Ctrl Pts',(-41.7698739269206,37.2325175785941,38.1021323141299));
#22222=CARTESIAN_POINT('Ctrl Pts',(-41.7703661075624,37.2333784136818,38.1031076330531));
#22223=CARTESIAN_POINT('Ctrl Pts',(-41.7708580401894,37.2342396974344,38.1040826811266));
#22224=CARTESIAN_POINT('Ctrl Pts',(-41.7713497246306,37.2351014295528,38.1050574580117));
#22225=CARTESIAN_POINT('Ctrl Pts',(-41.7718414090719,37.2359631616712,38.1060322348969));
#22226=CARTESIAN_POINT('Ctrl Pts',(-41.7723328453274,37.2368253421553,38.1070067405936));
#22227=CARTESIAN_POINT('Ctrl Pts',(-41.7728240332267,37.2376879707059,38.1079809747636));
#22228=CARTESIAN_POINT('Ctrl Pts',(-41.7733152211259,37.2385505992564,38.1089552089337));
#22229=CARTESIAN_POINT('Ctrl Pts',(-41.7738061606688,37.2394136758734,38.1099291715769));
#22230=CARTESIAN_POINT('Ctrl Pts',(-41.774296851685,37.240277200257,38.1109028623553));
#22231=CARTESIAN_POINT('Ctrl Pts',(-41.7747875427011,37.2411407246407,38.1118765531336));
#22232=CARTESIAN_POINT('Ctrl Pts',(-41.7752779851904,37.242004696791,38.112849972047));
#22233=CARTESIAN_POINT('Ctrl Pts',(-41.7757681789827,37.2428691164081,38.1138231187574));
#22234=CARTESIAN_POINT('Ctrl Pts',(-41.776258372775,37.2437335360252,38.1147962654678));
#22235=CARTESIAN_POINT('Ctrl Pts',(-41.7767483178702,37.244598403109,38.1157691399753));
#22236=CARTESIAN_POINT('Ctrl Pts',(-41.7772380140983,37.2454637173591,38.1167417419419));
#22237=CARTESIAN_POINT('Ctrl Pts',(-41.7777277103263,37.2463290316093,38.1177143439086));
#22238=CARTESIAN_POINT('Ctrl Pts',(-41.7782171576872,37.2471947930257,38.1186866733346));
#22239=CARTESIAN_POINT('Ctrl Pts',(-41.778706356011,37.2480610013081,38.119658729882));
#22240=CARTESIAN_POINT('Ctrl Pts',(-41.7791955543347,37.2489272095904,38.1206307864295));
#22241=CARTESIAN_POINT('Ctrl Pts',(-41.7796845036214,37.2497938647384,38.1216025700986));
#22242=CARTESIAN_POINT('Ctrl Pts',(-41.7801732037012,37.2506609664512,38.1225740805518));
#22243=CARTESIAN_POINT('Ctrl Pts',(-41.7806619037809,37.2515280681641,38.123545591005));
#22244=CARTESIAN_POINT('Ctrl Pts',(-41.7811503546538,37.2523956164418,38.1245168282424));
#22245=CARTESIAN_POINT('Ctrl Pts',(-41.7816385561502,37.2532636109831,38.1254877919266));
#22246=CARTESIAN_POINT('Ctrl Pts',(-41.7821267576466,37.2541316055244,38.1264587556108));
#22247=CARTESIAN_POINT('Ctrl Pts',(-41.7826147097666,37.2550000463293,38.1274294457419));
#22248=CARTESIAN_POINT('Ctrl Pts',(-41.7831024123406,37.2558689330961,38.1283998619829));
#22249=CARTESIAN_POINT('Ctrl Pts',(-41.7835901149147,37.256737819863,38.1293702782238));
#22250=CARTESIAN_POINT('Ctrl Pts',(-41.7840775679428,37.2576071525919,38.1303404205745));
#22251=CARTESIAN_POINT('Ctrl Pts',(-41.7845647712558,37.258476930981,38.1313102886982));
#22252=CARTESIAN_POINT('Ctrl Pts',(-41.7850519745688,37.25934670937,38.1322801568219));
#22253=CARTESIAN_POINT('Ctrl Pts',(-41.7855389281667,37.2602169334193,38.1332497507186));
#22254=CARTESIAN_POINT('Ctrl Pts',(-41.7860256318803,37.2610876028265,38.1342190700514));
#22255=CARTESIAN_POINT('Ctrl Pts',(-41.7613770641789,37.2183331411396,38.0863036281828));
#22256=CARTESIAN_POINT('Ctrl Pts',(-41.7618876562635,37.2192157760948,38.0873122441619));
#22257=CARTESIAN_POINT('Ctrl Pts',(-41.7623979856072,37.2200988899049,38.0883205740934));
#22258=CARTESIAN_POINT('Ctrl Pts',(-41.7629080520215,37.2209824822438,38.0893286176052));
#22259=CARTESIAN_POINT('Ctrl Pts',(-41.7634176655205,37.2218652899938,38.0903357660211));
#22260=CARTESIAN_POINT('Ctrl Pts',(-41.7639270165568,37.222748575423,38.0913426285256));
#22261=CARTESIAN_POINT('Ctrl Pts',(-41.7644361049428,37.223632338206,38.0923492047476));
#22262=CARTESIAN_POINT('Ctrl Pts',(-41.7649451933288,37.224516100989,38.0933557809696));
#22263=CARTESIAN_POINT('Ctrl Pts',(-41.7654540190643,37.2254003411258,38.0943620709091));
#22264=CARTESIAN_POINT('Ctrl Pts',(-41.765962581962,37.2262850582903,38.0953680741951));
#22265=CARTESIAN_POINT('Ctrl Pts',(-41.7664711448597,37.2271697754548,38.0963740774812));
#22266=CARTESIAN_POINT('Ctrl Pts',(-41.7669794449194,37.2280549696471,38.0973797941137));
#22267=CARTESIAN_POINT('Ctrl Pts',(-41.7674874819539,37.2289406405409,38.0983852237221));
#22268=CARTESIAN_POINT('Ctrl Pts',(-41.7679955189883,37.2298263114347,38.0993906533304));
#22269=CARTESIAN_POINT('Ctrl Pts',(-41.7685032929975,37.2307124590299,38.1003957959146));
#22270=CARTESIAN_POINT('Ctrl Pts',(-41.7690108037943,37.231599083,38.1014006511041));
#22271=CARTESIAN_POINT('Ctrl Pts',(-41.7695183145911,37.2324857069701,38.1024055062937));
#22272=CARTESIAN_POINT('Ctrl Pts',(-41.7700255621754,37.233372807315,38.1034100740885));
#22273=CARTESIAN_POINT('Ctrl Pts',(-41.7705325463604,37.2342603837078,38.1044143541183));
#22274=CARTESIAN_POINT('Ctrl Pts',(-41.7710395305453,37.2351479601006,38.1054186341482));
#22275=CARTESIAN_POINT('Ctrl Pts',(-41.7715462513308,37.2360360125412,38.106422626413));
#22276=CARTESIAN_POINT('Ctrl Pts',(-41.7720527085303,37.2369245407023,38.1074263305428));
#22277=CARTESIAN_POINT('Ctrl Pts',(-41.7725591657296,37.2378130688634,38.1084300346726));
#22278=CARTESIAN_POINT('Ctrl Pts',(-41.7730653593429,37.238702072745,38.1094334506673));
#22279=CARTESIAN_POINT('Ctrl Pts',(-41.7735712891834,37.2395915520194,38.110436578157));
#22280=CARTESIAN_POINT('Ctrl Pts',(-41.7740772190239,37.2404810312937,38.1114397056469));
#22281=CARTESIAN_POINT('Ctrl Pts',(-41.7745828850917,37.2413709859609,38.1124425446317));
#22282=CARTESIAN_POINT('Ctrl Pts',(-41.7750882872003,37.2422614156928,38.1134450947419));
#22283=CARTESIAN_POINT('Ctrl Pts',(-41.775593689309,37.2431518454246,38.1144476448522));
#22284=CARTESIAN_POINT('Ctrl Pts',(-41.7760988274585,37.2440427502213,38.1154499060878));
#22285=CARTESIAN_POINT('Ctrl Pts',(-41.7766037014628,37.2449341297543,38.1164518780793));
#22286=CARTESIAN_POINT('Ctrl Pts',(-41.777108575467,37.2458255092872,38.1174538500709));
#22287=CARTESIAN_POINT('Ctrl Pts',(-41.777613185326,37.2467173635565,38.1184555328185));
#22288=CARTESIAN_POINT('Ctrl Pts',(-41.7781175308536,37.2476096922334,38.1194569259527));
#22289=CARTESIAN_POINT('Ctrl Pts',(-41.7786218763813,37.2485020209103,38.1204583190869));
#22290=CARTESIAN_POINT('Ctrl Pts',(-41.7791259575776,37.2493948239948,38.1214594226079));
#22291=CARTESIAN_POINT('Ctrl Pts',(-41.7796297742569,37.2502881011577,38.1224602361465));
#22292=CARTESIAN_POINT('Ctrl Pts',(-41.7801335909362,37.2511813783207,38.1234610496852));
#22293=CARTESIAN_POINT('Ctrl Pts',(-41.7806371430984,37.2520751295621,38.1244615732415));
#22294=CARTESIAN_POINT('Ctrl Pts',(-41.7811404305579,37.2529693545526,38.1254618064468));
#22295=CARTESIAN_POINT('Ctrl Pts',(-41.7816437180174,37.2538635795431,38.126462039652));
#22296=CARTESIAN_POINT('Ctrl Pts',(-41.7821467407742,37.2547582782826,38.1274619825061));
#22297=CARTESIAN_POINT('Ctrl Pts',(-41.7826494986429,37.2556534504414,38.1284616346405));
#22298=CARTESIAN_POINT('Ctrl Pts',(-41.7831522565116,37.2565486226002,38.1294612867749));
#22299=CARTESIAN_POINT('Ctrl Pts',(-41.7836547494923,37.2574442681782,38.1304606481896));
#22300=CARTESIAN_POINT('Ctrl Pts',(-41.7841569773996,37.2583403868454,38.1314597185161));
#22301=CARTESIAN_POINT('Ctrl Pts',(-41.7846592053069,37.2592365055125,38.1324587888427));
#22302=CARTESIAN_POINT('Ctrl Pts',(-41.7851611681409,37.2601330972687,38.1334575680812));
#22303=CARTESIAN_POINT('Ctrl Pts',(-41.7856628657165,37.2610301617836,38.1344560558635));
#22304=CARTESIAN_POINT('Ctrl Pts',(-41.7602656007636,37.217011975673,38.0851109242317));
#22305=CARTESIAN_POINT('Ctrl Pts',(-41.760792130705,37.2179204777448,38.0861495472797));
#22306=CARTESIAN_POINT('Ctrl Pts',(-41.7613183818872,37.2188294882312,38.0871878669253));
#22307=CARTESIAN_POINT('Ctrl Pts',(-41.7618443541036,37.2197390067751,38.088225882761));
#22308=CARTESIAN_POINT('Ctrl Pts',(-41.7623698592811,37.2206477177089,38.0892629768868));
#22309=CARTESIAN_POINT('Ctrl Pts',(-41.7628950859879,37.2215569357985,38.0902997677418));
#22310=CARTESIAN_POINT('Ctrl Pts',(-41.7634200340183,37.2224666606875,38.0913362549198));
#22311=CARTESIAN_POINT('Ctrl Pts',(-41.7639449820487,37.2233763855765,38.0923727420979));
#22312=CARTESIAN_POINT('Ctrl Pts',(-41.7644696514026,37.224286617265,38.0934089255988));
#22313=CARTESIAN_POINT('Ctrl Pts',(-41.7649940418743,37.2251973553961,38.0944448050165));
#22314=CARTESIAN_POINT('Ctrl Pts',(-41.7655184323462,37.2261080935271,38.0954806844343));
#22315=CARTESIAN_POINT('Ctrl Pts',(-41.7660425439358,37.2270193381009,38.0965162597688));
#22316=CARTESIAN_POINT('Ctrl Pts',(-41.7665663764379,37.2279310887602,38.0975515306143));
#22317=CARTESIAN_POINT('Ctrl Pts',(-41.76709020894,37.2288428394195,38.0985868014598));
#22318=CARTESIAN_POINT('Ctrl Pts',(-41.7676137623545,37.2297550961644,38.0996217678161));
#22319=CARTESIAN_POINT('Ctrl Pts',(-41.7681370364763,37.2306678586371,38.1006564292777));
#22320=CARTESIAN_POINT('Ctrl Pts',(-41.7686603105981,37.2315806211098,38.1016910907394));
#22321=CARTESIAN_POINT('Ctrl Pts',(-41.7691833054271,37.2324938893106,38.1027254473063));
#22322=CARTESIAN_POINT('Ctrl Pts',(-41.7697060207585,37.2334076628813,38.1037594985731));
#22323=CARTESIAN_POINT('Ctrl Pts',(-41.7702287360898,37.234321436452,38.1047935498398));
#22324=CARTESIAN_POINT('Ctrl Pts',(-41.7707511719234,37.2352357153927,38.1058272958065));
#22325=CARTESIAN_POINT('Ctrl Pts',(-41.7712733280544,37.2361504993452,38.1068607360678));
#22326=CARTESIAN_POINT('Ctrl Pts',(-41.7717954841855,37.2370652832975,38.1078941763291));
#22327=CARTESIAN_POINT('Ctrl Pts',(-41.772317360614,37.2379805722616,38.1089273108851));
#22328=CARTESIAN_POINT('Ctrl Pts',(-41.7728389571356,37.2388963658785,38.1099601393308));
#22329=CARTESIAN_POINT('Ctrl Pts',(-41.7733605536571,37.2398121594955,38.1109929677765));
#22330=CARTESIAN_POINT('Ctrl Pts',(-41.7738818702715,37.2407284577654,38.112025490112));
#22331=CARTESIAN_POINT('Ctrl Pts',(-41.7744029067746,37.241645260329,38.1130577059326));
#22332=CARTESIAN_POINT('Ctrl Pts',(-41.7749239432777,37.2425620628927,38.1140899217531));
#22333=CARTESIAN_POINT('Ctrl Pts',(-41.7754446996694,37.2434793697501,38.1151218310587));
#22334=CARTESIAN_POINT('Ctrl Pts',(-41.7759651757456,37.2443971805418,38.1161534334449));
#22335=CARTESIAN_POINT('Ctrl Pts',(-41.7764856518219,37.2453149913334,38.1171850358311));
#22336=CARTESIAN_POINT('Ctrl Pts',(-41.7770058475826,37.2462333060593,38.1182163312979));
#22337=CARTESIAN_POINT('Ctrl Pts',(-41.7775257628239,37.2471521243595,38.1192473194412));
#22338=CARTESIAN_POINT('Ctrl Pts',(-41.7780456780652,37.2480709426598,38.1202783075843));
#22339=CARTESIAN_POINT('Ctrl Pts',(-41.7785653127873,37.2489902645343,38.1213089884039));
#22340=CARTESIAN_POINT('Ctrl Pts',(-41.7790846667862,37.2499100896229,38.1223393614959));
#22341=CARTESIAN_POINT('Ctrl Pts',(-41.7796040207851,37.2508299147114,38.123369734588));
#22342=CARTESIAN_POINT('Ctrl Pts',(-41.780123094061,37.2517502430139,38.1243997999524));
#22343=CARTESIAN_POINT('Ctrl Pts',(-41.7806418864104,37.2526710741697,38.1254295571855));
#22344=CARTESIAN_POINT('Ctrl Pts',(-41.7811606787598,37.2535919053255,38.1264593144186));
#22345=CARTESIAN_POINT('Ctrl Pts',(-41.7816791901827,37.2545132393345,38.1274887635205));
#22346=CARTESIAN_POINT('Ctrl Pts',(-41.7821974204759,37.2554350758357,38.1285179040875));
#22347=CARTESIAN_POINT('Ctrl Pts',(-41.782715650769,37.2563569123369,38.1295470446545));
#22348=CARTESIAN_POINT('Ctrl Pts',(-41.7832335999325,37.2572792513303,38.1305758766868));
#22349=CARTESIAN_POINT('Ctrl Pts',(-41.7837512677633,37.2582020924543,38.131604399781));
#22350=CARTESIAN_POINT('Ctrl Pts',(-41.784268935594,37.2591249335783,38.1326329228752));
#22351=CARTESIAN_POINT('Ctrl Pts',(-41.784786322092,37.260048276833,38.1336611370313));
#22352=CARTESIAN_POINT('Ctrl Pts',(-41.7853034270545,37.2609721218564,38.1346890418465));
#22353=CARTESIAN_POINT('Ctrl Pts',(-41.7558197471023,37.2117273138067,38.0803401084276));
#22354=CARTESIAN_POINT('Ctrl Pts',(-41.7564100284709,37.2127392843447,38.0814987597511));
#22355=CARTESIAN_POINT('Ctrl Pts',(-41.7569999670072,37.213751881536,38.082657038253));
#22356=CARTESIAN_POINT('Ctrl Pts',(-41.7575895624321,37.2147651049003,38.0838149433843));
#22357=CARTESIAN_POINT('Ctrl Pts',(-41.7581786343235,37.2157774285695,38.0849718203494));
#22358=CARTESIAN_POINT('Ctrl Pts',(-41.7587673637124,37.2167903773003,38.0861283246066));
#22359=CARTESIAN_POINT('Ctrl Pts',(-41.7593557503204,37.2178039506134,38.0872844556087));
#22360=CARTESIAN_POINT('Ctrl Pts',(-41.7599441369285,37.2188175239264,38.0884405866107));
#22361=CARTESIAN_POINT('Ctrl Pts',(-41.7605321807556,37.2198317218217,38.0895963443575));
#22362=CARTESIAN_POINT('Ctrl Pts',(-41.7611198815238,37.2208465438191,38.0907517283021));
#22363=CARTESIAN_POINT('Ctrl Pts',(-41.761707582292,37.2218613658167,38.0919071122468));
#22364=CARTESIAN_POINT('Ctrl Pts',(-41.7622949400013,37.2228768119163,38.0930621223893));
#22365=CARTESIAN_POINT('Ctrl Pts',(-41.7628819543739,37.2238928816376,38.0942167581831));
#22366=CARTESIAN_POINT('Ctrl Pts',(-41.7634689687465,37.224908951359,38.0953713939769));
#22367=CARTESIAN_POINT('Ctrl Pts',(-41.7640556397825,37.225925644702,38.096525655422));
#22368=CARTESIAN_POINT('Ctrl Pts',(-41.7646419672044,37.2269429611854,38.0976795419723));
#22369=CARTESIAN_POINT('Ctrl Pts',(-41.7652282946264,37.2279602776687,38.0988334285225));
#22370=CARTESIAN_POINT('Ctrl Pts',(-41.7658142784342,37.2289782172926,38.0999869401777));
#22371=CARTESIAN_POINT('Ctrl Pts',(-41.766399918351,37.2299967795751,38.1011400763922));
#22372=CARTESIAN_POINT('Ctrl Pts',(-41.7669855582677,37.2310153418577,38.1022932126067));
#22373=CARTESIAN_POINT('Ctrl Pts',(-41.7675708542934,37.2320345267988,38.1034459733804));
#22374=CARTESIAN_POINT('Ctrl Pts',(-41.7681558061512,37.2330543339164,38.1045983581678));
#22375=CARTESIAN_POINT('Ctrl Pts',(-41.7687407580089,37.234074141034,38.1057507429551));
#22376=CARTESIAN_POINT('Ctrl Pts',(-41.7693253656987,37.2350945703279,38.1069027517562));
#22377=CARTESIAN_POINT('Ctrl Pts',(-41.7699096289443,37.2361156213152,38.1080543840258));
#22378=CARTESIAN_POINT('Ctrl Pts',(-41.7704938921898,37.2371366723026,38.1092060162953));
#22379=CARTESIAN_POINT('Ctrl Pts',(-41.771077810991,37.2381583449833,38.1103572720334));
#22380=CARTESIAN_POINT('Ctrl Pts',(-41.7716613850718,37.2391806388741,38.1115081506952));
#22381=CARTESIAN_POINT('Ctrl Pts',(-41.7722449591525,37.2402029327648,38.112659029357));
#22382=CARTESIAN_POINT('Ctrl Pts',(-41.7728281885128,37.2412258478655,38.1138095309424));
#22383=CARTESIAN_POINT('Ctrl Pts',(-41.773411072877,37.2422493836919,38.1149596549072));
#22384=CARTESIAN_POINT('Ctrl Pts',(-41.773993957241,37.2432729195185,38.1161097788719));
#22385=CARTESIAN_POINT('Ctrl Pts',(-41.7745764966089,37.2442970760708,38.1172595252158));
#22386=CARTESIAN_POINT('Ctrl Pts',(-41.775158690705,37.2453218528644,38.1184088933949));
#22387=CARTESIAN_POINT('Ctrl Pts',(-41.7757408848011,37.246346629658,38.1195582615739));
#22388=CARTESIAN_POINT('Ctrl Pts',(-41.7763227336255,37.2473720266928,38.120707251588));
#22389=CARTESIAN_POINT('Ctrl Pts',(-41.7769042369031,37.2483980434835,38.1218558628935));
#22390=CARTESIAN_POINT('Ctrl Pts',(-41.7774857401807,37.2494240602743,38.123004474199));
#22391=CARTESIAN_POINT('Ctrl Pts',(-41.7780668979113,37.2504506968211,38.1241527067959));
#22392=CARTESIAN_POINT('Ctrl Pts',(-41.7786477098203,37.251477952638,38.1253005601407));
#22393=CARTESIAN_POINT('Ctrl Pts',(-41.7792285217293,37.2525052084549,38.1264484134854));
#22394=CARTESIAN_POINT('Ctrl Pts',(-41.7798089878166,37.253533083542,38.1275958875781));
#22395=CARTESIAN_POINT('Ctrl Pts',(-41.7803891078076,37.254561577413,38.1287429818757));
#22396=CARTESIAN_POINT('Ctrl Pts',(-41.7809692277987,37.2555900712838,38.1298900761733));
#22397=CARTESIAN_POINT('Ctrl Pts',(-41.7815490016936,37.2566191839385,38.1310367906757));
#22398=CARTESIAN_POINT('Ctrl Pts',(-41.782128429218,37.2576489148901,38.1321831248404));
#22399=CARTESIAN_POINT('Ctrl Pts',(-41.7827078567425,37.2586786458416,38.133329459005));
#22400=CARTESIAN_POINT('Ctrl Pts',(-41.7832869378965,37.2597089950899,38.1344754128318));
#22401=CARTESIAN_POINT('Ctrl Pts',(-41.7838656724063,37.2607399621476,38.1356209857784));
#22402=CARTESIAN_POINT('Ctrl Pts',(-41.7513111929665,37.2064115906167,38.0755313098334));
#22403=CARTESIAN_POINT('Ctrl Pts',(-41.751966757934,37.2075273833708,38.0768110311642));
#22404=CARTESIAN_POINT('Ctrl Pts',(-41.7526219045242,37.208643942912,38.0780902979841));
#22405=CARTESIAN_POINT('Ctrl Pts',(-41.7532766323584,37.2097612685937,38.0793691095526));
#22406=CARTESIAN_POINT('Ctrl Pts',(-41.7539307788246,37.210877602142,38.0806467855958));
#22407=CARTESIAN_POINT('Ctrl Pts',(-41.754584507278,37.2119947004709,38.0819240071957));
#22408=CARTESIAN_POINT('Ctrl Pts',(-41.7552378173414,37.2131125629345,38.0832007736143));
#22409=CARTESIAN_POINT('Ctrl Pts',(-41.7558911274048,37.2142304253979,38.0844775400328));
#22410=CARTESIAN_POINT('Ctrl Pts',(-41.7565440190782,37.2153490519962,38.08575385127));
#22411=CARTESIAN_POINT('Ctrl Pts',(-41.7571964919848,37.2164684420825,38.0870297065882));
#22412=CARTESIAN_POINT('Ctrl Pts',(-41.7578489648914,37.2175878321687,38.0883055619064));
#22413=CARTESIAN_POINT('Ctrl Pts',(-41.7585010190312,37.218707985743,38.0895809613056));
#22414=CARTESIAN_POINT('Ctrl Pts',(-41.7591526540278,37.2198289021578,38.0908559040488));
#22415=CARTESIAN_POINT('Ctrl Pts',(-41.7598042890245,37.2209498185725,38.0921308467919));
#22416=CARTESIAN_POINT('Ctrl Pts',(-41.760455504878,37.2220714978278,38.0934053328791));
#22417=CARTESIAN_POINT('Ctrl Pts',(-41.7611063012126,37.2231939392752,38.0946793615737));
#22418=CARTESIAN_POINT('Ctrl Pts',(-41.7617570975472,37.2243163807225,38.0959533902682));
#22419=CARTESIAN_POINT('Ctrl Pts',(-41.7624074743628,37.225439584362,38.0972269615702));
#22420=CARTESIAN_POINT('Ctrl Pts',(-41.763057431284,37.2265635495444,38.0985000747435));
#22421=CARTESIAN_POINT('Ctrl Pts',(-41.7637073882053,37.2276875147267,38.0997731879169));
#22422=CARTESIAN_POINT('Ctrl Pts',(-41.7643569252322,37.2288122414519,38.1010458429616));
#22423=CARTESIAN_POINT('Ctrl Pts',(-41.7650060419899,37.2299377290699,38.1023180391421));
#22424=CARTESIAN_POINT('Ctrl Pts',(-41.7656551587476,37.2310632166879,38.1035902353226));
#22425=CARTESIAN_POINT('Ctrl Pts',(-41.766303855236,37.2321894651987,38.104861972639));
#22426=CARTESIAN_POINT('Ctrl Pts',(-41.7669521310807,37.2333164739512,38.1061332503562));
#22427=CARTESIAN_POINT('Ctrl Pts',(-41.7676004069255,37.2344434827038,38.1074045280734));
#22428=CARTESIAN_POINT('Ctrl Pts',(-41.7682482621266,37.2355712516982,38.1086753461915));
#22429=CARTESIAN_POINT('Ctrl Pts',(-41.7688956963101,37.2366997802825,38.1099457039759));
#22430=CARTESIAN_POINT('Ctrl Pts',(-41.7695431304936,37.2378283088669,38.1112160617603));
#22431=CARTESIAN_POINT('Ctrl Pts',(-41.7701901436595,37.2389575970412,38.112485959211));
#22432=CARTESIAN_POINT('Ctrl Pts',(-41.7708367354343,37.2400876441529,38.1137553955942));
#22433=CARTESIAN_POINT('Ctrl Pts',(-41.7714833272091,37.2412176912646,38.1150248319773));
#22434=CARTESIAN_POINT('Ctrl Pts',(-41.7721294975928,37.2423484973136,38.1162938072928));
#22435=CARTESIAN_POINT('Ctrl Pts',(-41.7727752462124,37.2434800616463,38.1175623208073));
#22436=CARTESIAN_POINT('Ctrl Pts',(-41.773420994832,37.2446116259791,38.1188308343217));
#22437=CARTESIAN_POINT('Ctrl Pts',(-41.7740663216875,37.2457439485957,38.1200988860351));
#22438=CARTESIAN_POINT('Ctrl Pts',(-41.7747112264064,37.2468770288417,38.1213664752145));
#22439=CARTESIAN_POINT('Ctrl Pts',(-41.7753561311253,37.2480101090876,38.1226340643939));
#22440=CARTESIAN_POINT('Ctrl Pts',(-41.7760006137076,37.2491439469631,38.1239011910393));
#22441=CARTESIAN_POINT('Ctrl Pts',(-41.7766446737812,37.2502785418127,38.1251678544182));
#22442=CARTESIAN_POINT('Ctrl Pts',(-41.7772887338548,37.2514131366622,38.1264345177972));
#22443=CARTESIAN_POINT('Ctrl Pts',(-41.7779323714198,37.252548488486,38.1277007179098));
#22444=CARTESIAN_POINT('Ctrl Pts',(-41.7785755861045,37.2536845966279,38.1289664540241));
#22445=CARTESIAN_POINT('Ctrl Pts',(-41.7792188007892,37.2548207047697,38.1302321901384));
#22446=CARTESIAN_POINT('Ctrl Pts',(-41.7798615925936,37.2559575692297,38.1314974622543));
#22447=CARTESIAN_POINT('Ctrl Pts',(-41.7805039611468,37.2570951893507,38.1327622696407));
#22448=CARTESIAN_POINT('Ctrl Pts',(-41.7811463296999,37.2582328094719,38.134027077027));
#22449=CARTESIAN_POINT('Ctrl Pts',(-41.7817882750017,37.2593711852541,38.1352914196837));
#22450=CARTESIAN_POINT('Ctrl Pts',(-41.7824297966815,37.2605103160397,38.1365552968799));
#22451=CARTESIAN_POINT('Ctrl Pts',(-41.7467400817451,37.2010672456454,38.0706862117665));
#22452=CARTESIAN_POINT('Ctrl Pts',(-41.7474624663532,37.2022871437449,38.0720880159783));
#22453=CARTESIAN_POINT('Ctrl Pts',(-41.74818434518,37.2035079719612,38.0734892714123));
#22454=CARTESIAN_POINT('Ctrl Pts',(-41.7489057177088,37.204729729421,38.0748899770657));
#22455=CARTESIAN_POINT('Ctrl Pts',(-41.7496264496923,37.2059504020168,38.0762894389575));
#22456=CARTESIAN_POINT('Ctrl Pts',(-41.7503466762767,37.2071720022066,38.0776883520447));
#22457=CARTESIAN_POINT('Ctrl Pts',(-41.7510663969476,37.2083945291177,38.0790867153282));
#22458=CARTESIAN_POINT('Ctrl Pts',(-41.7517861176184,37.2096170560288,38.0804850786117));
#22459=CARTESIAN_POINT('Ctrl Pts',(-41.7525053323757,37.2108405096613,38.0818828920914));
#22460=CARTESIAN_POINT('Ctrl Pts',(-41.7532240407058,37.2120648891413,38.083280154769));
#22461=CARTESIAN_POINT('Ctrl Pts',(-41.7539427490358,37.2132892686213,38.0846774174467));
#22462=CARTESIAN_POINT('Ctrl Pts',(-41.7546609509386,37.2145145739489,38.0860741293221));
#22463=CARTESIAN_POINT('Ctrl Pts',(-41.7553786459012,37.2157408042489,38.0874702893979));
#22464=CARTESIAN_POINT('Ctrl Pts',(-41.7560963408638,37.2169670345488,38.0888664494737));
#22465=CARTESIAN_POINT('Ctrl Pts',(-41.7568135288862,37.2181941898211,38.0902620577498));
#22466=CARTESIAN_POINT('Ctrl Pts',(-41.7575302094561,37.2194222691894,38.0916571132293));
#22467=CARTESIAN_POINT('Ctrl Pts',(-41.7582468900261,37.2206503485575,38.0930521687089));
#22468=CARTESIAN_POINT('Ctrl Pts',(-41.7589630631436,37.2218793520216,38.094446671392));
#22469=CARTESIAN_POINT('Ctrl Pts',(-41.7596787282971,37.2231092787038,38.0958406202826));
#22470=CARTESIAN_POINT('Ctrl Pts',(-41.7603943934506,37.2243392053861,38.0972345691731));
#22471=CARTESIAN_POINT('Ctrl Pts',(-41.7611095506402,37.2255700552863,38.0986279642712));
#22472=CARTESIAN_POINT('Ctrl Pts',(-41.761824199355,37.2268018275256,38.1000208045815));
#22473=CARTESIAN_POINT('Ctrl Pts',(-41.7625388480698,37.2280335997649,38.1014136448918));
#22474=CARTESIAN_POINT('Ctrl Pts',(-41.7632529883098,37.2292662943431,38.1028059304144));
#22475=CARTESIAN_POINT('Ctrl Pts',(-41.763966619565,37.2304999103799,38.1041976601548));
#22476=CARTESIAN_POINT('Ctrl Pts',(-41.7646802508202,37.2317335264167,38.1055893898952));
#22477=CARTESIAN_POINT('Ctrl Pts',(-41.7653933730906,37.232968063912,38.1069805638536));
#22478=CARTESIAN_POINT('Ctrl Pts',(-41.7661059858668,37.2342035219841,38.108371181036));
#22479=CARTESIAN_POINT('Ctrl Pts',(-41.766818598643,37.2354389800562,38.1097617982186));
#22480=CARTESIAN_POINT('Ctrl Pts',(-41.767530701925,37.2366753587051,38.1111518586253));
#22481=CARTESIAN_POINT('Ctrl Pts',(-41.7682422952044,37.2379126570476,38.1125413612635));
#22482=CARTESIAN_POINT('Ctrl Pts',(-41.7689538884836,37.2391499553902,38.1139308639016));
#22483=CARTESIAN_POINT('Ctrl Pts',(-41.7696649717601,37.2403881734266,38.1153198087711));
#22484=CARTESIAN_POINT('Ctrl Pts',(-41.7703755445259,37.2416273102722,38.11670819488));
#22485=CARTESIAN_POINT('Ctrl Pts',(-41.7710861172917,37.2428664471179,38.1180965809888));
#22486=CARTESIAN_POINT('Ctrl Pts',(-41.7717961795469,37.2441065027729,38.119484408337));
#22487=CARTESIAN_POINT('Ctrl Pts',(-41.7725057307843,37.2453474763514,38.1208716759333));
#22488=CARTESIAN_POINT('Ctrl Pts',(-41.7732152820216,37.24658844993,38.1222589435297));
#22489=CARTESIAN_POINT('Ctrl Pts',(-41.7739243222412,37.2478303414323,38.1236456513741));
#22490=CARTESIAN_POINT('Ctrl Pts',(-41.7746328509364,37.2490731499712,38.1250317984762));
#22491=CARTESIAN_POINT('Ctrl Pts',(-41.7753413796317,37.2503159585101,38.1264179455783));
#22492=CARTESIAN_POINT('Ctrl Pts',(-41.7760493968028,37.2515596840855,38.1278035319381));
#22493=CARTESIAN_POINT('Ctrl Pts',(-41.7767569019439,37.2528043258094,38.1291885565659));
#22494=CARTESIAN_POINT('Ctrl Pts',(-41.7774644070851,37.2540489675332,38.1305735811937));
#22495=CARTESIAN_POINT('Ctrl Pts',(-41.7781714001963,37.2552945254054,38.1319580440895));
#22496=CARTESIAN_POINT('Ctrl Pts',(-41.7788778807726,37.2565409985362,38.1333419442646));
#22497=CARTESIAN_POINT('Ctrl Pts',(-41.7795843613489,37.257787471667,38.1347258444396));
#22498=CARTESIAN_POINT('Ctrl Pts',(-41.7802903293903,37.2590348600565,38.1361091818938));
#22499=CARTESIAN_POINT('Ctrl Pts',(-41.7809957843926,37.2602831628138,38.1374919556392));
#22500=CARTESIAN_POINT('Ctrl Pts',(-41.7284556368598,37.1796898657602,38.0513058194986));
#22501=CARTESIAN_POINT('Ctrl Pts',(-41.72944530003,37.1813261852412,38.0531959552349));
#22502=CARTESIAN_POINT('Ctrl Pts',(-41.7304341078028,37.1829640881581,38.0550851651249));
#22503=CARTESIAN_POINT('Ctrl Pts',(-41.7314220591106,37.1846035727302,38.0569734471179));
#22504=CARTESIAN_POINT('Ctrl Pts',(-41.7324091331635,37.186241601516,38.0588600524042));
#22505=CARTESIAN_POINT('Ctrl Pts',(-41.7333953522717,37.1878812091493,38.0607457314407));
#22506=CARTESIAN_POINT('Ctrl Pts',(-41.7343807153722,37.1895223938508,38.0626304821839));
#22507=CARTESIAN_POINT('Ctrl Pts',(-41.7353660784728,37.1911635785522,38.0645152329272));
#22508=CARTESIAN_POINT('Ctrl Pts',(-41.7363505855657,37.1928063403217,38.0663990553772));
#22509=CARTESIAN_POINT('Ctrl Pts',(-41.7373342355896,37.1944506773768,38.0682819474925));
#22510=CARTESIAN_POINT('Ctrl Pts',(-41.7383178856135,37.1960950144319,38.0701648396078));
#22511=CARTESIAN_POINT('Ctrl Pts',(-41.7393006785684,37.1977409267727,38.0720468013883));
#22512=CARTESIAN_POINT('Ctrl Pts',(-41.7402826133948,37.1993884126133,38.0739278307945));
#22513=CARTESIAN_POINT('Ctrl Pts',(-41.7412645482211,37.201035898454,38.0758088602006));
#22514=CARTESIAN_POINT('Ctrl Pts',(-41.7422456249189,37.2026849577945,38.0776889572324));
#22515=CARTESIAN_POINT('Ctrl Pts',(-41.7432258424304,37.204335588846,38.0795681198521));
#22516=CARTESIAN_POINT('Ctrl Pts',(-41.7442060599419,37.2059862198976,38.0814472824717));
#22517=CARTESIAN_POINT('Ctrl Pts',(-41.7451854182669,37.2076384226602,38.0833255106791));
#22518=CARTESIAN_POINT('Ctrl Pts',(-41.7461639163495,37.2092921953418,38.0852028024386));
#22519=CARTESIAN_POINT('Ctrl Pts',(-41.7471424144321,37.2109459680234,38.0870800941981));
#22520=CARTESIAN_POINT('Ctrl Pts',(-41.7481200522723,37.2126013106239,38.0889564495096));
#22521=CARTESIAN_POINT('Ctrl Pts',(-41.7490968288155,37.2142582213483,38.090831866339));
#22522=CARTESIAN_POINT('Ctrl Pts',(-41.7500736053588,37.2159151320727,38.0927072831685));
#22523=CARTESIAN_POINT('Ctrl Pts',(-41.7510495206052,37.2175736109209,38.0945817615159));
#22524=CARTESIAN_POINT('Ctrl Pts',(-41.7520245735021,37.2192336560945,38.0964552993493));
#22525=CARTESIAN_POINT('Ctrl Pts',(-41.752999626399,37.2208937012682,38.0983288371826));
#22526=CARTESIAN_POINT('Ctrl Pts',(-41.7539738169465,37.2225553127673,38.1002014345018));
#22527=CARTESIAN_POINT('Ctrl Pts',(-41.7549471440936,37.2242184887904,38.1020730892768));
#22528=CARTESIAN_POINT('Ctrl Pts',(-41.7559204712406,37.2258816648134,38.1039447440518));
#22529=CARTESIAN_POINT('Ctrl Pts',(-41.7568929349873,37.2275464053604,38.1058154562824));
#22530=CARTESIAN_POINT('Ctrl Pts',(-41.7578645342845,37.2292127086268,38.1076852239405));
#22531=CARTESIAN_POINT('Ctrl Pts',(-41.7588361335817,37.230879011893,38.1095549915986));
#22532=CARTESIAN_POINT('Ctrl Pts',(-41.7598068684293,37.2325468778786,38.1114238146841));
#22533=CARTESIAN_POINT('Ctrl Pts',(-41.76077673778,37.2342163047757,38.1132916911706));
#22534=CARTESIAN_POINT('Ctrl Pts',(-41.7617466071307,37.2358857316728,38.1151595676571));
#22535=CARTESIAN_POINT('Ctrl Pts',(-41.7627156109845,37.2375567194813,38.1170264975447));
#22536=CARTESIAN_POINT('Ctrl Pts',(-41.7636837482957,37.2392292663904,38.1188924788088));
#22537=CARTESIAN_POINT('Ctrl Pts',(-41.7646518856068,37.2409018132995,38.1207584600729));
#22538=CARTESIAN_POINT('Ctrl Pts',(-41.7656191563754,37.2425759193091,38.1226234927135));
#22539=CARTESIAN_POINT('Ctrl Pts',(-41.7665855595574,37.2442515826052,38.1244875747081));
#22540=CARTESIAN_POINT('Ctrl Pts',(-41.7675519627395,37.2459272459012,38.1263516567027));
#22541=CARTESIAN_POINT('Ctrl Pts',(-41.768517498335,37.2476044664838,38.1282147880512));
#22542=CARTESIAN_POINT('Ctrl Pts',(-41.7694821653018,37.2492832425355,38.1300769667331));
#22543=CARTESIAN_POINT('Ctrl Pts',(-41.7704468322687,37.2509620185871,38.131939145415));
#22544=CARTESIAN_POINT('Ctrl Pts',(-41.7714106306068,37.2526423501081,38.1338003714302));
#22545=CARTESIAN_POINT('Ctrl Pts',(-41.7723735592759,37.2543242352779,38.1356606427601));
#22546=CARTESIAN_POINT('Ctrl Pts',(-41.7733364879449,37.2560061204476,38.1375209140899));
#22547=CARTESIAN_POINT('Ctrl Pts',(-41.7742985469448,37.2576895592663,38.1393802307343));
#22548=CARTESIAN_POINT('Ctrl Pts',(-41.775259735237,37.2593745499102,38.1412385906764));
#22549=CARTESIAN_POINT('Ctrl Pts',(-41.7091602750971,37.1578460913556,38.0313362231075));
#22550=CARTESIAN_POINT('Ctrl Pts',(-41.7104420238158,37.1599035150217,38.0337310951134));
#22551=CARTESIAN_POINT('Ctrl Pts',(-41.7117223763588,37.1619635480723,38.0361244614683));
#22552=CARTESIAN_POINT('Ctrl Pts',(-41.7130013305215,37.1640261868666,38.0385163179722));
#22553=CARTESIAN_POINT('Ctrl Pts',(-41.7142791490322,37.1660869941335,38.0409060506185));
#22554=CARTESIAN_POINT('Ctrl Pts',(-41.7155555716447,37.1681504025185,38.0432942760941));
#22555=CARTESIAN_POINT('Ctrl Pts',(-41.7168305961639,37.1702164083836,38.0456809902143));
#22556=CARTESIAN_POINT('Ctrl Pts',(-41.7181056206831,37.1722824142486,38.0480677043346));
#22557=CARTESIAN_POINT('Ctrl Pts',(-41.719379247109,37.1743510175936,38.0504529070995));
#22558=CARTESIAN_POINT('Ctrl Pts',(-41.7206514732504,37.1764222147733,38.0528365943289));
#22559=CARTESIAN_POINT('Ctrl Pts',(-41.7219236993918,37.178493411953,38.0552202815582));
#22560=CARTESIAN_POINT('Ctrl Pts',(-41.7231945252486,37.1805672029672,38.0576024532521));
#22561=CARTESIAN_POINT('Ctrl Pts',(-41.7244639486337,37.1826435841636,38.0599831052344));
#22562=CARTESIAN_POINT('Ctrl Pts',(-41.7257333720188,37.18471996536,38.0623637572168));
#22563=CARTESIAN_POINT('Ctrl Pts',(-41.727001392932,37.1867989367385,38.0647428894876));
#22564=CARTESIAN_POINT('Ctrl Pts',(-41.7282680091901,37.1888804946396,38.0671204978753));
#22565=CARTESIAN_POINT('Ctrl Pts',(-41.7295346254482,37.1909620525406,38.069498106263));
#22566=CARTESIAN_POINT('Ctrl Pts',(-41.7307998370511,37.1930461969642,38.0718741907675));
#22567=CARTESIAN_POINT('Ctrl Pts',(-41.7320636418194,37.1951329242436,38.0742487472214));
#22568=CARTESIAN_POINT('Ctrl Pts',(-41.7333274465877,37.1972196515231,38.0766233036752));
#22569=CARTESIAN_POINT('Ctrl Pts',(-41.7345898445214,37.1993089616584,38.0789963320785));
#22570=CARTESIAN_POINT('Ctrl Pts',(-41.7358508334449,37.2014008509757,38.081367828268));
#22571=CARTESIAN_POINT('Ctrl Pts',(-41.7371118223684,37.203492740293,38.0837393244575));
#22572=CARTESIAN_POINT('Ctrl Pts',(-41.7383714022818,37.2055872087923,38.0861092884332));
#22573=CARTESIAN_POINT('Ctrl Pts',(-41.7396295710134,37.2076842527928,38.0884777160364));
#22574=CARTESIAN_POINT('Ctrl Pts',(-41.740887739745,37.2097812967933,38.0908461436395));
#22575=CARTESIAN_POINT('Ctrl Pts',(-41.7421444972949,37.211880916295,38.09321303487));
#22576=CARTESIAN_POINT('Ctrl Pts',(-41.7433998414954,37.2139831076097,38.0955783855734));
#22577=CARTESIAN_POINT('Ctrl Pts',(-41.7446551856959,37.2160852989245,38.0979437362768));
#22578=CARTESIAN_POINT('Ctrl Pts',(-41.745909116547,37.2181900620525,38.100307546453));
#22579=CARTESIAN_POINT('Ctrl Pts',(-41.7471616318849,37.2202973932986,38.1026698119518));
#22580=CARTESIAN_POINT('Ctrl Pts',(-41.7484141472228,37.2224047245446,38.1050320774506));
#22581=CARTESIAN_POINT('Ctrl Pts',(-41.7496652470475,37.2245146239088,38.1073927982719));
#22582=CARTESIAN_POINT('Ctrl Pts',(-41.7509149291994,37.2266270876888,38.1097519702699));
#22583=CARTESIAN_POINT('Ctrl Pts',(-41.7521646113512,37.2287395514689,38.112111142268));
#22584=CARTESIAN_POINT('Ctrl Pts',(-41.7534128758301,37.230854579665,38.1144687654425));
#22585=CARTESIAN_POINT('Ctrl Pts',(-41.7546597204802,37.2329721685677,38.1168248356522));
#22586=CARTESIAN_POINT('Ctrl Pts',(-41.7559065651303,37.2350897574705,38.1191809058618));
#22587=CARTESIAN_POINT('Ctrl Pts',(-41.7571519899515,37.23720990708,38.1215354231064));
#22588=CARTESIAN_POINT('Ctrl Pts',(-41.7583959927921,37.23933261368,38.1238883832486));
#22589=CARTESIAN_POINT('Ctrl Pts',(-41.7596399956326,37.2414553202799,38.1262413433909));
#22590=CARTESIAN_POINT('Ctrl Pts',(-41.7608825764924,37.2435805838703,38.1285927464307));
#22591=CARTESIAN_POINT('Ctrl Pts',(-41.7621237332236,37.2457084007279,38.1309425882353));
#22592=CARTESIAN_POINT('Ctrl Pts',(-41.7633648899547,37.2478362175854,38.1332924300399));
#22593=CARTESIAN_POINT('Ctrl Pts',(-41.7646046225571,37.24996658771,38.1356407106091));
#22594=CARTESIAN_POINT('Ctrl Pts',(-41.7658429288868,37.2520995073713,38.1379874258143));
#22595=CARTESIAN_POINT('Ctrl Pts',(-41.7670812352165,37.2542324270326,38.1403341410195));
#22596=CARTESIAN_POINT('Ctrl Pts',(-41.7683181152735,37.2563678962306,38.1426792908607));
#22597=CARTESIAN_POINT('Ctrl Pts',(-41.7695535669177,37.2585059112279,38.1450228712136));
#22598=CARTESIAN_POINT('Ctrl Pts',(-41.6889393053371,37.1357612177105,38.0109524721443));
#22599=CARTESIAN_POINT('Ctrl Pts',(-41.6905364576388,37.1382386034432,38.0138650725638));
#22600=CARTESIAN_POINT('Ctrl Pts',(-41.6921314669563,37.1407200717346,38.0167753755858));
#22601=CARTESIAN_POINT('Ctrl Pts',(-41.6937243283598,37.1432056149149,38.019683372215));
#22602=CARTESIAN_POINT('Ctrl Pts',(-41.6953157753764,37.1456889510481,38.0225887866781));
#22603=CARTESIAN_POINT('Ctrl Pts',(-41.6969050782917,37.1481763548368,38.0254918988425));
#22604=CARTESIAN_POINT('Ctrl Pts',(-41.6984922322021,37.1506678186063,38.0283926997509));
#22605=CARTESIAN_POINT('Ctrl Pts',(-41.7000793861125,37.1531592823757,38.0312935006593));
#22606=CARTESIAN_POINT('Ctrl Pts',(-41.701664391018,37.1556548061259,38.0341919903117));
#22607=CARTESIAN_POINT('Ctrl Pts',(-41.7032472420284,37.1581543821572,38.0370881597651));
#22608=CARTESIAN_POINT('Ctrl Pts',(-41.7048300930387,37.1606539581885,38.0399843292186));
#22609=CARTESIAN_POINT('Ctrl Pts',(-41.7064107901537,37.1631575865009,38.042878178473));
#22610=CARTESIAN_POINT('Ctrl Pts',(-41.7079893284965,37.1656652593697,38.0457696985998));
#22611=CARTESIAN_POINT('Ctrl Pts',(-41.7095678668393,37.1681729322385,38.0486612187265));
#22612=CARTESIAN_POINT('Ctrl Pts',(-41.7111442464097,37.1706846496637,38.0515504097256));
#22613=CARTESIAN_POINT('Ctrl Pts',(-41.7127184623441,37.1732004038957,38.0544372626828));
#22614=CARTESIAN_POINT('Ctrl Pts',(-41.7142926782785,37.1757161581277,38.0573241156399));
#22615=CARTESIAN_POINT('Ctrl Pts',(-41.7158647305767,37.1782359491665,38.0602086305551));
#22616=CARTESIAN_POINT('Ctrl Pts',(-41.7174346143886,37.1807597692374,38.0630907985285));
#22617=CARTESIAN_POINT('Ctrl Pts',(-41.7190044982004,37.1832835893083,38.0659729665019));
#22618=CARTESIAN_POINT('Ctrl Pts',(-41.7205722135258,37.1858114384115,38.0688527875335));
#22619=CARTESIAN_POINT('Ctrl Pts',(-41.7221377555276,37.1883433087475,38.0717302527378));
#22620=CARTESIAN_POINT('Ctrl Pts',(-41.7237032975295,37.1908751790835,38.0746077179421));
#22621=CARTESIAN_POINT('Ctrl Pts',(-41.7252666662079,37.1934110706522,38.0774828273193));
#22622=CARTESIAN_POINT('Ctrl Pts',(-41.7268278567391,37.1959509756296,38.0803555719983));
#22623=CARTESIAN_POINT('Ctrl Pts',(-41.7283890472704,37.198490880607,38.0832283166774));
#22624=CARTESIAN_POINT('Ctrl Pts',(-41.7299480596546,37.2010347989929,38.0860986966584));
#22625=CARTESIAN_POINT('Ctrl Pts',(-41.7315048890814,37.2035827229384,38.0889667030851));
#22626=CARTESIAN_POINT('Ctrl Pts',(-41.7330617185083,37.2061306468839,38.0918347095118));
#22627=CARTESIAN_POINT('Ctrl Pts',(-41.7346163649779,37.208682576389,38.0947003423842));
#22628=CARTESIAN_POINT('Ctrl Pts',(-41.7361688236936,37.2112385035799,38.0975635928606));
#22629=CARTESIAN_POINT('Ctrl Pts',(-41.7377212824092,37.2137944307708,38.1004268433371));
#22630=CARTESIAN_POINT('Ctrl Pts',(-41.7392715533709,37.2163543556476,38.1032877114176));
#22631=CARTESIAN_POINT('Ctrl Pts',(-41.7408196317953,37.2189182703119,38.1061461882752));
#22632=CARTESIAN_POINT('Ctrl Pts',(-41.7423677102199,37.2214821849762,38.1090046651329));
#22633=CARTESIAN_POINT('Ctrl Pts',(-41.7439135961072,37.224050089428,38.1118607507677));
#22634=CARTESIAN_POINT('Ctrl Pts',(-41.7454572846877,37.2266219757442,38.1147144363676));
#22635=CARTESIAN_POINT('Ctrl Pts',(-41.7470009732681,37.2291938620605,38.1175681219675));
#22636=CARTESIAN_POINT('Ctrl Pts',(-41.7485424645417,37.2317697302412,38.1204194075323));
#22637=CARTESIAN_POINT('Ctrl Pts',(-41.7500817537524,37.2343495723389,38.1232682842648));
#22638=CARTESIAN_POINT('Ctrl Pts',(-41.7516210429631,37.2369294144365,38.1261171609973));
#22639=CARTESIAN_POINT('Ctrl Pts',(-41.7531581301108,37.2395132304511,38.1289636288975));
#22640=CARTESIAN_POINT('Ctrl Pts',(-41.7546930104531,37.2421010124104,38.1318076791829));
#22641=CARTESIAN_POINT('Ctrl Pts',(-41.7562278907953,37.2446887943699,38.1346517294682));
#22642=CARTESIAN_POINT('Ctrl Pts',(-41.7577605643321,37.247280542274,38.1374933621388));
#22643=CARTESIAN_POINT('Ctrl Pts',(-41.7592910263345,37.2498762481265,38.140332568427));
#22644=CARTESIAN_POINT('Ctrl Pts',(-41.7608214883369,37.2524719539789,38.1431717747151));
#22645=CARTESIAN_POINT('Ctrl Pts',(-41.7623497388049,37.2550716177796,38.1460085546209));
#22646=CARTESIAN_POINT('Ctrl Pts',(-41.7638757730233,37.2576752315076,38.1488428993918));
#22647=CARTESIAN_POINT('Ctrl Pts',(-41.6687183355772,37.1136763440655,37.9905687211811));
#22648=CARTESIAN_POINT('Ctrl Pts',(-41.6706308914618,37.1165736918647,37.9939990500142));
#22649=CARTESIAN_POINT('Ctrl Pts',(-41.6725405575538,37.119476595397,37.9974262897033));
#22650=CARTESIAN_POINT('Ctrl Pts',(-41.6744473261982,37.1223850429631,38.0008504264578));
#22651=CARTESIAN_POINT('Ctrl Pts',(-41.6763524017206,37.1252909079628,38.0042715227377));
#22652=CARTESIAN_POINT('Ctrl Pts',(-41.6782545849386,37.1282023071551,38.007689521591));
#22653=CARTESIAN_POINT('Ctrl Pts',(-41.6801538682403,37.1311192288289,38.0111044092876));
#22654=CARTESIAN_POINT('Ctrl Pts',(-41.6820531515419,37.1340361505028,38.0145192969841));
#22655=CARTESIAN_POINT('Ctrl Pts',(-41.6839495349271,37.1369585946581,38.017931073524));
#22656=CARTESIAN_POINT('Ctrl Pts',(-41.6858430108064,37.1398865495411,38.0213397252014));
#22657=CARTESIAN_POINT('Ctrl Pts',(-41.6877364866856,37.1428145044241,38.0247483768789));
#22658=CARTESIAN_POINT('Ctrl Pts',(-41.6896270550588,37.1457479700346,38.0281539036939));
#22659=CARTESIAN_POINT('Ctrl Pts',(-41.6915147083593,37.1486869345758,38.0315562919651));
#22660=CARTESIAN_POINT('Ctrl Pts',(-41.6934023616597,37.1516258991171,38.0349586802362));
#22661=CARTESIAN_POINT('Ctrl Pts',(-41.6952870998874,37.154570362589,38.0383579299636));
#22662=CARTESIAN_POINT('Ctrl Pts',(-41.697168915498,37.1575203131519,38.0417540274902));
#22663=CARTESIAN_POINT('Ctrl Pts',(-41.6990507311087,37.1604702637148,38.0451501250169));
#22664=CARTESIAN_POINT('Ctrl Pts',(-41.7009296241024,37.1634257013687,38.0485430703428));
#22665=CARTESIAN_POINT('Ctrl Pts',(-41.7028055869577,37.1663866142312,38.0519328498357));
#22666=CARTESIAN_POINT('Ctrl Pts',(-41.7046815498131,37.1693475270936,38.0553226293286));
#22667=CARTESIAN_POINT('Ctrl Pts',(-41.7065545825302,37.1723139151648,38.0587092429884));
#22668=CARTESIAN_POINT('Ctrl Pts',(-41.7084246776104,37.1752857665193,38.0620926772076));
#22669=CARTESIAN_POINT('Ctrl Pts',(-41.7102947726906,37.178257617874,38.0654761114268));
#22670=CARTESIAN_POINT('Ctrl Pts',(-41.712161930134,37.1812349325122,38.0688563662053));
#22671=CARTESIAN_POINT('Ctrl Pts',(-41.7140261424648,37.1842176984664,38.0722334279603));
#22672=CARTESIAN_POINT('Ctrl Pts',(-41.7158903547957,37.1872004644206,38.0756104897153));
#22673=CARTESIAN_POINT('Ctrl Pts',(-41.7177516220142,37.1901886816908,38.0789843584468));
#22674=CARTESIAN_POINT('Ctrl Pts',(-41.7196099366675,37.193182338267,38.0823550205968));
#22675=CARTESIAN_POINT('Ctrl Pts',(-41.7214682513208,37.1961759948432,38.0857256827468));
#22676=CARTESIAN_POINT('Ctrl Pts',(-41.7233236134089,37.1991750907254,38.0890931383153));
#22677=CARTESIAN_POINT('Ctrl Pts',(-41.7251760155023,37.2021796138613,38.0924573737694));
#22678=CARTESIAN_POINT('Ctrl Pts',(-41.7270284175957,37.205184136997,38.0958216092235));
#22679=CARTESIAN_POINT('Ctrl Pts',(-41.7288778596942,37.2081940873865,38.0991826245632));
#22680=CARTESIAN_POINT('Ctrl Pts',(-41.7307243343914,37.211209452935,38.1025404062805));
#22681=CARTESIAN_POINT('Ctrl Pts',(-41.7325708090885,37.2142248184835,38.1058981879979));
#22682=CARTESIAN_POINT('Ctrl Pts',(-41.7344143163842,37.217245599191,38.1092527360929));
#22683=CARTESIAN_POINT('Ctrl Pts',(-41.7362548488951,37.2202717829207,38.112604037083));
#22684=CARTESIAN_POINT('Ctrl Pts',(-41.738095381406,37.2232979666505,38.1159553380731));
#22685=CARTESIAN_POINT('Ctrl Pts',(-41.739932939132,37.2263295534024,38.1193033919582));
#22686=CARTESIAN_POINT('Ctrl Pts',(-41.7417675147128,37.2293665309978,38.122648185281));
#22687=CARTESIAN_POINT('Ctrl Pts',(-41.7436020902936,37.2324035085931,38.1259929786038));
#22688=CARTESIAN_POINT('Ctrl Pts',(-41.7454336837292,37.2354458770318,38.1293345113643));
#22689=CARTESIAN_POINT('Ctrl Pts',(-41.7472622876826,37.2384936240931,38.1326727701304));
#22690=CARTESIAN_POINT('Ctrl Pts',(-41.749090891636,37.2415413711543,38.1360110288966));
#22691=CARTESIAN_POINT('Ctrl Pts',(-41.7509165061071,37.2445944968381,38.1393460136685));
#22692=CARTESIAN_POINT('Ctrl Pts',(-41.7527391237821,37.2476529888817,38.1426777110396));
#22693=CARTESIAN_POINT('Ctrl Pts',(-41.7545617414572,37.2507114809253,38.1460094084107));
#22694=CARTESIAN_POINT('Ctrl Pts',(-41.7563813623363,37.2537753393287,38.1493378183811));
#22695=CARTESIAN_POINT('Ctrl Pts',(-41.7581979791288,37.2568445517873,38.1526629275699));
#22696=CARTESIAN_POINT('Ctrl Pts',(-41.6475728892226,37.0913544340564,37.969773861755));
#22697=CARTESIAN_POINT('Ctrl Pts',(-41.6498241513043,37.0946704940769,37.9737348553367));
#22698=CARTESIAN_POINT('Ctrl Pts',(-41.6520715703113,37.0979940317792,37.9776917557169));
#22699=CARTESIAN_POINT('Ctrl Pts',(-41.6543151342611,37.1013250292433,37.9816445416399));
#22700=CARTESIAN_POINT('Ctrl Pts',(-41.6565567060304,37.1046530689362,37.9855938176725));
#22701=CARTESIAN_POINT('Ctrl Pts',(-41.6587944295858,37.1079885551487,37.9895389865515));
#22702=CARTESIAN_POINT('Ctrl Pts',(-41.6610282930162,37.1113314699335,37.9934800271196));
#22703=CARTESIAN_POINT('Ctrl Pts',(-41.6632621564465,37.1146743847181,37.9974210676877));
#22704=CARTESIAN_POINT('Ctrl Pts',(-41.6654921597517,37.1180247280751,38.0013579799447));
#22705=CARTESIAN_POINT('Ctrl Pts',(-41.6677182910599,37.1213824819817,38.0052907427754));
#22706=CARTESIAN_POINT('Ctrl Pts',(-41.6699444223679,37.1247402358884,38.009223505606));
#22707=CARTESIAN_POINT('Ctrl Pts',(-41.6721666816788,37.128105400345,38.01315211901));
#22708=CARTESIAN_POINT('Ctrl Pts',(-41.6743850571597,37.1314779572543,38.0170765619143));
#22709=CARTESIAN_POINT('Ctrl Pts',(-41.6766034326405,37.1348505141636,38.0210010048186));
#22710=CARTESIAN_POINT('Ctrl Pts',(-41.6788179242914,37.1382304635258,38.024921277223));
#22711=CARTESIAN_POINT('Ctrl Pts',(-41.6810285203188,37.1416177871692,38.0288373580966));
#22712=CARTESIAN_POINT('Ctrl Pts',(-41.6832391163462,37.1450051108127,38.0327534389702));
#22713=CARTESIAN_POINT('Ctrl Pts',(-41.68544581675,37.1483998087376,38.0366653283129));
#22714=CARTESIAN_POINT('Ctrl Pts',(-41.6876486097765,37.1518018626979,38.0405730051363));
#22715=CARTESIAN_POINT('Ctrl Pts',(-41.6898514028029,37.1552039166582,38.0444806819597));
#22716=CARTESIAN_POINT('Ctrl Pts',(-41.6920502884518,37.1586133266541,38.0483841462638));
#22717=CARTESIAN_POINT('Ctrl Pts',(-41.6942452550088,37.1620300743655,38.0522833771027));
#22718=CARTESIAN_POINT('Ctrl Pts',(-41.6964402215659,37.165446822077,38.0561826079417));
#22719=CARTESIAN_POINT('Ctrl Pts',(-41.6986312690311,37.168870907504,38.0600776053155));
#22720=CARTESIAN_POINT('Ctrl Pts',(-41.7008183857296,37.1723023122527,38.0639683483214));
#22721=CARTESIAN_POINT('Ctrl Pts',(-41.7030055024282,37.1757337170013,38.0678590913274));
#22722=CARTESIAN_POINT('Ctrl Pts',(-41.7051886883601,37.1791724410717,38.0717455799653));
#22723=CARTESIAN_POINT('Ctrl Pts',(-41.7073679318905,37.1826184659959,38.0756277933756));
#22724=CARTESIAN_POINT('Ctrl Pts',(-41.7095471754209,37.1860644909201,38.0795100067858));
#22725=CARTESIAN_POINT('Ctrl Pts',(-41.7117224765497,37.1895178166982,38.0833879449684));
#22726=CARTESIAN_POINT('Ctrl Pts',(-41.713893823682,37.1929784247889,38.0872615871069));
#22727=CARTESIAN_POINT('Ctrl Pts',(-41.7160651708142,37.1964390328797,38.0911352292454));
#22728=CARTESIAN_POINT('Ctrl Pts',(-41.7182325639499,37.1999069232829,38.0950045753397));
#22729=CARTESIAN_POINT('Ctrl Pts',(-41.720395991534,37.2033820773839,38.098869604617));
#22730=CARTESIAN_POINT('Ctrl Pts',(-41.7225594191181,37.2068572314848,38.1027346338944));
#22731=CARTESIAN_POINT('Ctrl Pts',(-41.7247188811506,37.2103396492834,38.1065953463546));
#22732=CARTESIAN_POINT('Ctrl Pts',(-41.7268743661166,37.2138293120917,38.1104517212686));
#22733=CARTESIAN_POINT('Ctrl Pts',(-41.7290298510826,37.2173189748999,38.1143080961826));
#22734=CARTESIAN_POINT('Ctrl Pts',(-41.7311813589821,37.2208158827178,38.1181601335503));
#22735=CARTESIAN_POINT('Ctrl Pts',(-41.7333288783403,37.224320016784,38.1220078126863));
#22736=CARTESIAN_POINT('Ctrl Pts',(-41.7354763976986,37.2278241508502,38.1258554918223));
#22737=CARTESIAN_POINT('Ctrl Pts',(-41.7376199285156,37.2313355111647,38.1296988127267));
#22738=CARTESIAN_POINT('Ctrl Pts',(-41.7397594593571,37.2348540788934,38.1335377547582));
#22739=CARTESIAN_POINT('Ctrl Pts',(-41.7418989901986,37.238372646622,38.1373766967897));
#22740=CARTESIAN_POINT('Ctrl Pts',(-41.7440345210644,37.2418984217649,38.1412112599481));
#22741=CARTESIAN_POINT('Ctrl Pts',(-41.7461660405608,37.2454313854149,38.1450414236367));
#22742=CARTESIAN_POINT('Ctrl Pts',(-41.7482975600572,37.2489643490649,38.1488715873253));
#22743=CARTESIAN_POINT('Ctrl Pts',(-41.750425068184,37.2525045012221,38.1526973515439));
#22744=CARTESIAN_POINT('Ctrl Pts',(-41.7525485535879,37.256051822907,38.15651869574));
#22745=CARTESIAN_POINT('Ctrl Pts',(-41.6257141900876,37.0691011556449,37.9488313498428));
#22746=CARTESIAN_POINT('Ctrl Pts',(-41.6283229847769,37.0728276862717,37.9533303089943));
#22747=CARTESIAN_POINT('Ctrl Pts',(-41.6309267846842,37.0765641067473,37.9578239725956));
#22748=CARTESIAN_POINT('Ctrl Pts',(-41.6335255706247,37.0803103895415,37.9623123075375));
#22749=CARTESIAN_POINT('Ctrl Pts',(-41.636122048964,37.0840533458105,37.9667966570464));
#22750=CARTESIAN_POINT('Ctrl Pts',(-41.6387135222368,37.0878061468915,37.9712756873548));
#22751=CARTESIAN_POINT('Ctrl Pts',(-41.6412999713831,37.0915687651826,37.9757493655199));
#22752=CARTESIAN_POINT('Ctrl Pts',(-41.6438864205294,37.0953313834738,37.9802230436849));
#22753=CARTESIAN_POINT('Ctrl Pts',(-41.6464678455491,37.0991038189753,37.9846913697065));
#22754=CARTESIAN_POINT('Ctrl Pts',(-41.6490442274561,37.1028860439409,37.9891543107205));
#22755=CARTESIAN_POINT('Ctrl Pts',(-41.6516206093631,37.1066682689066,37.9936172517345));
#22756=CARTESIAN_POINT('Ctrl Pts',(-41.6541919481574,37.1104602833365,37.9980748077408));
#22757=CARTESIAN_POINT('Ctrl Pts',(-41.6567582249268,37.1142620593407,38.0025269459543));
#22758=CARTESIAN_POINT('Ctrl Pts',(-41.6593245016963,37.1180638353448,38.006979084168));
#22759=CARTESIAN_POINT('Ctrl Pts',(-41.6618857164409,37.1218753729231,38.0114258045888));
#22760=CARTESIAN_POINT('Ctrl Pts',(-41.6644418503232,37.1256966440421,38.0158670745116));
#22761=CARTESIAN_POINT('Ctrl Pts',(-41.6669979842055,37.1295179151611,38.0203083444344));
#22762=CARTESIAN_POINT('Ctrl Pts',(-41.6695490372254,37.1333489198205,38.0247441638592));
#22763=CARTESIAN_POINT('Ctrl Pts',(-41.6720949906201,37.1371896298438,38.0291745001607));
#22764=CARTESIAN_POINT('Ctrl Pts',(-41.6746409440149,37.1410303398672,38.0336048364622));
#22765=CARTESIAN_POINT('Ctrl Pts',(-41.6771817977843,37.1448807552543,38.0380296896405));
#22766=CARTESIAN_POINT('Ctrl Pts',(-41.6797175332409,37.1487408476856,38.042449027151));
#22767=CARTESIAN_POINT('Ctrl Pts',(-41.6822532686974,37.152600940117,38.0468683646616));
#22768=CARTESIAN_POINT('Ctrl Pts',(-41.6847838858408,37.1564707095926,38.0512821865043));
#22769=CARTESIAN_POINT('Ctrl Pts',(-41.6873093660587,37.1603501276504,38.055690460216));
#22770=CARTESIAN_POINT('Ctrl Pts',(-41.6898348462767,37.1642295457083,38.0600987339277));
#22771=CARTESIAN_POINT('Ctrl Pts',(-41.6923551895691,37.1681186123485,38.0645014595082));
#22772=CARTESIAN_POINT('Ctrl Pts',(-41.6948703773989,37.1720172989672,38.0688986045758));
#22773=CARTESIAN_POINT('Ctrl Pts',(-41.6973855652288,37.1759159855859,38.0732957496434));
#22774=CARTESIAN_POINT('Ctrl Pts',(-41.6998955975961,37.179824292183,38.0776873141981));
#22775=CARTESIAN_POINT('Ctrl Pts',(-41.7024004560398,37.1837421900134,38.0820732659402));
#22776=CARTESIAN_POINT('Ctrl Pts',(-41.7049053144835,37.1876600878437,38.0864592176823));
#22777=CARTESIAN_POINT('Ctrl Pts',(-41.7074049990036,37.1915875769071,38.0908395566119));
#22778=CARTESIAN_POINT('Ctrl Pts',(-41.7098994912149,37.1955246283172,38.0952142505117));
#22779=CARTESIAN_POINT('Ctrl Pts',(-41.7123939834263,37.1994616797273,38.0995889444116));
#22780=CARTESIAN_POINT('Ctrl Pts',(-41.714883283329,37.2034082934841,38.1039579932818));
#22781=CARTESIAN_POINT('Ctrl Pts',(-41.7173673726144,37.2073644405605,38.1083213649881));
#22782=CARTESIAN_POINT('Ctrl Pts',(-41.7198514618998,37.2113205876369,38.1126847366945));
#22783=CARTESIAN_POINT('Ctrl Pts',(-41.7223303405679,37.2152862680329,38.1170424312371));
#22784=CARTESIAN_POINT('Ctrl Pts',(-41.7248039903866,37.2192614525812,38.1213944165653));
#22785=CARTESIAN_POINT('Ctrl Pts',(-41.7272776402054,37.2232366371295,38.1257464018935));
#22786=CARTESIAN_POINT('Ctrl Pts',(-41.7297460611749,37.22722132583,38.1300926780074));
#22787=CARTESIAN_POINT('Ctrl Pts',(-41.7322092351399,37.2312154893756,38.1344332129404));
#22788=CARTESIAN_POINT('Ctrl Pts',(-41.734672409105,37.2352096529214,38.1387737478733));
#22789=CARTESIAN_POINT('Ctrl Pts',(-41.7371303360657,37.2392132913121,38.1431085416253));
#22790=CARTESIAN_POINT('Ctrl Pts',(-41.7395829979441,37.2432263751015,38.1474375623142));
#22791=CARTESIAN_POINT('Ctrl Pts',(-41.7420356598224,37.247239458891,38.1517665830032));
#22792=CARTESIAN_POINT('Ctrl Pts',(-41.7444830566185,37.251261988079,38.156089830629));
#22793=CARTESIAN_POINT('Ctrl Pts',(-41.7469251703319,37.2552939330803,38.1604072733946));
#22794=CARTESIAN_POINT('Ctrl Pts',(-41.6038554909526,37.0468478772333,37.9278888379305));
#22795=CARTESIAN_POINT('Ctrl Pts',(-41.6068218182495,37.0509848784665,37.9329257626518));
#22796=CARTESIAN_POINT('Ctrl Pts',(-41.6097819990572,37.0551341817153,37.9379561894743));
#22797=CARTESIAN_POINT('Ctrl Pts',(-41.6127360069883,37.0592957498397,37.9429800734352));
#22798=CARTESIAN_POINT('Ctrl Pts',(-41.6156873918975,37.063453622685,37.9479994964203));
#22799=CARTESIAN_POINT('Ctrl Pts',(-41.6186326148878,37.0676237386342,37.9530123881581));
#22800=CARTESIAN_POINT('Ctrl Pts',(-41.62157164975,37.0718060604318,37.9580187039201));
#22801=CARTESIAN_POINT('Ctrl Pts',(-41.6245106846123,37.0759883822295,37.9630250196822));
#22802=CARTESIAN_POINT('Ctrl Pts',(-41.6274435313465,37.0801829098755,37.9680247594683));
#22803=CARTESIAN_POINT('Ctrl Pts',(-41.6303701638525,37.0843896059001,37.9730178786657));
#22804=CARTESIAN_POINT('Ctrl Pts',(-41.6332967963584,37.0885963019248,37.978010997863));
#22805=CARTESIAN_POINT('Ctrl Pts',(-41.6362172146359,37.0928151663281,37.9829974964715));
#22806=CARTESIAN_POINT('Ctrl Pts',(-41.639131392694,37.0970461614271,37.9879773299944));
#22807=CARTESIAN_POINT('Ctrl Pts',(-41.642045570752,37.1012771565259,37.9929571635173));
#22808=CARTESIAN_POINT('Ctrl Pts',(-41.6449535085904,37.1055202823205,37.9979303319545));
#22809=CARTESIAN_POINT('Ctrl Pts',(-41.6478551803277,37.1097755009149,38.0028967909266));
#22810=CARTESIAN_POINT('Ctrl Pts',(-41.6507568520649,37.1140307195093,38.0078632498987));
#22811=CARTESIAN_POINT('Ctrl Pts',(-41.6536522577008,37.1182980309035,38.0128229994054));
#22812=CARTESIAN_POINT('Ctrl Pts',(-41.6565413714638,37.1225773969899,38.017775995185));
#22813=CARTESIAN_POINT('Ctrl Pts',(-41.6594304852268,37.1268567630762,38.0227289909647));
#22814=CARTESIAN_POINT('Ctrl Pts',(-41.6623133071169,37.1311481838545,38.0276752330172));
#22815=CARTESIAN_POINT('Ctrl Pts',(-41.6651898114729,37.1354516210057,38.0326146771993));
#22816=CARTESIAN_POINT('Ctrl Pts',(-41.6680663158288,37.139755058157,38.0375541213814));
#22817=CARTESIAN_POINT('Ctrl Pts',(-41.6709365026506,37.1440705116811,38.0424867676931));
#22818=CARTESIAN_POINT('Ctrl Pts',(-41.6738003463879,37.1483979430482,38.0474125721105));
#22819=CARTESIAN_POINT('Ctrl Pts',(-41.6766641901252,37.1527253744153,38.0523383765279));
#22820=CARTESIAN_POINT('Ctrl Pts',(-41.679521690778,37.1570647836254,38.057257339051));
#22821=CARTESIAN_POINT('Ctrl Pts',(-41.6823728229074,37.1614161319385,38.062169415776));
#22822=CARTESIAN_POINT('Ctrl Pts',(-41.6852239550367,37.1657674802517,38.0670814925009));
#22823=CARTESIAN_POINT('Ctrl Pts',(-41.6880687186425,37.1701307676679,38.0719866834278));
#22824=CARTESIAN_POINT('Ctrl Pts',(-41.6909070883976,37.1745059552378,38.0768849447736));
#22825=CARTESIAN_POINT('Ctrl Pts',(-41.6937454581527,37.1788811428077,38.0817832061194));
#22826=CARTESIAN_POINT('Ctrl Pts',(-41.6965774340572,37.1832682305312,38.0866745378841));
#22827=CARTESIAN_POINT('Ctrl Pts',(-41.6994029908958,37.1876671792505,38.0915588964065));
#22828=CARTESIAN_POINT('Ctrl Pts',(-41.7022285477345,37.1920661279698,38.0964432549289));
#22829=CARTESIAN_POINT('Ctrl Pts',(-41.7050476855074,37.1964769376847,38.1013206402089));
#22830=CARTESIAN_POINT('Ctrl Pts',(-41.7078603791122,37.2008995690293,38.1061910087076));
#22831=CARTESIAN_POINT('Ctrl Pts',(-41.710673072717,37.2053222003739,38.1110613772063));
#22832=CARTESIAN_POINT('Ctrl Pts',(-41.7134793221537,37.209756653348,38.1159247289238));
#22833=CARTESIAN_POINT('Ctrl Pts',(-41.716279102433,37.2142028883784,38.1207810204443));
#22834=CARTESIAN_POINT('Ctrl Pts',(-41.7190788827123,37.2186491234088,38.1256373119647));
#22835=CARTESIAN_POINT('Ctrl Pts',(-41.7218721938341,37.2231071404953,38.1304865432881));
#22836=CARTESIAN_POINT('Ctrl Pts',(-41.7246590109227,37.227576899858,38.1353286711225));
#22837=CARTESIAN_POINT('Ctrl Pts',(-41.7274458280114,37.2320466592206,38.1401707989569));
#22838=CARTESIAN_POINT('Ctrl Pts',(-41.7302261510669,37.2365281608594,38.1450058233024));
#22839=CARTESIAN_POINT('Ctrl Pts',(-41.7329999553273,37.2410213647883,38.1498337009917));
#22840=CARTESIAN_POINT('Ctrl Pts',(-41.7357737595877,37.2455145687171,38.154661578681));
#22841=CARTESIAN_POINT('Ctrl Pts',(-41.7385410450531,37.2500194749359,38.1594823097141));
#22842=CARTESIAN_POINT('Ctrl Pts',(-41.7413017870759,37.2545360432535,38.1642958510492));
#22843=CARTESIAN_POINT('Ctrl Pts',(-41.5812887586841,37.0246695558006,37.9068043561179));
#22844=CARTESIAN_POINT('Ctrl Pts',(-41.5846313316133,37.029208650787,37.9123864232581));
#22845=CARTESIAN_POINT('Ctrl Pts',(-41.5879664082902,37.0337629504581,37.9179605923033));
#22846=CARTESIAN_POINT('Ctrl Pts',(-41.5912939522271,37.0383324046554,37.923526802022));
#22847=CARTESIAN_POINT('Ctrl Pts',(-41.5946185414596,37.0428978013895,37.9290880692049));
#22848=CARTESIAN_POINT('Ctrl Pts',(-41.5979356113237,37.0474783257485,37.93464139119));
#22849=CARTESIAN_POINT('Ctrl Pts',(-41.6012451255902,37.0520739273846,37.940186707079));
#22850=CARTESIAN_POINT('Ctrl Pts',(-41.6045546398567,37.0566695290208,37.945732022968));
#22851=CARTESIAN_POINT('Ctrl Pts',(-41.6078565985256,37.0612802079339,37.9512693327608));
#22852=CARTESIAN_POINT('Ctrl Pts',(-41.6111509655294,37.0659059134548,37.9567985757307));
#22853=CARTESIAN_POINT('Ctrl Pts',(-41.6144453325332,37.0705316189757,37.9623278187007));
#22854=CARTESIAN_POINT('Ctrl Pts',(-41.6177321078719,37.0751723511041,37.9678489948478));
#22855=CARTESIAN_POINT('Ctrl Pts',(-41.6210112556406,37.0798280588501,37.9733620436181));
#22856=CARTESIAN_POINT('Ctrl Pts',(-41.6242904034094,37.084483766596,37.9788750923885));
#22857=CARTESIAN_POINT('Ctrl Pts',(-41.6275619236081,37.0891544499595,37.9843800137821));
#22858=CARTESIAN_POINT('Ctrl Pts',(-41.6308257804953,37.0938400576309,37.9898767474193));
#22859=CARTESIAN_POINT('Ctrl Pts',(-41.6340896373825,37.0985256653023,37.9953734810565));
#22860=CARTESIAN_POINT('Ctrl Pts',(-41.6373458309581,37.1032261972816,38.0008620269372));
#22861=CARTESIAN_POINT('Ctrl Pts',(-41.6405943256446,37.1079416019407,38.0063423248572));
#22862=CARTESIAN_POINT('Ctrl Pts',(-41.6438428203311,37.1126570065999,38.0118226227772));
#22863=CARTESIAN_POINT('Ctrl Pts',(-41.6470836161284,37.1173872839388,38.0172946727364));
#22864=CARTESIAN_POINT('Ctrl Pts',(-41.6503166776239,37.1221323820122,38.0227584147072));
#22865=CARTESIAN_POINT('Ctrl Pts',(-41.6535497391193,37.1268774800855,38.0282221566779));
#22866=CARTESIAN_POINT('Ctrl Pts',(-41.6567750663129,37.1316373988932,38.0336775906601));
#22867=CARTESIAN_POINT('Ctrl Pts',(-41.6599926239573,37.1364120861736,38.0391246568041));
#22868=CARTESIAN_POINT('Ctrl Pts',(-41.6632101816016,37.141186773454,38.044571722948));
#22869=CARTESIAN_POINT('Ctrl Pts',(-41.6664199696968,37.1459762292069,38.0500104212536));
#22870=CARTESIAN_POINT('Ctrl Pts',(-41.6696219531617,37.1507804008554,38.0554406920501));
#22871=CARTESIAN_POINT('Ctrl Pts',(-41.6728239366267,37.155584572504,38.0608709628466));
#22872=CARTESIAN_POINT('Ctrl Pts',(-41.6760181154612,37.1604034600481,38.066292806134));
#22873=CARTESIAN_POINT('Ctrl Pts',(-41.6792044547515,37.1652370105968,38.0717061624219));
#22874=CARTESIAN_POINT('Ctrl Pts',(-41.6823907940418,37.1700705611453,38.0771195187099));
#22875=CARTESIAN_POINT('Ctrl Pts',(-41.6855692937877,37.1749187746984,38.0825243879982));
#22876=CARTESIAN_POINT('Ctrl Pts',(-41.6887399192427,37.1797815980517,38.0879207109784));
#22877=CARTESIAN_POINT('Ctrl Pts',(-41.6919105446977,37.184644421405,38.0933170339585));
#22878=CARTESIAN_POINT('Ctrl Pts',(-41.6950732958619,37.1895218545586,38.0987048106302));
#22879=CARTESIAN_POINT('Ctrl Pts',(-41.6982281381571,37.1944138439962,38.1040839818675));
#22880=CARTESIAN_POINT('Ctrl Pts',(-41.7013829804523,37.1993058334339,38.1094631531049));
#22881=CARTESIAN_POINT('Ctrl Pts',(-41.7045299138786,37.2042123791556,38.1148337189078));
#22882=CARTESIAN_POINT('Ctrl Pts',(-41.7076689040269,37.2091334273345,38.1201956203343));
#22883=CARTESIAN_POINT('Ctrl Pts',(-41.7108078941752,37.2140544755134,38.1255575217609));
#22884=CARTESIAN_POINT('Ctrl Pts',(-41.7139389410454,37.2189900261494,38.1309107588109));
#22885=CARTESIAN_POINT('Ctrl Pts',(-41.7170620103986,37.2239400251058,38.1362552727277));
#22886=CARTESIAN_POINT('Ctrl Pts',(-41.7201850797517,37.2288900240622,38.1415997866445));
#22887=CARTESIAN_POINT('Ctrl Pts',(-41.7233001715877,37.2338544713389,38.1469355774281));
#22888=CARTESIAN_POINT('Ctrl Pts',(-41.7264072518377,37.2388333124907,38.152262586508));
#22889=CARTESIAN_POINT('Ctrl Pts',(-41.7295143320877,37.2438121536425,38.157589595588));
#22890=CARTESIAN_POINT('Ctrl Pts',(-41.7326134007518,37.2488053886693,38.1629078229643));
#22891=CARTESIAN_POINT('Ctrl Pts',(-41.7357044239324,37.2538129628184,38.1682172102543));
#22892=CARTESIAN_POINT('Ctrl Pts',(-41.5583014337907,37.0028702244532,37.8858609795071));
#22893=CARTESIAN_POINT('Ctrl Pts',(-41.5620325071846,37.0077967995883,37.8919889217062));
#22894=CARTESIAN_POINT('Ctrl Pts',(-41.565754568211,37.012741966141,37.8981074045777));
#22895=CARTESIAN_POINT('Ctrl Pts',(-41.5694675661243,37.0177056566895,37.9042163447035));
#22896=CARTESIAN_POINT('Ctrl Pts',(-41.5731772670678,37.0226649397112,37.9103198603741));
#22897=CARTESIAN_POINT('Ctrl Pts',(-41.5768779209862,37.0276427138463,37.9164138502385));
#22898=CARTESIAN_POINT('Ctrl Pts',(-41.580569477515,37.0326389113493,37.9224982313596));
#22899=CARTESIAN_POINT('Ctrl Pts',(-41.5842610340438,37.0376351088523,37.9285826124808));
#22900=CARTESIAN_POINT('Ctrl Pts',(-41.5879434931829,37.042649729723,37.9346573848587));
#22901=CARTESIAN_POINT('Ctrl Pts',(-41.5916168048155,37.0476827057143,37.9407224658179));
#22902=CARTESIAN_POINT('Ctrl Pts',(-41.595290116448,37.0527156817056,37.9467875467772));
#22903=CARTESIAN_POINT('Ctrl Pts',(-41.5989542805739,37.0577670128175,37.9528429363176));
#22904=CARTESIAN_POINT('Ctrl Pts',(-41.6026092473254,37.0628366303032,37.9588885520279));
#22905=CARTESIAN_POINT('Ctrl Pts',(-41.6062642140768,37.067906247789,37.9649341677381));
#22906=CARTESIAN_POINT('Ctrl Pts',(-41.6099099834537,37.0729941516485,37.9709700096178));
#22907=CARTESIAN_POINT('Ctrl Pts',(-41.6135465058385,37.0781002726373,37.9769959955217));
#22908=CARTESIAN_POINT('Ctrl Pts',(-41.6171830282233,37.0832063936262,37.9830219814256));
#22909=CARTESIAN_POINT('Ctrl Pts',(-41.6208103036159,37.0883307317442,37.9890381113535));
#22910=CARTESIAN_POINT('Ctrl Pts',(-41.6244282826505,37.0934732172512,37.9950443034281));
#22911=CARTESIAN_POINT('Ctrl Pts',(-41.6280462616851,37.0986157027582,38.0010504955027));
#22912=CARTESIAN_POINT('Ctrl Pts',(-41.6316549443616,37.103776335654,38.0070467497239));
#22913=CARTESIAN_POINT('Ctrl Pts',(-41.6352542815672,37.1089550457045,38.013032984485));
#22914=CARTESIAN_POINT('Ctrl Pts',(-41.6388536187729,37.1141337557549,38.0190192192461));
#22915=CARTESIAN_POINT('Ctrl Pts',(-41.6424436105076,37.1193305429598,38.0249954345469));
#22916=CARTESIAN_POINT('Ctrl Pts',(-41.646024207913,37.1245453365929,38.0309615490536));
#22917=CARTESIAN_POINT('Ctrl Pts',(-41.6496048053184,37.129760130226,38.0369276635602));
#22918=CARTESIAN_POINT('Ctrl Pts',(-41.6531760083943,37.1349929302873,38.0428836772724));
#22919=CARTESIAN_POINT('Ctrl Pts',(-41.656737768538,37.1402436655602,38.0488295091312));
#22920=CARTESIAN_POINT('Ctrl Pts',(-41.6602995286818,37.1454944008331,38.0547753409901));
#22921=CARTESIAN_POINT('Ctrl Pts',(-41.6638518458934,37.1507630713176,38.0607109909953));
#22922=CARTESIAN_POINT('Ctrl Pts',(-41.6673946718271,37.1560496053091,38.0666363783651));
#22923=CARTESIAN_POINT('Ctrl Pts',(-41.6709374977608,37.1613361393005,38.0725617657349));
#22924=CARTESIAN_POINT('Ctrl Pts',(-41.6744708324165,37.1666405367989,38.0784768904691));
#22925=CARTESIAN_POINT('Ctrl Pts',(-41.6779946277069,37.1719627256134,38.084381672065));
#22926=CARTESIAN_POINT('Ctrl Pts',(-41.6815184229973,37.1772849144277,38.0902864536611));
#22927=CARTESIAN_POINT('Ctrl Pts',(-41.6850326789224,37.1826248945581,38.0961808921187));
#22928=CARTESIAN_POINT('Ctrl Pts',(-41.6885373476544,37.1879825933294,38.102064907217));
#22929=CARTESIAN_POINT('Ctrl Pts',(-41.6920420163864,37.1933402921006,38.1079489223154));
#22930=CARTESIAN_POINT('Ctrl Pts',(-41.6955370979252,37.1987157095126,38.1138225140541));
#22931=CARTESIAN_POINT('Ctrl Pts',(-41.6990225447042,37.2041087724079,38.1196856024962));
#22932=CARTESIAN_POINT('Ctrl Pts',(-41.7025079914833,37.2095018353033,38.1255486909382));
#22933=CARTESIAN_POINT('Ctrl Pts',(-41.7059838035024,37.2149125436819,38.1314012760832));
#22934=CARTESIAN_POINT('Ctrl Pts',(-41.7094499334571,37.2203408239061,38.1372432782799));
#22935=CARTESIAN_POINT('Ctrl Pts',(-41.7129160634118,37.2257691041303,38.1430852804766));
#22936=CARTESIAN_POINT('Ctrl Pts',(-41.7163725113021,37.2312149562,38.1489166997247));
#22937=CARTESIAN_POINT('Ctrl Pts',(-41.7198192300869,37.2366783059992,38.154737456661));
#22938=CARTESIAN_POINT('Ctrl Pts',(-41.7232659488718,37.2421416557985,38.1605582135972));
#22939=CARTESIAN_POINT('Ctrl Pts',(-41.7267029385512,37.2476225033271,38.1663683082215));
#22940=CARTESIAN_POINT('Ctrl Pts',(-41.730130152349,37.2531207739928,38.1721676614605));
#22941=CARTESIAN_POINT('Ctrl Pts',(-41.5353141088974,36.9810708931059,37.8649176028963));
#22942=CARTESIAN_POINT('Ctrl Pts',(-41.5394336827557,36.9863849483897,37.8715914201543));
#22943=CARTESIAN_POINT('Ctrl Pts',(-41.5435427281318,36.9917209818238,37.878254216852));
#22944=CARTESIAN_POINT('Ctrl Pts',(-41.5476411800214,36.9970789087236,37.884905887385));
#22945=CARTESIAN_POINT('Ctrl Pts',(-41.551735992676,37.002432078033,37.8915516515433));
#22946=CARTESIAN_POINT('Ctrl Pts',(-41.5558202306487,37.0078071019442,37.8981863092869));
#22947=CARTESIAN_POINT('Ctrl Pts',(-41.5598938294398,37.013203895314,37.9048097556403));
#22948=CARTESIAN_POINT('Ctrl Pts',(-41.5639674282308,37.0186006886838,37.9114332019936));
#22949=CARTESIAN_POINT('Ctrl Pts',(-41.5680303878402,37.0240192515119,37.9180454369566));
#22950=CARTESIAN_POINT('Ctrl Pts',(-41.5720826441015,37.0294594979738,37.9246463559051));
#22951=CARTESIAN_POINT('Ctrl Pts',(-41.5761349003628,37.0348997444356,37.9312472748536));
#22952=CARTESIAN_POINT('Ctrl Pts',(-41.580176453276,37.0403616745309,37.9378368777876));
#22953=CARTESIAN_POINT('Ctrl Pts',(-41.5842072390102,37.0458452017564,37.9444150604376));
#22954=CARTESIAN_POINT('Ctrl Pts',(-41.5882380247443,37.0513287289819,37.9509932430877));
#22955=CARTESIAN_POINT('Ctrl Pts',(-41.5922580432993,37.0568338533374,37.9575600054536));
#22956=CARTESIAN_POINT('Ctrl Pts',(-41.5962672311817,37.0623604876437,37.9641152436242));
#22957=CARTESIAN_POINT('Ctrl Pts',(-41.6002764190641,37.06788712195,37.9706704817948));
#22958=CARTESIAN_POINT('Ctrl Pts',(-41.6042747762737,37.0734352662068,37.9772141957697));
#22959=CARTESIAN_POINT('Ctrl Pts',(-41.6082622396564,37.0790048325617,37.9837462819989));
#22960=CARTESIAN_POINT('Ctrl Pts',(-41.6122497030391,37.0845743989165,37.9902783682281));
#22961=CARTESIAN_POINT('Ctrl Pts',(-41.6162262725948,37.0901653873693,37.9967988267113));
#22962=CARTESIAN_POINT('Ctrl Pts',(-41.6201918855106,37.0957777093968,38.0033075542628));
#22963=CARTESIAN_POINT('Ctrl Pts',(-41.6241574984265,37.1013900314243,38.0098162818142));
#22964=CARTESIAN_POINT('Ctrl Pts',(-41.6281121547024,37.1070236870264,38.0163132784337));
#22965=CARTESIAN_POINT('Ctrl Pts',(-41.6320557918687,37.1126785870122,38.0227984413031));
#22966=CARTESIAN_POINT('Ctrl Pts',(-41.6359994290351,37.1183334869982,38.0292836041724));
#22967=CARTESIAN_POINT('Ctrl Pts',(-41.6399320470917,37.1240096313677,38.0357569332913));
#22968=CARTESIAN_POINT('Ctrl Pts',(-41.6438535839144,37.1297069302649,38.0422183262124));
#22969=CARTESIAN_POINT('Ctrl Pts',(-41.647775120737,37.1354042291623,38.0486797191335));
#22970=CARTESIAN_POINT('Ctrl Pts',(-41.6516855763256,37.141122682587,38.0551291758567));
#22971=CARTESIAN_POINT('Ctrl Pts',(-41.6555848889026,37.1468622000214,38.0615665943083));
#22972=CARTESIAN_POINT('Ctrl Pts',(-41.6594842014798,37.1526017174557,38.06800401276));
#22973=CARTESIAN_POINT('Ctrl Pts',(-41.6633723710453,37.1583622988995,38.0744293929399));
#22974=CARTESIAN_POINT('Ctrl Pts',(-41.6672493361711,37.164143853175,38.0808426331518));
#22975=CARTESIAN_POINT('Ctrl Pts',(-41.6711263012969,37.1699254074505,38.0872558733636));
#22976=CARTESIAN_POINT('Ctrl Pts',(-41.6749920619829,37.1757279345577,38.0936569736073));
#22977=CARTESIAN_POINT('Ctrl Pts',(-41.6788465571516,37.1815513426625,38.1000458325666));
#22978=CARTESIAN_POINT('Ctrl Pts',(-41.6827010523204,37.1873747507672,38.1064346915258));
#22979=CARTESIAN_POINT('Ctrl Pts',(-41.6865442819719,37.1932190398695,38.1128113092005));
#22980=CARTESIAN_POINT('Ctrl Pts',(-41.6903761853817,37.1990841174813,38.119175584658));
#22981=CARTESIAN_POINT('Ctrl Pts',(-41.6942080887914,37.2049491950931,38.1255398601155));
#22982=CARTESIAN_POINT('Ctrl Pts',(-41.6980286659593,37.2108350612144,38.1318917933555));
#22983=CARTESIAN_POINT('Ctrl Pts',(-41.7018378565156,37.2167416227065,38.1382312838321));
#22984=CARTESIAN_POINT('Ctrl Pts',(-41.7056470470719,37.2226481841985,38.1445707743086));
#22985=CARTESIAN_POINT('Ctrl Pts',(-41.7094448510165,37.2285754410611,38.1508978220214));
#22986=CARTESIAN_POINT('Ctrl Pts',(-41.7132312083362,37.2345232995077,38.1572123268139));
#22987=CARTESIAN_POINT('Ctrl Pts',(-41.7170175656559,37.2404711579544,38.1635268316065));
#22988=CARTESIAN_POINT('Ctrl Pts',(-41.7207924763506,37.2464396179848,38.1698287934786));
#22989=CARTESIAN_POINT('Ctrl Pts',(-41.7245558807656,37.2524285851673,38.1761181126667));
#22990=CARTESIAN_POINT('Ctrl Pts',(-41.5119116205319,36.9596544812705,37.8441194560785));
#22991=CARTESIAN_POINT('Ctrl Pts',(-41.5164318225131,36.9653413393433,37.8513397802637));
#22992=CARTESIAN_POINT('Ctrl Pts',(-41.5209398144549,36.9710540452047,37.8585473625558));
#22993=CARTESIAN_POINT('Ctrl Pts',(-41.5254355129223,36.9767924926594,37.8657420692341));
#22994=CARTESIAN_POINT('Ctrl Pts',(-41.5299272194183,36.9825258446392,37.8729303873468));
#22995=CARTESIAN_POINT('Ctrl Pts',(-41.534406654262,36.9882848925176,37.8801058527013));
#22996=CARTESIAN_POINT('Ctrl Pts',(-41.5388737346897,36.9940695294441,37.8872683324032));
#22997=CARTESIAN_POINT('Ctrl Pts',(-41.5433408151174,36.9998541663706,37.8944308121051));
#22998=CARTESIAN_POINT('Ctrl Pts',(-41.5477955411289,37.0056643923449,37.9015803061543));
#22999=CARTESIAN_POINT('Ctrl Pts',(-41.5522378304123,37.0115000995826,37.908716682132));
#23000=CARTESIAN_POINT('Ctrl Pts',(-41.5566801196957,37.0173358068204,37.9158530581097));
#23001=CARTESIAN_POINT('Ctrl Pts',(-41.561109972251,37.0231969953212,37.9229763160157));
#23002=CARTESIAN_POINT('Ctrl Pts',(-41.5655273062213,37.029083556371,37.9300863239114));
#23003=CARTESIAN_POINT('Ctrl Pts',(-41.5699446401916,37.0349701174208,37.9371963318071));
#23004=CARTESIAN_POINT('Ctrl Pts',(-41.5743494555768,37.0408820510191,37.9442930896923));
#23005=CARTESIAN_POINT('Ctrl Pts',(-41.5787416709781,37.0468192475256,37.9513764661133));
#23006=CARTESIAN_POINT('Ctrl Pts',(-41.5831338863793,37.0527564440322,37.9584598425344));
#23007=CARTESIAN_POINT('Ctrl Pts',(-41.5875135017965,37.0587189034466,37.965529837491));
#23008=CARTESIAN_POINT('Ctrl Pts',(-41.5918804362916,37.0647065152065,37.9725863200193));
#23009=CARTESIAN_POINT('Ctrl Pts',(-41.5962473707868,37.0706941269664,37.9796428025476));
#23010=CARTESIAN_POINT('Ctrl Pts',(-41.6006016243598,37.0767068910715,37.9866857726473));
#23011=CARTESIAN_POINT('Ctrl Pts',(-41.6049431165364,37.082744696041,37.9937150998487));
#23012=CARTESIAN_POINT('Ctrl Pts',(-41.609284608713,37.0887825010107,38.0007444270501));
#23013=CARTESIAN_POINT('Ctrl Pts',(-41.6136133394932,37.0948453468446,38.007760111353));
#23014=CARTESIAN_POINT('Ctrl Pts',(-41.6179292288694,37.1009331211479,38.0147620227869));
#23015=CARTESIAN_POINT('Ctrl Pts',(-41.6222451182455,37.1070208954514,38.0217639342208));
#23016=CARTESIAN_POINT('Ctrl Pts',(-41.6265481662175,37.1131335982241,38.0287520727853));
#23017=CARTESIAN_POINT('Ctrl Pts',(-41.6308382932475,37.1192711161612,38.0357263090137));
#23018=CARTESIAN_POINT('Ctrl Pts',(-41.6351284202774,37.1254086340983,38.042700545242));
#23019=CARTESIAN_POINT('Ctrl Pts',(-41.639405626365,37.1315709671997,38.0496608791339));
#23020=CARTESIAN_POINT('Ctrl Pts',(-41.6436698324448,37.1377580012544,38.0566071817309));
#23021=CARTESIAN_POINT('Ctrl Pts',(-41.6479340385245,37.1439450353091,38.0635534843278));
#23022=CARTESIAN_POINT('Ctrl Pts',(-41.6521852445963,37.1501567703169,38.0704857556296));
#23023=CARTESIAN_POINT('Ctrl Pts',(-41.6564233720695,37.1563930911652,38.0774038671906));
#23024=CARTESIAN_POINT('Ctrl Pts',(-41.6606614995428,37.1626294120135,38.0843219787517));
#23025=CARTESIAN_POINT('Ctrl Pts',(-41.6648865484175,37.1688903187019,38.0912259305717));
#23026=CARTESIAN_POINT('Ctrl Pts',(-41.6690984405812,37.17517569522,38.0981155947229));
#23027=CARTESIAN_POINT('Ctrl Pts',(-41.673310332745,37.1814610717381,38.1050052588741));
#23028=CARTESIAN_POINT('Ctrl Pts',(-41.6775090681976,37.1877709180856,38.1118806353562));
#23029=CARTESIAN_POINT('Ctrl Pts',(-41.6816945693075,37.1941051173586,38.1187415967635));
#23030=CARTESIAN_POINT('Ctrl Pts',(-41.6858800704174,37.2004393166314,38.1256025581708));
#23031=CARTESIAN_POINT('Ctrl Pts',(-41.6900523371845,37.2067978688295,38.132449104503));
#23032=CARTESIAN_POINT('Ctrl Pts',(-41.6942112924608,37.2131806561592,38.1392811088814));
#23033=CARTESIAN_POINT('Ctrl Pts',(-41.6983702477371,37.2195634434889,38.1461131132597));
#23034=CARTESIAN_POINT('Ctrl Pts',(-41.7025158915224,37.22597046595,38.1529305756838));
#23035=CARTESIAN_POINT('Ctrl Pts',(-41.7066481471553,37.2324016048639,38.1597333698063));
#23036=CARTESIAN_POINT('Ctrl Pts',(-41.7107804027881,37.2388327437779,38.1665361639287));
#23037=CARTESIAN_POINT('Ctrl Pts',(-41.7148992702682,37.2452879991444,38.1733242897491));
#23038=CARTESIAN_POINT('Ctrl Pts',(-41.7190046734231,37.2517672514041,38.1800976214559));
#23039=CARTESIAN_POINT('Ctrl Pts',(-41.4883731457974,36.9388425395209,37.8236917716039));
#23040=CARTESIAN_POINT('Ctrl Pts',(-41.4932995733036,36.944883604912,37.8314537588732));
#23041=CARTESIAN_POINT('Ctrl Pts',(-41.4982119888981,36.950954823534,37.8392011713985));
#23042=CARTESIAN_POINT('Ctrl Pts',(-41.5031102855784,36.9570560631423,37.8469338404252));
#23043=CARTESIAN_POINT('Ctrl Pts',(-41.5080042327986,36.9631518851332,37.8546596432006));
#23044=CARTESIAN_POINT('Ctrl Pts',(-41.5128840861671,36.9692776748191,37.8623707286484));
#23045=CARTESIAN_POINT('Ctrl Pts',(-41.5177497395788,36.9754332990042,37.8700669291027));
#23046=CARTESIAN_POINT('Ctrl Pts',(-41.5226153929905,36.9815889231893,37.877763129557));
#23047=CARTESIAN_POINT('Ctrl Pts',(-41.5274668464452,36.9877743818732,37.8854444450174));
#23048=CARTESIAN_POINT('Ctrl Pts',(-41.5323039944555,36.9939895405628,37.8931107084654));
#23049=CARTESIAN_POINT('Ctrl Pts',(-41.5371411424658,37.0002046992523,37.9007769719134));
#23050=CARTESIAN_POINT('Ctrl Pts',(-41.5419639850314,37.0064495579469,37.9084281833486));
#23051=CARTESIAN_POINT('Ctrl Pts',(-41.546772417287,37.0127239808619,37.9160641764072));
#23052=CARTESIAN_POINT('Ctrl Pts',(-41.5515808495426,37.0189984037769,37.9237001694659));
#23053=CARTESIAN_POINT('Ctrl Pts',(-41.5563748714879,37.0253023909118,37.9313209441474));
#23054=CARTESIAN_POINT('Ctrl Pts',(-41.5611543788843,37.0316358051961,37.9389263347498));
#23055=CARTESIAN_POINT('Ctrl Pts',(-41.5659338862806,37.0379692194805,37.9465317253522));
#23056=CARTESIAN_POINT('Ctrl Pts',(-41.5706988791277,37.0443320609139,37.954121731875));
#23057=CARTESIAN_POINT('Ctrl Pts',(-41.5754492538182,37.050724191146,37.9616961892852));
#23058=CARTESIAN_POINT('Ctrl Pts',(-41.5801996285086,37.0571163213783,37.9692706466953));
#23059=CARTESIAN_POINT('Ctrl Pts',(-41.5849353850422,37.0635377404088,37.9768295549925));
#23060=CARTESIAN_POINT('Ctrl Pts',(-41.5896564204469,37.0699883086141,37.9843727498196));
#23061=CARTESIAN_POINT('Ctrl Pts',(-41.5943774558517,37.0764388768193,37.9919159446468));
#23062=CARTESIAN_POINT('Ctrl Pts',(-41.5990837701275,37.0829185941986,37.9994434260036));
#23063=CARTESIAN_POINT('Ctrl Pts',(-41.6037752609427,37.0894273198606,38.0069550302165));
#23064=CARTESIAN_POINT('Ctrl Pts',(-41.6084667517579,37.0959360455226,38.0144666344295));
#23065=CARTESIAN_POINT('Ctrl Pts',(-41.6131434191123,37.1024737794668,38.021962361498));
#23066=CARTESIAN_POINT('Ctrl Pts',(-41.6178051613189,37.1090403795404,38.0294420484391));
#23067=CARTESIAN_POINT('Ctrl Pts',(-41.6224669035254,37.115606979614,38.0369217353803));
#23068=CARTESIAN_POINT('Ctrl Pts',(-41.6271137205839,37.1222024458164,38.0443853821936));
#23069=CARTESIAN_POINT('Ctrl Pts',(-41.6317455114564,37.1288266347395,38.0518328265934));
#23070=CARTESIAN_POINT('Ctrl Pts',(-41.6363773023289,37.1354508236625,38.0592802709933));
#23071=CARTESIAN_POINT('Ctrl Pts',(-41.6409940670151,37.1421037353058,38.0667115129793));
#23072=CARTESIAN_POINT('Ctrl Pts',(-41.6455957051307,37.1487852250119,38.0741263909705));
#23073=CARTESIAN_POINT('Ctrl Pts',(-41.6501973432462,37.155466714718,38.0815412689617));
#23074=CARTESIAN_POINT('Ctrl Pts',(-41.6547838547908,37.1621767824866,38.0889397829577));
#23075=CARTESIAN_POINT('Ctrl Pts',(-41.6593551400376,37.1689152824175,38.0963217720891));
#23076=CARTESIAN_POINT('Ctrl Pts',(-41.6639264252845,37.1756537823485,38.1037037612205));
#23077=CARTESIAN_POINT('Ctrl Pts',(-41.6684824842335,37.1824207144413,38.1110692254869));
#23078=CARTESIAN_POINT('Ctrl Pts',(-41.6730232178201,37.1892159315596,38.1184180047376));
#23079=CARTESIAN_POINT('Ctrl Pts',(-41.6775639514066,37.1960111486779,38.1257667839883));
#23080=CARTESIAN_POINT('Ctrl Pts',(-41.6820893596305,37.2028346508212,38.1330988782228));
#23081=CARTESIAN_POINT('Ctrl Pts',(-41.6865993440937,37.2096862896228,38.140414128016));
#23082=CARTESIAN_POINT('Ctrl Pts',(-41.6911093285568,37.2165379284245,38.1477293778093));
#23083=CARTESIAN_POINT('Ctrl Pts',(-41.6956038892589,37.2234177038842,38.1550277831608));
#23084=CARTESIAN_POINT('Ctrl Pts',(-41.7000829284727,37.2303254664117,38.162309185378));
#23085=CARTESIAN_POINT('Ctrl Pts',(-41.7045619676864,37.2372332289392,38.1695905875952));
#23086=CARTESIAN_POINT('Ctrl Pts',(-41.7090254854116,37.2441689785342,38.1768549866776));
#23087=CARTESIAN_POINT('Ctrl Pts',(-41.7134733845959,37.2511325643894,38.184102224672));
#23088=CARTESIAN_POINT('Ctrl Pts',(-41.4648346710629,36.9180305977713,37.8032640871294));
#23089=CARTESIAN_POINT('Ctrl Pts',(-41.4701673240942,36.9244258704808,37.8115677374827));
#23090=CARTESIAN_POINT('Ctrl Pts',(-41.4754841633414,36.9308556018634,37.8198549802413));
#23091=CARTESIAN_POINT('Ctrl Pts',(-41.4807850582345,36.9373196336253,37.8281256116162));
#23092=CARTESIAN_POINT('Ctrl Pts',(-41.486081246179,36.9437779256271,37.8363888990545));
#23093=CARTESIAN_POINT('Ctrl Pts',(-41.4913615180722,36.9502704571205,37.8446356045956));
#23094=CARTESIAN_POINT('Ctrl Pts',(-41.4966257444679,36.9567970685643,37.8528655258022));
#23095=CARTESIAN_POINT('Ctrl Pts',(-41.5018899708636,36.963323680008,37.8610954470088));
#23096=CARTESIAN_POINT('Ctrl Pts',(-41.5071381517616,36.9698843714016,37.8693085838804));
#23097=CARTESIAN_POINT('Ctrl Pts',(-41.5123701584987,36.9764789815429,37.8775047347988));
#23098=CARTESIAN_POINT('Ctrl Pts',(-41.5176021652359,36.9830735916842,37.8857008857171));
#23099=CARTESIAN_POINT('Ctrl Pts',(-41.5228179978118,36.9897021205725,37.8938800506816));
#23100=CARTESIAN_POINT('Ctrl Pts',(-41.5280175283527,36.9963644053527,37.9020420289031));
#23101=CARTESIAN_POINT('Ctrl Pts',(-41.5332170588936,37.003026690133,37.9102040071246));
#23102=CARTESIAN_POINT('Ctrl Pts',(-41.538400287399,37.0097227308045,37.9183487986025));
#23103=CARTESIAN_POINT('Ctrl Pts',(-41.5435670867904,37.0164523628666,37.9264762033862));
#23104=CARTESIAN_POINT('Ctrl Pts',(-41.5487338861819,37.0231819949288,37.93460360817));
#23105=CARTESIAN_POINT('Ctrl Pts',(-41.553884256459,37.029945218381,37.9427136262589));
#23106=CARTESIAN_POINT('Ctrl Pts',(-41.5590180713448,37.0367418670856,37.950806058551));
#23107=CARTESIAN_POINT('Ctrl Pts',(-41.5641518862305,37.0435385157901,37.9588984908431));
#23108=CARTESIAN_POINT('Ctrl Pts',(-41.5692691457245,37.0503685897463,37.9669733373377));
#23109=CARTESIAN_POINT('Ctrl Pts',(-41.5743697243575,37.0572319211871,37.9750303997906));
#23110=CARTESIAN_POINT('Ctrl Pts',(-41.5794703029904,37.0640952526279,37.9830874622435));
#23111=CARTESIAN_POINT('Ctrl Pts',(-41.5845542007618,37.0709918415526,37.9911267406543));
#23112=CARTESIAN_POINT('Ctrl Pts',(-41.5896212930161,37.0779215185733,37.9991480376462));
#23113=CARTESIAN_POINT('Ctrl Pts',(-41.5946883852703,37.0848511955938,38.0071693346381));
#23114=CARTESIAN_POINT('Ctrl Pts',(-41.599738672007,37.0918139607097,38.0151726502107));
#23115=CARTESIAN_POINT('Ctrl Pts',(-41.6047720293902,37.0988096429197,38.0231577878646));
#23116=CARTESIAN_POINT('Ctrl Pts',(-41.6098053867735,37.1058053251296,38.0311429255186));
#23117=CARTESIAN_POINT('Ctrl Pts',(-41.6148218148028,37.1128339244332,38.0391098852532));
#23118=CARTESIAN_POINT('Ctrl Pts',(-41.619821190468,37.1198952682246,38.047058471456));
#23119=CARTESIAN_POINT('Ctrl Pts',(-41.6248205661333,37.1269566120159,38.0550070576587));
#23120=CARTESIAN_POINT('Ctrl Pts',(-41.629802889434,37.1340507002946,38.062937270329));
#23121=CARTESIAN_POINT('Ctrl Pts',(-41.6347680381918,37.1411773588585,38.0708489147504));
#23122=CARTESIAN_POINT('Ctrl Pts',(-41.6397331869496,37.1483040174226,38.0787605591718));
#23123=CARTESIAN_POINT('Ctrl Pts',(-41.644681161164,37.1554632462713,38.0866536353436));
#23124=CARTESIAN_POINT('Ctrl Pts',(-41.649611839494,37.1626548696151,38.0945279494552));
#23125=CARTESIAN_POINT('Ctrl Pts',(-41.6545425178241,37.1698464929588,38.1024022635669));
#23126=CARTESIAN_POINT('Ctrl Pts',(-41.6594559002695,37.177070510797,38.1102578156176));
#23127=CARTESIAN_POINT('Ctrl Pts',(-41.6643518663326,37.1843267457607,38.1180944127116));
#23128=CARTESIAN_POINT('Ctrl Pts',(-41.6692478323959,37.1915829807243,38.1259310098057));
#23129=CARTESIAN_POINT('Ctrl Pts',(-41.6741263820765,37.1988714328129,38.1337486519425));
#23130=CARTESIAN_POINT('Ctrl Pts',(-41.6789873957265,37.2061919230865,38.1415471471507));
#23131=CARTESIAN_POINT('Ctrl Pts',(-41.6838484093764,37.2135124133602,38.1493456423588));
#23132=CARTESIAN_POINT('Ctrl Pts',(-41.6886918869953,37.2208649418183,38.1571249906378));
#23133=CARTESIAN_POINT('Ctrl Pts',(-41.69351770979,37.2282493279595,38.1648850009497));
#23134=CARTESIAN_POINT('Ctrl Pts',(-41.6983435325848,37.2356337141006,38.1726450112617));
#23135=CARTESIAN_POINT('Ctrl Pts',(-41.703151700555,37.243049957924,38.180385683606));
#23136=CARTESIAN_POINT('Ctrl Pts',(-41.7079420957686,37.2504978773748,38.1881068278881));
#23137=CARTESIAN_POINT('Ctrl Pts',(-41.4411625260449,36.8978229684399,37.7832073884005));
#23138=CARTESIAN_POINT('Ctrl Pts',(-41.4469069412086,36.9045538788403,37.7920478342999));
#23139=CARTESIAN_POINT('Ctrl Pts',(-41.4526336212004,36.9113239876996,37.8008699290073));
#23140=CARTESIAN_POINT('Ctrl Pts',(-41.4583424066575,36.9181331060726,37.8096734267128));
#23141=CARTESIAN_POINT('Ctrl Pts',(-41.464046122978,36.9249361782645,37.8184691073211));
#23142=CARTESIAN_POINT('Ctrl Pts',(-41.4697319765726,36.9317781907605,37.8272462239758));
#23143=CARTESIAN_POINT('Ctrl Pts',(-41.4753998095769,36.9386589530465,37.8360045326208));
#23144=CARTESIAN_POINT('Ctrl Pts',(-41.4810676425811,36.9455397153324,37.8447628412659));
#23145=CARTESIAN_POINT('Ctrl Pts',(-41.4867174549946,36.9524592274075,37.8535023419004));
#23146=CARTESIAN_POINT('Ctrl Pts',(-41.4923490899483,36.9594172966217,37.8622227915074));
#23147=CARTESIAN_POINT('Ctrl Pts',(-41.4979807249019,36.9663753658359,37.8709432411143));
#23148=CARTESIAN_POINT('Ctrl Pts',(-41.5035941823952,36.9733719921884,37.8796446396928));
#23149=CARTESIAN_POINT('Ctrl Pts',(-41.5091893065629,36.9804069809039,37.8883267452782));
#23150=CARTESIAN_POINT('Ctrl Pts',(-41.5147844307306,36.9874419696193,37.8970088508636));
#23151=CARTESIAN_POINT('Ctrl Pts',(-41.5203612215722,36.9945153206969,37.905671663455));
#23152=CARTESIAN_POINT('Ctrl Pts',(-41.5259195242348,37.0016268372465,37.9143149421534));
#23153=CARTESIAN_POINT('Ctrl Pts',(-41.5314778268974,37.0087383537961,37.9229582208518));
#23154=CARTESIAN_POINT('Ctrl Pts',(-41.5370176413805,37.0158880358169,37.9315819656562));
#23155=CARTESIAN_POINT('Ctrl Pts',(-41.542538813852,37.0230756843147,37.9401859367464));
#23156=CARTESIAN_POINT('Ctrl Pts',(-41.5480599863234,37.0302633328126,37.9487899078366));
#23157=CARTESIAN_POINT('Ctrl Pts',(-41.5535625167827,37.0374889477867,37.9573741052116));
#23158=CARTESIAN_POINT('Ctrl Pts',(-41.5590462524268,37.0447523281498,37.9659382901431));
#23159=CARTESIAN_POINT('Ctrl Pts',(-41.5645299880708,37.052015708513,37.9745024750745));
#23160=CARTESIAN_POINT('Ctrl Pts',(-41.5699949288992,37.0593168542644,37.9830466475614));
#23161=CARTESIAN_POINT('Ctrl Pts',(-41.5754409231463,37.0666555622348,37.9915705699802));
#23162=CARTESIAN_POINT('Ctrl Pts',(-41.5808869173934,37.0739942702052,38.000094492399));
#23163=CARTESIAN_POINT('Ctrl Pts',(-41.5863139650587,37.0813705403938,38.0085981647488));
#23164=CARTESIAN_POINT('Ctrl Pts',(-41.5917219154225,37.0887841675603,38.017081350524));
#23165=CARTESIAN_POINT('Ctrl Pts',(-41.5971298657864,37.0961977947268,38.0255645362992));
#23166=CARTESIAN_POINT('Ctrl Pts',(-41.6025187188481,37.1036487788704,38.0340272354987));
#23167=CARTESIAN_POINT('Ctrl Pts',(-41.607888324942,37.111136912691,38.0424692127479));
#23168=CARTESIAN_POINT('Ctrl Pts',(-41.613257931036,37.1186250465116,38.050911189997));
#23169=CARTESIAN_POINT('Ctrl Pts',(-41.6186082901615,37.1261503300086,38.0593324452947));
#23170=CARTESIAN_POINT('Ctrl Pts',(-41.623939253715,37.1337125538333,38.0677327444099));
#23171=CARTESIAN_POINT('Ctrl Pts',(-41.6292702172685,37.1412747776581,38.0761330435249));
#23172=CARTESIAN_POINT('Ctrl Pts',(-41.6345817852494,37.1488739418099,38.0845123864566));
#23173=CARTESIAN_POINT('Ctrl Pts',(-41.6398738101244,37.1565098349032,38.09287054013));
#23174=CARTESIAN_POINT('Ctrl Pts',(-41.6451658349994,37.1641457279966,38.1012286938033));
#23175=CARTESIAN_POINT('Ctrl Pts',(-41.6504383167679,37.1718183500307,38.1095656582175));
#23176=CARTESIAN_POINT('Ctrl Pts',(-41.6556911089748,37.1795274875948,38.1178812014669));
#23177=CARTESIAN_POINT('Ctrl Pts',(-41.6609439011816,37.1872366251589,38.1261967447164));
#23178=CARTESIAN_POINT('Ctrl Pts',(-41.6661770038263,37.1949822782522,38.1344908668002));
#23179=CARTESIAN_POINT('Ctrl Pts',(-41.6713902715401,37.2027642314499,38.1427633369947));
#23180=CARTESIAN_POINT('Ctrl Pts',(-41.6766035392538,37.2105461846477,38.1510358071891));
#23181=CARTESIAN_POINT('Ctrl Pts',(-41.6817969720361,37.2183644379491,38.1592866254934));
#23182=CARTESIAN_POINT('Ctrl Pts',(-41.6869704256122,37.2262187739276,38.1675155623782));
#23183=CARTESIAN_POINT('Ctrl Pts',(-41.6921438791884,37.2340731099062,38.175744499263));
#23184=CARTESIAN_POINT('Ctrl Pts',(-41.6972973535554,37.241963528558,38.1839515547247));
#23185=CARTESIAN_POINT('Ctrl Pts',(-41.7024307055465,37.2498898104733,38.1921365004474));
#23186=CARTESIAN_POINT('Ctrl Pts',(-41.4175681781877,36.8783311375915,37.7636543125594));
#23187=CARTESIAN_POINT('Ctrl Pts',(-41.4237247372187,36.8853777678676,37.7730231199949));
#23188=CARTESIAN_POINT('Ctrl Pts',(-41.4298615655738,36.8924687040171,37.7823715691034));
#23189=CARTESIAN_POINT('Ctrl Pts',(-41.4359784694956,36.8996037221832,37.7916993647842));
#23190=CARTESIAN_POINT('Ctrl Pts',(-41.4420899418905,36.9067324047845,37.8010188778155));
#23191=CARTESIAN_POINT('Ctrl Pts',(-41.448181525261,36.913905091185,37.8103177741145));
#23192=CARTESIAN_POINT('Ctrl Pts',(-41.4542530277002,36.9211215554196,37.8195957607326));
#23193=CARTESIAN_POINT('Ctrl Pts',(-41.4603245301395,36.9283380196542,37.8288737473507));
#23194=CARTESIAN_POINT('Ctrl Pts',(-41.4663759516467,36.9355982617217,37.8381308242868));
#23195=CARTESIAN_POINT('Ctrl Pts',(-41.4724071015805,36.9429020528988,37.8473666999098));
#23196=CARTESIAN_POINT('Ctrl Pts',(-41.4784382515143,36.9502058440759,37.8566025755327));
#23197=CARTESIAN_POINT('Ctrl Pts',(-41.4844491298738,36.9575531843614,37.8658172498414));
#23198=CARTESIAN_POINT('Ctrl Pts',(-41.4904395472949,36.9649438422879,37.8750104325405));
#23199=CARTESIAN_POINT('Ctrl Pts',(-41.496429964716,36.9723345002145,37.8842036152396));
#23200=CARTESIAN_POINT('Ctrl Pts',(-41.5023999211979,36.9797684757809,37.8933753063279));
#23201=CARTESIAN_POINT('Ctrl Pts',(-41.5083492286656,36.9872455347906,37.9025252168644));
#23202=CARTESIAN_POINT('Ctrl Pts',(-41.5142985361333,36.9947225938003,37.9116751274009));
#23203=CARTESIAN_POINT('Ctrl Pts',(-41.520227194586,37.0022427362521,37.9208032573843));
#23204=CARTESIAN_POINT('Ctrl Pts',(-41.5261350172497,37.0098057252348,37.9299093192459));
#23205=CARTESIAN_POINT('Ctrl Pts',(-41.5320428399134,37.0173687142174,37.9390153811075));
#23206=CARTESIAN_POINT('Ctrl Pts',(-41.5379298267874,37.0249745497298,37.9480993748461));
#23207=CARTESIAN_POINT('Ctrl Pts',(-41.5437957924105,37.0326229921609,37.9571610142833));
#23208=CARTESIAN_POINT('Ctrl Pts',(-41.5496617580337,37.0402714345921,37.9662226537206));
#23209=CARTESIAN_POINT('Ctrl Pts',(-41.5555067024051,37.0479624839409,37.9752619388553));
#23210=CARTESIAN_POINT('Ctrl Pts',(-41.5613304413883,37.055695897912,37.9842785849177));
#23211=CARTESIAN_POINT('Ctrl Pts',(-41.5671541803714,37.063429311883,37.99329523098));
#23212=CARTESIAN_POINT('Ctrl Pts',(-41.5729567139654,37.0712050904752,38.0022892379688));
#23213=CARTESIAN_POINT('Ctrl Pts',(-41.5787378593698,37.0790229887236,38.0112603225407));
#23214=CARTESIAN_POINT('Ctrl Pts',(-41.5845190047742,37.086840886972,38.0202314071125));
#23215=CARTESIAN_POINT('Ctrl Pts',(-41.5902787619881,37.0947009048757,38.0291795692662));
#23216=CARTESIAN_POINT('Ctrl Pts',(-41.5960169495586,37.102602794816,38.0381045271027));
#23217=CARTESIAN_POINT('Ctrl Pts',(-41.6017551371292,37.1105046847562,38.0470294849391));
#23218=CARTESIAN_POINT('Ctrl Pts',(-41.6074717550556,37.1184484467319,38.0559312384571));
#23219=CARTESIAN_POINT('Ctrl Pts',(-41.6131666232439,37.1264338304863,38.0648095072195));
#23220=CARTESIAN_POINT('Ctrl Pts',(-41.6188614914322,37.1344192142406,38.073687775982));
#23221=CARTESIAN_POINT('Ctrl Pts',(-41.6245346098817,37.1424462197725,38.0825425599877));
#23222=CARTESIAN_POINT('Ctrl Pts',(-41.6301857998689,37.1505145942025,38.0913735802794));
#23223=CARTESIAN_POINT('Ctrl Pts',(-41.635836989856,37.1585829686325,38.100204600571));
#23224=CARTESIAN_POINT('Ctrl Pts',(-41.64146625138,37.1666927119596,38.1090118571474));
#23225=CARTESIAN_POINT('Ctrl Pts',(-41.6470734070991,37.1748435686977,38.1177950725484));
#23226=CARTESIAN_POINT('Ctrl Pts',(-41.6526805628181,37.1829944254359,38.1265782879495));
#23227=CARTESIAN_POINT('Ctrl Pts',(-41.6582656127314,37.1911863955842,38.1353374621739));
#23228=CARTESIAN_POINT('Ctrl Pts',(-41.66382838089,37.1994192210661,38.1440723192766));
#23229=CARTESIAN_POINT('Ctrl Pts',(-41.6693911490485,37.207652046548,38.1528071763792));
#23230=CARTESIAN_POINT('Ctrl Pts',(-41.6749316354515,37.2159257273625,38.1615177163588));
#23231=CARTESIAN_POINT('Ctrl Pts',(-41.6804496655538,37.2242400028591,38.1702036648023));
#23232=CARTESIAN_POINT('Ctrl Pts',(-41.6859676956561,37.2325542783556,38.1788896132457));
#23233=CARTESIAN_POINT('Ctrl Pts',(-41.6914632694547,37.2409091485302,38.1875509701493));
#23234=CARTESIAN_POINT('Ctrl Pts',(-41.6969362138248,37.2493043501811,38.1961874626549));
#23235=CARTESIAN_POINT('Ctrl Pts',(-41.3939738303305,36.8588393067431,37.7441012367184));
#23236=CARTESIAN_POINT('Ctrl Pts',(-41.4005425332289,36.8662016568948,37.7539984056898));
#23237=CARTESIAN_POINT('Ctrl Pts',(-41.4070895099472,36.8736134203346,37.7638732091995));
#23238=CARTESIAN_POINT('Ctrl Pts',(-41.4136145323336,36.8810743382939,37.7737253028556));
#23239=CARTESIAN_POINT('Ctrl Pts',(-41.4201337608031,36.8885286313044,37.78356864831));
#23240=CARTESIAN_POINT('Ctrl Pts',(-41.4266310739494,36.8960319916095,37.7933893242532));
#23241=CARTESIAN_POINT('Ctrl Pts',(-41.4331062458236,36.9035841577927,37.8031869888444));
#23242=CARTESIAN_POINT('Ctrl Pts',(-41.4395814176978,36.9111363239759,37.8129846534356));
#23243=CARTESIAN_POINT('Ctrl Pts',(-41.4460344482988,36.918737296036,37.8227593066733));
#23244=CARTESIAN_POINT('Ctrl Pts',(-41.4524651132127,36.926386809176,37.8325106083122));
#23245=CARTESIAN_POINT('Ctrl Pts',(-41.4588957781266,36.9340363223159,37.8422619099512));
#23246=CARTESIAN_POINT('Ctrl Pts',(-41.4653040773524,36.9417343765344,37.85198985999));
#23247=CARTESIAN_POINT('Ctrl Pts',(-41.4716897880269,36.949480703672,37.8616941198028));
#23248=CARTESIAN_POINT('Ctrl Pts',(-41.4780754987014,36.9572270308095,37.8713983796156));
#23249=CARTESIAN_POINT('Ctrl Pts',(-41.4844386208236,36.9650216308649,37.8810789492008));
#23250=CARTESIAN_POINT('Ctrl Pts',(-41.4907789330963,36.9728642323347,37.8907354915754));
#23251=CARTESIAN_POINT('Ctrl Pts',(-41.4971192453691,36.9807068338045,37.90039203395));
#23252=CARTESIAN_POINT('Ctrl Pts',(-41.5034367477914,36.9885974366874,37.9100245491124));
#23253=CARTESIAN_POINT('Ctrl Pts',(-41.5097312206474,36.9965357661548,37.9196327017454));
#23254=CARTESIAN_POINT('Ctrl Pts',(-41.5160256935034,37.0044740956222,37.9292408543784));
#23255=CARTESIAN_POINT('Ctrl Pts',(-41.5222971367922,37.0124601516729,37.9388246444805));
#23256=CARTESIAN_POINT('Ctrl Pts',(-41.5285453323944,37.020493656172,37.9483837384236));
#23257=CARTESIAN_POINT('Ctrl Pts',(-41.5347935279965,37.0285271606712,37.9579428323667));
#23258=CARTESIAN_POINT('Ctrl Pts',(-41.5410184759111,37.0366081136174,37.9674772301492));
#23259=CARTESIAN_POINT('Ctrl Pts',(-41.5472199596302,37.0447362335891,37.9769865998551));
#23260=CARTESIAN_POINT('Ctrl Pts',(-41.5534214433494,37.0528643535608,37.986495969561));
#23261=CARTESIAN_POINT('Ctrl Pts',(-41.5595994628721,37.0610396405565,37.9959803111888));
#23262=CARTESIAN_POINT('Ctrl Pts',(-41.565753803317,37.0692618098869,38.0054392945573));
#23263=CARTESIAN_POINT('Ctrl Pts',(-41.5719081437619,37.0774839792173,38.0148982779259));
#23264=CARTESIAN_POINT('Ctrl Pts',(-41.5780388051281,37.0857530308811,38.0243319030337));
#23265=CARTESIAN_POINT('Ctrl Pts',(-41.5841455741753,37.0940686769409,38.0337398414575));
#23266=CARTESIAN_POINT('Ctrl Pts',(-41.5902523432224,37.1023843230008,38.0431477798813));
#23267=CARTESIAN_POINT('Ctrl Pts',(-41.5963352199497,37.1107465634554,38.0525300316195));
#23268=CARTESIAN_POINT('Ctrl Pts',(-41.6023939927728,37.1191551071392,38.0618862700293));
#23269=CARTESIAN_POINT('Ctrl Pts',(-41.608452765596,37.1275636508232,38.071242508439));
#23270=CARTESIAN_POINT('Ctrl Pts',(-41.614487434514,37.1360184977352,38.0805727335188));
#23271=CARTESIAN_POINT('Ctrl Pts',(-41.6204977896133,37.1445193535017,38.0898766204288));
#23272=CARTESIAN_POINT('Ctrl Pts',(-41.6265081447126,37.1530202092684,38.0991805073388));
#23273=CARTESIAN_POINT('Ctrl Pts',(-41.6324941859922,37.1615670738884,38.1084580560773));
#23274=CARTESIAN_POINT('Ctrl Pts',(-41.6384557052234,37.1701596498007,38.1177089436299));
#23275=CARTESIAN_POINT('Ctrl Pts',(-41.6444172244546,37.1787522257129,38.1269598311826));
#23276=CARTESIAN_POINT('Ctrl Pts',(-41.6503542216365,37.1873905129162,38.1361840575477));
#23277=CARTESIAN_POINT('Ctrl Pts',(-41.6562664902398,37.1960742106822,38.1453813015585));
#23278=CARTESIAN_POINT('Ctrl Pts',(-41.6621787588431,37.2047579084483,38.1545785455694));
#23279=CARTESIAN_POINT('Ctrl Pts',(-41.6680662988668,37.2134870167759,38.1637488072244));
#23280=CARTESIAN_POINT('Ctrl Pts',(-41.6739289054954,37.2222612317904,38.1728917672265));
#23281=CARTESIAN_POINT('Ctrl Pts',(-41.6797915121239,37.231035446805,38.1820347272285));
#23282=CARTESIAN_POINT('Ctrl Pts',(-41.6856291853541,37.2398547685024,38.1911503855738));
#23283=CARTESIAN_POINT('Ctrl Pts',(-41.6914417221031,37.2487188898889,38.2002384248625));
#23284=CARTESIAN_POINT('Ctrl Pts',(-41.3704568141619,36.8400609999701,37.7250501241905));
#23285=CARTESIAN_POINT('Ctrl Pts',(-41.3774380466235,36.8477192136434,37.7354672496683));
#23286=CARTESIAN_POINT('Ctrl Pts',(-41.3843954836192,36.8554323147081,37.7458599393064));
#23287=CARTESIAN_POINT('Ctrl Pts',(-41.3913288569572,36.8632000051908,37.7562277921192));
#23288=CARTESIAN_POINT('Ctrl Pts',(-41.3982560737816,36.8709607983251,37.7665864387599));
#23289=CARTESIAN_POINT('Ctrl Pts',(-41.4051592696763,36.8787760839841,37.7769202926724));
#23290=CARTESIAN_POINT('Ctrl Pts',(-41.4120381790331,36.8866455608354,37.7872289558619));
#23291=CARTESIAN_POINT('Ctrl Pts',(-41.4189170883898,36.8945150376866,37.7975376190515));
#23292=CARTESIAN_POINT('Ctrl Pts',(-41.4257717112071,36.9024387057288,37.8078210915159));
#23293=CARTESIAN_POINT('Ctrl Pts',(-41.4326017837395,36.9104162594787,37.8180789771934));
#23294=CARTESIAN_POINT('Ctrl Pts',(-41.4394318562719,36.9183938132286,37.8283368628709));
#23295=CARTESIAN_POINT('Ctrl Pts',(-41.4462373785179,36.9264252526848,37.8385691617593));
#23296=CARTESIAN_POINT('Ctrl Pts',(-41.453018088615,36.9345102682369,37.8487754797595));
#23297=CARTESIAN_POINT('Ctrl Pts',(-41.4597987987121,36.9425952837891,37.8589817977596));
#23298=CARTESIAN_POINT('Ctrl Pts',(-41.4665546966589,36.9507338754356,37.8691621348695));
#23299=CARTESIAN_POINT('Ctrl Pts',(-41.4732855224958,36.9589257294625,37.8793160989828));
#23300=CARTESIAN_POINT('Ctrl Pts',(-41.4800163483326,36.9671175834893,37.8894700630961));
#23301=CARTESIAN_POINT('Ctrl Pts',(-41.4867221020581,36.9753626998948,37.8995976542109));
#23302=CARTESIAN_POINT('Ctrl Pts',(-41.4934025256351,36.9836607608853,37.9096984822434));
#23303=CARTESIAN_POINT('Ctrl Pts',(-41.5000829492121,36.9919588218757,37.919799310276));
#23304=CARTESIAN_POINT('Ctrl Pts',(-41.5067380426394,37.0003098274494,37.9298733752245));
#23305=CARTESIAN_POINT('Ctrl Pts',(-41.5133675498222,37.0087134557569,37.9399202890576));
#23306=CARTESIAN_POINT('Ctrl Pts',(-41.5199970570049,37.0171170840643,37.9499672028907));
#23307=CARTESIAN_POINT('Ctrl Pts',(-41.5266009779418,37.025573335104,37.9599869656065));
#23308=CARTESIAN_POINT('Ctrl Pts',(-41.5331790584998,37.0340818829953,37.9699791912559));
#23309=CARTESIAN_POINT('Ctrl Pts',(-41.5397571390579,37.0425904308867,37.9799714169054));
#23310=CARTESIAN_POINT('Ctrl Pts',(-41.5463093792357,37.0511512756281,37.9899361054864));
#23311=CARTESIAN_POINT('Ctrl Pts',(-41.5528355268815,37.0597640873328,37.9998728731613));
#23312=CARTESIAN_POINT('Ctrl Pts',(-41.5593616745273,37.0683768990375,38.0098096408362));
#23313=CARTESIAN_POINT('Ctrl Pts',(-41.5658617296397,37.077041677704,38.0197184876031));
#23314=CARTESIAN_POINT('Ctrl Pts',(-41.5723354420671,37.0857580894643,38.0295990317648));
#23315=CARTESIAN_POINT('Ctrl Pts',(-41.5788091544946,37.0944745012246,38.0394795759265));
#23316=CARTESIAN_POINT('Ctrl Pts',(-41.5852565242357,37.1032425460772,38.0493318174811));
#23317=CARTESIAN_POINT('Ctrl Pts',(-41.5916773031583,37.1120618861987,38.0591553769012));
#23318=CARTESIAN_POINT('Ctrl Pts',(-41.598098082081,37.1208812263202,38.0689789363214));
#23319=CARTESIAN_POINT('Ctrl Pts',(-41.6044922701839,37.1297518617088,38.0787738136053));
#23320=CARTESIAN_POINT('Ctrl Pts',(-41.6108596213729,37.1386734506113,38.088539631424));
#23321=CARTESIAN_POINT('Ctrl Pts',(-41.6172269725618,37.147595039514,38.0983054492427));
#23322=CARTESIAN_POINT('Ctrl Pts',(-41.6235674868357,37.1565675819287,38.1080422075945));
#23323=CARTESIAN_POINT('Ctrl Pts',(-41.6298809201574,37.1655907321986,38.1177495313779));
#23324=CARTESIAN_POINT('Ctrl Pts',(-41.6361943534791,37.1746138824685,38.1274568551614));
#23325=CARTESIAN_POINT('Ctrl Pts',(-41.6424807058473,37.1836876405919,38.1371347443747));
#23326=CARTESIAN_POINT('Ctrl Pts',(-41.6487397353004,37.1928116570341,38.1467828261724));
#23327=CARTESIAN_POINT('Ctrl Pts',(-41.6549987647536,37.2019356734762,38.1564309079702));
#23328=CARTESIAN_POINT('Ctrl Pts',(-41.6612304712904,37.2111099482355,38.1660491823505));
#23329=CARTESIAN_POINT('Ctrl Pts',(-41.6674346150433,37.2203341279265,38.1756372787524));
#23330=CARTESIAN_POINT('Ctrl Pts',(-41.6736387587962,37.2295583076174,38.1852253751544));
#23331=CARTESIAN_POINT('Ctrl Pts',(-41.6798153397637,37.2388323922379,38.1947832935759));
#23332=CARTESIAN_POINT('Ctrl Pts',(-41.6859641201911,37.2481560245796,38.2043106657693));
#23333=CARTESIAN_POINT('Ctrl Pts',(-41.3471485981035,36.8220184082047,37.7065516748432));
#23334=CARTESIAN_POINT('Ctrl Pts',(-41.3545393602976,36.8299531375333,37.7174786109716));
#23335=CARTESIAN_POINT('Ctrl Pts',(-41.3619042218529,36.8379485277722,37.7283790161319));
#23336=CARTESIAN_POINT('Ctrl Pts',(-41.3692428685891,36.8460042378472,37.7392524253368));
#23337=CARTESIAN_POINT('Ctrl Pts',(-41.3765749989477,36.8540527948257,37.7501161794591));
#23338=CARTESIAN_POINT('Ctrl Pts',(-41.3838809610326,36.8621615645735,37.7609529855544));
#23339=CARTESIAN_POINT('Ctrl Pts',(-41.3911604437533,36.8703302018164,37.7717623821877));
#23340=CARTESIAN_POINT('Ctrl Pts',(-41.3984399264739,36.8784988390592,37.782571778821));
#23341=CARTESIAN_POINT('Ctrl Pts',(-41.4056929298286,36.8867273437952,37.7933537659895));
#23342=CARTESIAN_POINT('Ctrl Pts',(-41.4129191449819,36.8950153656514,37.8041078845926));
#23343=CARTESIAN_POINT('Ctrl Pts',(-41.4201453601353,36.9033033875077,37.8148620031957));
#23344=CARTESIAN_POINT('Ctrl Pts',(-41.4273447870854,36.9116509264823,37.8255882532307));
#23345=CARTESIAN_POINT('Ctrl Pts',(-41.4345171192782,36.9200576271341,37.8362861779701));
#23346=CARTESIAN_POINT('Ctrl Pts',(-41.441689451471,36.928464327786,37.8469841027093));
#23347=CARTESIAN_POINT('Ctrl Pts',(-41.4488346889047,36.9369301901129,37.8576537021504));
#23348=CARTESIAN_POINT('Ctrl Pts',(-41.4559525273326,36.9454548536356,37.8682945219779));
#23349=CARTESIAN_POINT('Ctrl Pts',(-41.4630703657605,36.9539795171584,37.8789353418053));
#23350=CARTESIAN_POINT('Ctrl Pts',(-41.4701608051808,36.9625629818748,37.8895473820166));
#23351=CARTESIAN_POINT('Ctrl Pts',(-41.4772235436802,36.9712048822978,37.9001301907472));
#23352=CARTESIAN_POINT('Ctrl Pts',(-41.4842862821795,36.9798467827208,37.9107129994779));
#23353=CARTESIAN_POINT('Ctrl Pts',(-41.4913213197562,36.9885471188485,37.9212665767253));
#23354=CARTESIAN_POINT('Ctrl Pts',(-41.4983283568557,36.9973055202173,37.9317904731145));
#23355=CARTESIAN_POINT('Ctrl Pts',(-41.5053353939552,37.0060639215861,37.9423143695036));
#23356=CARTESIAN_POINT('Ctrl Pts',(-41.512314430576,37.0148803881939,37.952808585032));
#23357=CARTESIAN_POINT('Ctrl Pts',(-41.5192651695481,37.0237545446324,37.9632726728521));
#23358=CARTESIAN_POINT('Ctrl Pts',(-41.5262159085202,37.0326287010711,37.9737367606722));
#23359=CARTESIAN_POINT('Ctrl Pts',(-41.5331383498419,37.0415605473383,37.9841707207815));
#23360=CARTESIAN_POINT('Ctrl Pts',(-41.5400321987533,37.0505497031129,37.9945741088983));
#23361=CARTESIAN_POINT('Ctrl Pts',(-41.5469260476646,37.0595388588875,38.0049774970151));
#23362=CARTESIAN_POINT('Ctrl Pts',(-41.553791304164,37.0685853241673,38.0153503131368));
#23363=CARTESIAN_POINT('Ctrl Pts',(-41.5606276759261,37.0776887137508,38.0256921155853));
#23364=CARTESIAN_POINT('Ctrl Pts',(-41.5674640476884,37.0867921033341,38.0360339180337));
#23365=CARTESIAN_POINT('Ctrl Pts',(-41.5742715347118,37.0959524172188,38.0463447068064));
#23366=CARTESIAN_POINT('Ctrl Pts',(-41.5810498471313,37.1051692653554,38.0566240428664));
#23367=CARTESIAN_POINT('Ctrl Pts',(-41.5878281595508,37.114386113492,38.0669033789262));
#23368=CARTESIAN_POINT('Ctrl Pts',(-41.5945772973647,37.1236594958782,38.0771512622708));
#23369=CARTESIAN_POINT('Ctrl Pts',(-41.6012969731922,37.1329890176503,38.0873672565416));
#23370=CARTESIAN_POINT('Ctrl Pts',(-41.6080166490197,37.1423185394222,38.0975832508123));
#23371=CARTESIAN_POINT('Ctrl Pts',(-41.6147068628593,37.1517042005777,38.1077673560068));
#23372=CARTESIAN_POINT('Ctrl Pts',(-41.6213673298393,37.1611456014718,38.1179191384821));
#23373=CARTESIAN_POINT('Ctrl Pts',(-41.6280277968192,37.1705870023659,38.1280709209575));
#23374=CARTESIAN_POINT('Ctrl Pts',(-41.6346585169379,37.1800841429965,38.1381903807112));
#23375=CARTESIAN_POINT('Ctrl Pts',(-41.641259207857,37.1896366189718,38.1482770868531));
#23376=CARTESIAN_POINT('Ctrl Pts',(-41.647859898776,37.199189094947,38.1583637929951));
#23377=CARTESIAN_POINT('Ctrl Pts',(-41.6544305604938,37.2087969062648,38.1684177455228));
#23378=CARTESIAN_POINT('Ctrl Pts',(-41.6609709132292,37.218459643821,38.1784385163354));
#23379=CARTESIAN_POINT('Ctrl Pts',(-41.6675112659646,37.2281223813771,38.1884592871481));
#23380=CARTESIAN_POINT('Ctrl Pts',(-41.6740213097158,37.2378400451691,38.1984468762429));
#23381=CARTESIAN_POINT('Ctrl Pts',(-41.6805007672835,37.247612221416,38.2084008583455));
#23382=CARTESIAN_POINT('Ctrl Pts',(-41.323840382045,36.8039758164394,37.688053225496));
#23383=CARTESIAN_POINT('Ctrl Pts',(-41.3316406739716,36.8121870614232,37.6994899722748));
#23384=CARTESIAN_POINT('Ctrl Pts',(-41.3394129600866,36.8204647408363,37.7108980929574));
#23385=CARTESIAN_POINT('Ctrl Pts',(-41.347156880221,36.8288084705036,37.7222770585544));
#23386=CARTESIAN_POINT('Ctrl Pts',(-41.3548939241138,36.8371447913263,37.7336459201582));
#23387=CARTESIAN_POINT('Ctrl Pts',(-41.3626026523888,36.845547045163,37.7449856784364));
#23388=CARTESIAN_POINT('Ctrl Pts',(-41.3702827084734,36.8540148427975,37.7562958085134));
#23389=CARTESIAN_POINT('Ctrl Pts',(-41.377962764558,36.8624826404318,37.7676059385904));
#23390=CARTESIAN_POINT('Ctrl Pts',(-41.3856141484502,36.8710159818614,37.7788864404632));
#23391=CARTESIAN_POINT('Ctrl Pts',(-41.3932365062244,36.8796144718241,37.7901367919919));
#23392=CARTESIAN_POINT('Ctrl Pts',(-41.4008588639986,36.8882129617867,37.8013871435206));
#23393=CARTESIAN_POINT('Ctrl Pts',(-41.4084521956528,36.8968766002798,37.8126073447022));
#23394=CARTESIAN_POINT('Ctrl Pts',(-41.4160161499413,36.9056049860313,37.8237968761807));
#23395=CARTESIAN_POINT('Ctrl Pts',(-41.4235801042298,36.9143333717828,37.8349864076591));
#23396=CARTESIAN_POINT('Ctrl Pts',(-41.4311146811504,36.9231265047903,37.8461452694313));
#23397=CARTESIAN_POINT('Ctrl Pts',(-41.4386195321694,36.9319839778089,37.8572729449729));
#23398=CARTESIAN_POINT('Ctrl Pts',(-41.4461243831884,36.9408414508275,37.8684006205145));
#23399=CARTESIAN_POINT('Ctrl Pts',(-41.4535995083036,36.9497632638546,37.8794971098223));
#23400=CARTESIAN_POINT('Ctrl Pts',(-41.4610445617253,36.9587490037103,37.890561899251));
#23401=CARTESIAN_POINT('Ctrl Pts',(-41.4684896151469,36.967734743566,37.9016266886797));
#23402=CARTESIAN_POINT('Ctrl Pts',(-41.475904596873,36.9767844102475,37.9126597782262));
#23403=CARTESIAN_POINT('Ctrl Pts',(-41.4832891638893,36.9858975846777,37.9236606571714));
#23404=CARTESIAN_POINT('Ctrl Pts',(-41.4906737309056,36.9950107591077,37.9346615361166));
#23405=CARTESIAN_POINT('Ctrl Pts',(-41.4980278832102,37.0041874412838,37.9456302044575));
#23406=CARTESIAN_POINT('Ctrl Pts',(-41.5053512805964,37.0134272062696,37.9565661544483));
#23407=CARTESIAN_POINT('Ctrl Pts',(-41.5126746779825,37.0226669712554,37.9675021044391));
#23408=CARTESIAN_POINT('Ctrl Pts',(-41.5199673204481,37.0319698190485,37.9784053360766));
#23409=CARTESIAN_POINT('Ctrl Pts',(-41.527228870625,37.041335318893,37.9892753446353));
#23410=CARTESIAN_POINT('Ctrl Pts',(-41.534490420802,37.0507008187375,38.0001453531939));
#23411=CARTESIAN_POINT('Ctrl Pts',(-41.5417208786882,37.0601289706308,38.0109821386705));
#23412=CARTESIAN_POINT('Ctrl Pts',(-41.5489199097852,37.0696193380372,38.0217851994057));
#23413=CARTESIAN_POINT('Ctrl Pts',(-41.5561189408822,37.0791097054437,38.032588260141));
#23414=CARTESIAN_POINT('Ctrl Pts',(-41.5632865451879,37.0886622883605,38.0433575961318));
#23415=CARTESIAN_POINT('Ctrl Pts',(-41.5704223911043,37.0982766445122,38.0540927088314));
#23416=CARTESIAN_POINT('Ctrl Pts',(-41.5775582370206,37.1078910006639,38.064827821531));
#23417=CARTESIAN_POINT('Ctrl Pts',(-41.5846623245454,37.1175671300478,38.0755287109364));
#23418=CARTESIAN_POINT('Ctrl Pts',(-41.5917343250115,37.1273045846892,38.0861948816592));
#23419=CARTESIAN_POINT('Ctrl Pts',(-41.5988063254775,37.1370420393306,38.0968610523819));
#23420=CARTESIAN_POINT('Ctrl Pts',(-41.6058462388828,37.1468408192267,38.1074925044191));
#23421=CARTESIAN_POINT('Ctrl Pts',(-41.6128537395211,37.156700470745,38.1180887455863));
#23422=CARTESIAN_POINT('Ctrl Pts',(-41.6198612401594,37.1665601222634,38.1286849867535));
#23423=CARTESIAN_POINT('Ctrl Pts',(-41.6268363280286,37.1764806454011,38.1392460170477));
#23424=CARTESIAN_POINT('Ctrl Pts',(-41.6337786804136,37.1864615809095,38.1497713475339));
#23425=CARTESIAN_POINT('Ctrl Pts',(-41.6407210327985,37.1964425164179,38.16029667802));
#23426=CARTESIAN_POINT('Ctrl Pts',(-41.6476306496972,37.2064838642941,38.1707863086951));
#23427=CARTESIAN_POINT('Ctrl Pts',(-41.6545072114151,37.2165851597154,38.1812397539184));
#23428=CARTESIAN_POINT('Ctrl Pts',(-41.661383773133,37.2266864551368,38.1916931991416));
#23429=CARTESIAN_POINT('Ctrl Pts',(-41.6682272796678,37.2368476981002,38.2021104589099));
#23430=CARTESIAN_POINT('Ctrl Pts',(-41.6750374143759,37.2470684182525,38.2124910509217));
#23431=CARTESIAN_POINT('Ctrl Pts',(-41.300739486661,36.7866666524049,37.6701054954137));
#23432=CARTESIAN_POINT('Ctrl Pts',(-41.308946338799,36.7951351177238,37.6820419472366));
#23433=CARTESIAN_POINT('Ctrl Pts',(-41.3171230440224,36.8036760900231,37.6939476530182));
#23434=CARTESIAN_POINT('Ctrl Pts',(-41.325269190303,36.8122891381963,37.7058220124267));
#23435=CARTESIAN_POINT('Ctrl Pts',(-41.3334081031839,36.8208945383825,37.7176858279554));
#23436=CARTESIAN_POINT('Ctrl Pts',(-41.3415165113648,36.8295718864962,37.7295183527505));
#23437=CARTESIAN_POINT('Ctrl Pts',(-41.3495940069763,36.8383207453626,37.74131899122));
#23438=CARTESIAN_POINT('Ctrl Pts',(-41.3576715025878,36.847069604229,37.7531196296895));
#23439=CARTESIAN_POINT('Ctrl Pts',(-41.3657180856273,36.8558899738451,37.7648883818295));
#23440=CARTESIAN_POINT('Ctrl Pts',(-41.3737333513292,36.8647814098646,37.7766246552502));
#23441=CARTESIAN_POINT('Ctrl Pts',(-41.3817486170311,36.8736728458841,37.7883609286707));
#23442=CARTESIAN_POINT('Ctrl Pts',(-41.3897325653926,36.882635348304,37.800064723368));
#23443=CARTESIAN_POINT('Ctrl Pts',(-41.3976847947922,36.8916684656507,37.811735450213));
#23444=CARTESIAN_POINT('Ctrl Pts',(-41.4056370241918,36.9007015829975,37.823406177058));
#23445=CARTESIAN_POINT('Ctrl Pts',(-41.4135575346268,36.9098053152681,37.8350438360469));
#23446=CARTESIAN_POINT('Ctrl Pts',(-41.4214459276598,36.9189792039071,37.8466478413707));
#23447=CARTESIAN_POINT('Ctrl Pts',(-41.4293343206928,36.928153092546,37.8582518466945));
#23448=CARTESIAN_POINT('Ctrl Pts',(-41.4371905963211,36.9373971375502,37.8698221983494));
#23449=CARTESIAN_POINT('Ctrl Pts',(-41.4450143593312,36.9467108733282,37.8813583139049));
#23450=CARTESIAN_POINT('Ctrl Pts',(-41.4528381223413,36.9560246091062,37.8928944294605));
#23451=CARTESIAN_POINT('Ctrl Pts',(-41.4606293727305,36.9654080356548,37.9043963089128));
#23452=CARTESIAN_POINT('Ctrl Pts',(-41.4683877185487,36.9748606803929,37.9158633732683));
#23453=CARTESIAN_POINT('Ctrl Pts',(-41.476146064367,36.9843133251309,37.9273304376238));
#23454=CARTESIAN_POINT('Ctrl Pts',(-41.4838715055346,36.9938351879875,37.9387626868187));
#23455=CARTESIAN_POINT('Ctrl Pts',(-41.491563653561,37.0034257895769,37.9501595454759));
#23456=CARTESIAN_POINT('Ctrl Pts',(-41.4992558015874,37.0130163911663,37.9615564041331));
#23457=CARTESIAN_POINT('Ctrl Pts',(-41.5069146564582,37.0226757314765,37.9729178722397));
#23458=CARTESIAN_POINT('Ctrl Pts',(-41.5145398327278,37.0324033239651,37.9842433777404));
#23459=CARTESIAN_POINT('Ctrl Pts',(-41.5221650089974,37.0421309164538,37.9955688832409));
#23460=CARTESIAN_POINT('Ctrl Pts',(-41.5297565067344,37.0519267611811,38.006858426187));
#23461=CARTESIAN_POINT('Ctrl Pts',(-41.5373139440122,37.0617903648834,38.0181114382409));
#23462=CARTESIAN_POINT('Ctrl Pts',(-41.5448713812901,37.0716539685857,38.0293644502947));
#23463=CARTESIAN_POINT('Ctrl Pts',(-41.5523947581062,37.0815853312599,38.0405809314524));
#23464=CARTESIAN_POINT('Ctrl Pts',(-41.5598836959522,37.0915839528458,38.0517603170423));
#23465=CARTESIAN_POINT('Ctrl Pts',(-41.5673726337982,37.1015825744317,38.0629397026322));
#23466=CARTESIAN_POINT('Ctrl Pts',(-41.5748271326715,37.1116484549262,38.0740819926505));
#23467=CARTESIAN_POINT('Ctrl Pts',(-41.5822468175192,37.1217810875226,38.0851866261479));
#23468=CARTESIAN_POINT('Ctrl Pts',(-41.589666502367,37.1319137201192,38.0962912596452));
#23469=CARTESIAN_POINT('Ctrl Pts',(-41.5970513731868,37.1421131048144,38.107358236618));
#23470=CARTESIAN_POINT('Ctrl Pts',(-41.604401058419,37.1523787281061,38.1183869998953));
#23471=CARTESIAN_POINT('Ctrl Pts',(-41.6117507436512,37.1626443513978,38.1294157631727));
#23472=CARTESIAN_POINT('Ctrl Pts',(-41.6190652432934,37.1729762132827,38.1404063127509));
#23473=CARTESIAN_POINT('Ctrl Pts',(-41.6263441893162,37.1833737936141,38.1513580952935));
#23474=CARTESIAN_POINT('Ctrl Pts',(-41.6336231353391,37.1937713739454,38.1623098778361));
#23475=CARTESIAN_POINT('Ctrl Pts',(-41.6408665277401,37.2042346727198,38.1732228933392));
#23476=CARTESIAN_POINT('Ctrl Pts',(-41.6480740020571,37.2147631631981,38.184096592356));
#23477=CARTESIAN_POINT('Ctrl Pts',(-41.6552814763742,37.2252916536764,38.1949702913728));
#23478=CARTESIAN_POINT('Ctrl Pts',(-41.6624530326048,37.2358853358551,38.2058046738995));
#23479=CARTESIAN_POINT('Ctrl Pts',(-41.6695883098903,37.2465436764554,38.2165991944336));
#23480=CARTESIAN_POINT('Ctrl Pts',(-41.277913517507,36.7700593990031,37.6527056210249));
#23481=CARTESIAN_POINT('Ctrl Pts',(-41.2865220517812,36.7787672739902,37.665131206525));
#23482=CARTESIAN_POINT('Ctrl Pts',(-41.2950982902937,36.7875539692752,37.6775239293325));
#23483=CARTESIAN_POINT('Ctrl Pts',(-41.3036417632543,36.7964190035341,37.6898831105967));
#23484=CARTESIAN_POINT('Ctrl Pts',(-41.3121776500075,36.8052761660542,37.7022313174816));
#23485=CARTESIAN_POINT('Ctrl Pts',(-41.3206808293679,36.8142115284835,37.7145460423583));
#23486=CARTESIAN_POINT('Ctrl Pts',(-41.3291508363723,36.8232246022265,37.726826611844));
#23487=CARTESIAN_POINT('Ctrl Pts',(-41.3376208433767,36.8322376759696,37.7391071813297));
#23488=CARTESIAN_POINT('Ctrl Pts',(-41.3460576780217,36.8413284610227,37.7513535954195));
#23489=CARTESIAN_POINT('Ctrl Pts',(-41.3544608789718,36.8504964602918,37.7635651844659));
#23490=CARTESIAN_POINT('Ctrl Pts',(-41.3628640799219,36.8596644595609,37.7757767735122));
#23491=CARTESIAN_POINT('Ctrl Pts',(-41.3712336471738,36.8689096730424,37.7879535375104));
#23492=CARTESIAN_POINT('Ctrl Pts',(-41.3795691230703,36.8782315951976,37.8000948106213));
#23493=CARTESIAN_POINT('Ctrl Pts',(-41.3879045989668,36.8875535173528,37.8122360837323));
#23494=CARTESIAN_POINT('Ctrl Pts',(-41.3962059835046,36.8969521481781,37.8243418659513));
#23495=CARTESIAN_POINT('Ctrl Pts',(-41.4044728227548,36.906426973746,37.8364114953207));
#23496=CARTESIAN_POINT('Ctrl Pts',(-41.4127396620049,36.9159017993139,37.84848112469));
#23497=CARTESIAN_POINT('Ctrl Pts',(-41.4209719559642,36.9254528196206,37.8605146012051));
#23498=CARTESIAN_POINT('Ctrl Pts',(-41.4291692544817,36.9350795124057,37.8725112668619));
#23499=CARTESIAN_POINT('Ctrl Pts',(-41.4373665529991,36.9447062051908,37.8845079325187));
#23500=CARTESIAN_POINT('Ctrl Pts',(-41.4455288560714,36.9544085704505,37.8964677873126));
#23501=CARTESIAN_POINT('Ctrl Pts',(-41.4536557173749,36.9641860776488,37.9083901772654));
#23502=CARTESIAN_POINT('Ctrl Pts',(-41.4617825786783,36.973963584847,37.9203125672183));
#23503=CARTESIAN_POINT('Ctrl Pts',(-41.469873998137,36.9838162339168,37.9321974922695));
#23504=CARTESIAN_POINT('Ctrl Pts',(-41.4779295334512,36.9937434862326,37.9440443026519));
#23505=CARTESIAN_POINT('Ctrl Pts',(-41.4859850687655,37.0036707385483,37.9558911130344));
#23506=CARTESIAN_POINT('Ctrl Pts',(-41.494004719921,37.0136725940981,37.967699808735));
#23507=CARTESIAN_POINT('Ctrl Pts',(-41.5019880482629,37.0237485058532,37.9794697439402));
#23508=CARTESIAN_POINT('Ctrl Pts',(-41.5099713766048,37.0338244176084,37.9912396791453));
#23509=CARTESIAN_POINT('Ctrl Pts',(-41.5179183821971,37.0439743856239,38.0029708539018));
#23510=CARTESIAN_POINT('Ctrl Pts',(-41.5258286304887,37.0541978548883,38.0146626267361));
#23511=CARTESIAN_POINT('Ctrl Pts',(-41.5337388787803,37.0644213241527,38.0263543995704));
#23512=CARTESIAN_POINT('Ctrl Pts',(-41.5416123697679,37.0747182946621,38.0380067704779));
#23513=CARTESIAN_POINT('Ctrl Pts',(-41.5494486729206,37.0850882033665,38.0496191022939));
#23514=CARTESIAN_POINT('Ctrl Pts',(-41.5572849760732,37.0954581120709,38.06123143411));
#23515=CARTESIAN_POINT('Ctrl Pts',(-41.5650840913877,37.1059009589663,38.07280372683));
#23516=CARTESIAN_POINT('Ctrl Pts',(-41.5728455923997,37.1164161730263,38.0843353476683));
#23517=CARTESIAN_POINT('Ctrl Pts',(-41.5806070934118,37.1269313870862,38.0958669685066));
#23518=CARTESIAN_POINT('Ctrl Pts',(-41.5883309801183,37.1375189683066,38.1073579174584));
#23519=CARTESIAN_POINT('Ctrl Pts',(-41.5960168301686,37.1481783377467,38.1188075661862));
#23520=CARTESIAN_POINT('Ctrl Pts',(-41.6037026802189,37.1588377071868,38.1302572149139));
#23521=CARTESIAN_POINT('Ctrl Pts',(-41.61135049361,37.1695688648423,38.1416655634129));
#23522=CARTESIAN_POINT('Ctrl Pts',(-41.618959852151,37.1803712239218,38.1530319878621));
#23523=CARTESIAN_POINT('Ctrl Pts',(-41.6265692106919,37.1911735830013,38.1643984123112));
#23524=CARTESIAN_POINT('Ctrl Pts',(-41.6341401143796,37.2020471435004,38.1757229127059));
#23525=CARTESIAN_POINT('Ctrl Pts',(-41.6416721492288,37.2129913108407,38.1870048698101));
#23526=CARTESIAN_POINT('Ctrl Pts',(-41.649204184078,37.2239354781811,38.1982868269143));
#23527=CARTESIAN_POINT('Ctrl Pts',(-41.6566973500857,37.2349502523584,38.2095262407234));
#23528=CARTESIAN_POINT('Ctrl Pts',(-41.6641512375171,37.2460350310726,38.2207224966539));
#23529=CARTESIAN_POINT('Ctrl Pts',(-41.2322615791988,36.7368448921995,37.6179058722475));
#23530=CARTESIAN_POINT('Ctrl Pts',(-41.2416734777457,36.7460315865228,37.6313097251018));
#23531=CARTESIAN_POINT('Ctrl Pts',(-41.2510487828363,36.7553097277793,37.6446764819612));
#23532=CARTESIAN_POINT('Ctrl Pts',(-41.2603869091568,36.7646787342098,37.6580053069365));
#23533=CARTESIAN_POINT('Ctrl Pts',(-41.2697167436546,36.7740394213977,37.671322296534));
#23534=CARTESIAN_POINT('Ctrl Pts',(-41.2790094653743,36.7834908124581,37.6846014215741));
#23535=CARTESIAN_POINT('Ctrl Pts',(-41.2882644951643,36.7930323159545,37.6978418530921));
#23536=CARTESIAN_POINT('Ctrl Pts',(-41.2975195249545,36.8025738194508,37.7110822846101));
#23537=CARTESIAN_POINT('Ctrl Pts',(-41.3067368628103,36.812205435378,37.7242840225993));
#23538=CARTESIAN_POINT('Ctrl Pts',(-41.315915934257,36.8219265611464,37.7374462428973));
#23539=CARTESIAN_POINT('Ctrl Pts',(-41.3250950057036,36.8316476869147,37.7506084631952));
#23540=CARTESIAN_POINT('Ctrl Pts',(-41.3342358107362,36.8414583225193,37.7637311657951));
#23541=CARTESIAN_POINT('Ctrl Pts',(-41.3433377796266,36.8513578542914,37.776813531438));
#23542=CARTESIAN_POINT('Ctrl Pts',(-41.3524397485169,36.8612573860636,37.7898958970809));
#23543=CARTESIAN_POINT('Ctrl Pts',(-41.3615028812602,36.8712458139983,37.8029379257601));
#23544=CARTESIAN_POINT('Ctrl Pts',(-41.3705266129447,36.881322513424,37.8159388032206));
#23545=CARTESIAN_POINT('Ctrl Pts',(-41.3795503446293,36.8913992128497,37.8289396806812));
#23546=CARTESIAN_POINT('Ctrl Pts',(-41.3885346752505,36.9015641837612,37.8418994069165));
#23547=CARTESIAN_POINT('Ctrl Pts',(-41.3974790447827,36.9118167905605,37.8548171727759));
#23548=CARTESIAN_POINT('Ctrl Pts',(-41.4064234143148,36.9220693973599,37.8677349386352));
#23549=CARTESIAN_POINT('Ctrl Pts',(-41.4153278227533,36.9324096400418,37.8806107441121));
#23550=CARTESIAN_POINT('Ctrl Pts',(-41.4241917150271,36.9428368721605,37.8934437852596));
#23551=CARTESIAN_POINT('Ctrl Pts',(-41.433055607301,36.9532641042791,37.9062768264071));
#23552=CARTESIAN_POINT('Ctrl Pts',(-41.4418789833418,36.9637783257753,37.919067103171));
#23553=CARTESIAN_POINT('Ctrl Pts',(-41.4506612932317,36.9743788795439,37.931813817004));
#23554=CARTESIAN_POINT('Ctrl Pts',(-41.4594436031217,36.9849794333125,37.944560530837));
#23555=CARTESIAN_POINT('Ctrl Pts',(-41.4681848468466,36.9956663193414,37.9572636817256));
#23556=CARTESIAN_POINT('Ctrl Pts',(-41.4768844793332,37.0064388696294,37.9699224763397));
#23557=CARTESIAN_POINT('Ctrl Pts',(-41.4855841118197,37.0172114199174,37.9825812709539));
#23558=CARTESIAN_POINT('Ctrl Pts',(-41.4942421331226,37.0280696345095,37.9951957093312));
#23559=CARTESIAN_POINT('Ctrl Pts',(-41.5028580034416,37.0390128348981,38.0077650037266));
#23560=CARTESIAN_POINT('Ctrl Pts',(-41.5114738737606,37.0499560352868,38.0203342981219));
#23561=CARTESIAN_POINT('Ctrl Pts',(-41.5200475930913,37.0609842214665,38.0328584485288));
#23562=CARTESIAN_POINT('Ctrl Pts',(-41.5285786268573,37.0720967044079,38.0453366727972));
#23563=CARTESIAN_POINT('Ctrl Pts',(-41.5371096606233,37.0832091873492,38.0578148970656));
#23564=CARTESIAN_POINT('Ctrl Pts',(-41.5455980088201,37.0944059670466,38.0702471951892));
#23565=CARTESIAN_POINT('Ctrl Pts',(-41.5540431421607,37.1056863440336,38.0826327907092));
#23566=CARTESIAN_POINT('Ctrl Pts',(-41.5624882755012,37.1169667210205,38.0950183862292));
#23567=CARTESIAN_POINT('Ctrl Pts',(-41.5708901939812,37.1283306952912,38.1073572791394));
#23568=CARTESIAN_POINT('Ctrl Pts',(-41.5792483736678,37.1397775570278,38.1196486987679));
#23569=CARTESIAN_POINT('Ctrl Pts',(-41.5876065533543,37.1512244187646,38.1319401183963));
#23570=CARTESIAN_POINT('Ctrl Pts',(-41.5959209942432,37.1627541679616,38.1441840647368));
#23571=CARTESIAN_POINT('Ctrl Pts',(-41.6041911778204,37.1743660845373,38.1563797729991));
#23572=CARTESIAN_POINT('Ctrl Pts',(-41.6124613613976,37.185978001113,38.1685754812615));
#23573=CARTESIAN_POINT('Ctrl Pts',(-41.6206872876587,37.1976720850615,38.1807229514394));
#23574=CARTESIAN_POINT('Ctrl Pts',(-41.6288684435722,37.209447606126,38.1928214247184));
#23575=CARTESIAN_POINT('Ctrl Pts',(-41.6370495994857,37.2212231271905,38.2049198979974));
#23576=CARTESIAN_POINT('Ctrl Pts',(-41.6451859850473,37.233080085365,38.2169693743713));
#23577=CARTESIAN_POINT('Ctrl Pts',(-41.6532770927708,37.2450177403072,38.2289691010946));
#23578=CARTESIAN_POINT('Ctrl Pts',(-41.1877289817149,36.7064399824573,37.5853042020928));
#23579=CARTESIAN_POINT('Ctrl Pts',(-41.1979242219596,36.7160343690079,37.5996437919289));
#23580=CARTESIAN_POINT('Ctrl Pts',(-41.2080785460692,36.7257337815324,37.6139420716953));
#23581=CARTESIAN_POINT('Ctrl Pts',(-41.2181912296561,36.7355375248302,37.6281980198277));
#23582=CARTESIAN_POINT('Ctrl Pts',(-41.2282949336494,36.7453325628591,37.64244130934));
#23583=CARTESIAN_POINT('Ctrl Pts',(-41.2383570710302,36.755231746455,37.6566423423526));
#23584=CARTESIAN_POINT('Ctrl Pts',(-41.2483769252352,36.7652343675505,37.6708001060175));
#23585=CARTESIAN_POINT('Ctrl Pts',(-41.2583967794402,36.775236988646,37.6849578696824));
#23586=CARTESIAN_POINT('Ctrl Pts',(-41.2683743504628,36.7853430472343,37.6990723639902));
#23587=CARTESIAN_POINT('Ctrl Pts',(-41.2783089277365,36.7955518206302,37.7131425822324));
#23588=CARTESIAN_POINT('Ctrl Pts',(-41.2882435050103,36.8057605940261,37.7272128004746));
#23589=CARTESIAN_POINT('Ctrl Pts',(-41.2981350885286,36.8160720822226,37.7412387426419));
#23590=CARTESIAN_POINT('Ctrl Pts',(-41.307982973821,36.8264855480185,37.755219408306));
#23591=CARTESIAN_POINT('Ctrl Pts',(-41.3178308591135,36.8368990138144,37.7692000739701));
#23592=CARTESIAN_POINT('Ctrl Pts',(-41.3276350461735,36.8474144572026,37.7831354631218));
#23593=CARTESIAN_POINT('Ctrl Pts',(-41.3373948367249,36.8580311265692,37.7970245817532));
#23594=CARTESIAN_POINT('Ctrl Pts',(-41.3471546272764,36.8686477959358,37.8109137003846));
#23595=CARTESIAN_POINT('Ctrl Pts',(-41.3568700213129,36.8793656912737,37.8247565484865));
#23596=CARTESIAN_POINT('Ctrl Pts',(-41.3665403268503,36.8901840466619,37.8385521386106));
#23597=CARTESIAN_POINT('Ctrl Pts',(-41.3762106323877,36.90100240205,37.8523477287347));
#23598=CARTESIAN_POINT('Ctrl Pts',(-41.3858358494196,36.9119212174812,37.8660960608719));
#23599=CARTESIAN_POINT('Ctrl Pts',(-41.3954152923506,36.9229397128349,37.8797961542715));
#23600=CARTESIAN_POINT('Ctrl Pts',(-41.4049947352816,36.9339582081886,37.8934962476712));
#23601=CARTESIAN_POINT('Ctrl Pts',(-41.4145284041053,36.9450763834573,37.9071481023244));
#23602=CARTESIAN_POINT('Ctrl Pts',(-41.4240156197108,36.9562934444306,37.9207507443156));
#23603=CARTESIAN_POINT('Ctrl Pts',(-41.4335028353163,36.9675105054037,37.9343533863069));
#23604=CARTESIAN_POINT('Ctrl Pts',(-41.4429435976973,36.9788264520739,37.9479068156272));
#23605=CARTESIAN_POINT('Ctrl Pts',(-41.4523372343223,36.9902404762517,37.9614100653328));
#23606=CARTESIAN_POINT('Ctrl Pts',(-41.4617308709474,37.0016545004295,37.9749133150385));
#23607=CARTESIAN_POINT('Ctrl Pts',(-41.4710773818102,37.0131666021072,37.9883663851205));
#23608=CARTESIAN_POINT('Ctrl Pts',(-41.4803761010527,37.0247759592303,38.001768315742));
#23609=CARTESIAN_POINT('Ctrl Pts',(-41.4896748202951,37.0363853163534,38.0151702463634));
#23610=CARTESIAN_POINT('Ctrl Pts',(-41.4989257479112,37.048091928914,38.0285210375155));
#23611=CARTESIAN_POINT('Ctrl Pts',(-41.5081282248091,37.0598949611075,38.0418197366027));
#23612=CARTESIAN_POINT('Ctrl Pts',(-41.517330701707,37.071697993301,38.0551184356899));
#23613=CARTESIAN_POINT('Ctrl Pts',(-41.5264847278807,37.0835974451195,38.0683650427034));
#23614=CARTESIAN_POINT('Ctrl Pts',(-41.5355896510973,37.0955924671253,38.0815586124227));
#23615=CARTESIAN_POINT('Ctrl Pts',(-41.5446945743139,37.107587489131,38.0947521821419));
#23616=CARTESIAN_POINT('Ctrl Pts',(-41.5537503945673,37.1196780813162,38.107892714558));
#23617=CARTESIAN_POINT('Ctrl Pts',(-41.5627564665744,37.1318633807292,38.1209792719577));
#23618=CARTESIAN_POINT('Ctrl Pts',(-41.5717625385814,37.1440486801423,38.1340658293574));
#23619=CARTESIAN_POINT('Ctrl Pts',(-41.5807188623362,37.156328686775,38.147098411732));
#23620=CARTESIAN_POINT('Ctrl Pts',(-41.5896247995955,37.1687025242832,38.1600760890065));
#23621=CARTESIAN_POINT('Ctrl Pts',(-41.5985307368549,37.1810763617914,38.1730537662811));
#23622=CARTESIAN_POINT('Ctrl Pts',(-41.6073862876129,37.1935440301667,38.1859765384471));
#23623=CARTESIAN_POINT('Ctrl Pts',(-41.6161908207558,37.2061046397946,38.1988434831987));
#23624=CARTESIAN_POINT('Ctrl Pts',(-41.6249953538988,37.2186652494225,38.2117104279504));
#23625=CARTESIAN_POINT('Ctrl Pts',(-41.6337488694209,37.2313188002946,38.2245215452789));
#23626=CARTESIAN_POINT('Ctrl Pts',(-41.6424507434257,37.244064389651,38.2372759207768));
#23627=CARTESIAN_POINT('Ctrl Pts',(-41.1444195426625,36.6783597806106,37.5546020043376));
#23628=CARTESIAN_POINT('Ctrl Pts',(-41.1553734557036,36.6883054348728,37.5698384308781));
#23629=CARTESIAN_POINT('Ctrl Pts',(-41.166282235733,36.6983703147992,37.5850294796951));
#23630=CARTESIAN_POINT('Ctrl Pts',(-41.1771449970972,36.708553603238,37.6001739174679));
#23631=CARTESIAN_POINT('Ctrl Pts',(-41.1879981128335,36.7187278493895,37.615304907683));
#23632=CARTESIAN_POINT('Ctrl Pts',(-41.1988052915835,36.7290202938554,37.6303893695809));
#23633=CARTESIAN_POINT('Ctrl Pts',(-41.2095656574962,36.7394301025007,37.6454260806647));
#23634=CARTESIAN_POINT('Ctrl Pts',(-41.220326023409,36.749839911146,37.6604627917486));
#23635=CARTESIAN_POINT('Ctrl Pts',(-41.2310395764751,36.7603670839615,37.6754517520053));
#23636=CARTESIAN_POINT('Ctrl Pts',(-41.2417054484313,36.771010767789,37.690391746678));
#23637=CARTESIAN_POINT('Ctrl Pts',(-41.2523713203876,36.7816544516165,37.7053317413507));
#23638=CARTESIAN_POINT('Ctrl Pts',(-41.2629895112246,36.7924146464467,37.7202227704263));
#23639=CARTESIAN_POINT('Ctrl Pts',(-41.2735591604079,36.8032904802363,37.7350636270846));
#23640=CARTESIAN_POINT('Ctrl Pts',(-41.2841288095911,36.8141663140259,37.7499044837429));
#23641=CARTESIAN_POINT('Ctrl Pts',(-41.2946499171111,36.8251577867655,37.7646951679709));
#23642=CARTESIAN_POINT('Ctrl Pts',(-41.3051216303013,36.8362640076682,37.7794344810807));
#23643=CARTESIAN_POINT('Ctrl Pts',(-41.3155933434915,36.8473702285709,37.7941737941905));
#23644=CARTESIAN_POINT('Ctrl Pts',(-41.3260156623427,36.8585911976271,37.8088617361692));
#23645=CARTESIAN_POINT('Ctrl Pts',(-41.3363877421943,36.8699260054509,37.8234971166555));
#23646=CARTESIAN_POINT('Ctrl Pts',(-41.3467598220459,36.8812608132747,37.8381324971418));
#23647=CARTESIAN_POINT('Ctrl Pts',(-41.3570816628888,36.892709459856,37.8527153161229));
#23648=CARTESIAN_POINT('Ctrl Pts',(-41.3673524282056,36.9042710173573,37.8672443917569));
#23649=CARTESIAN_POINT('Ctrl Pts',(-41.3776231935224,36.9158325748587,37.8817734673908));
#23650=CARTESIAN_POINT('Ctrl Pts',(-41.387842883304,36.9275070432698,37.8962487996651));
#23651=CARTESIAN_POINT('Ctrl Pts',(-41.3980106693117,36.9392934764517,37.9106692154489));
#23652=CARTESIAN_POINT('Ctrl Pts',(-41.4081784553195,36.9510799096335,37.9250896312327));
#23653=CARTESIAN_POINT('Ctrl Pts',(-41.4182943375443,36.9629783075759,37.9394551305134));
#23654=CARTESIAN_POINT('Ctrl Pts',(-41.4283574961605,36.9749877059916,37.9537645490616));
#23655=CARTESIAN_POINT('Ctrl Pts',(-41.4384206547766,36.9869971044073,37.9680739676097));
#23656=CARTESIAN_POINT('Ctrl Pts',(-41.4484310897753,36.9991175032858,37.9823273054128));
#23657=CARTESIAN_POINT('Ctrl Pts',(-41.4583879898763,37.0113479203483,37.9965234073313));
#23658=CARTESIAN_POINT('Ctrl Pts',(-41.4683448899773,37.0235783374109,38.0107195092498));
#23659=CARTESIAN_POINT('Ctrl Pts',(-41.478248255172,37.0359187726468,38.0248583752714));
#23660=CARTESIAN_POINT('Ctrl Pts',(-41.4880972828577,37.0483682259447,38.0389388595335));
#23661=CARTESIAN_POINT('Ctrl Pts',(-41.4979463105433,37.0608176792426,38.0530193437957));
#23662=CARTESIAN_POINT('Ctrl Pts',(-41.5077410007112,37.0733761505917,38.0670414462863));
#23663=CARTESIAN_POINT('Ctrl Pts',(-41.5174805595661,37.0860426222101,38.0810040306058));
#23664=CARTESIAN_POINT('Ctrl Pts',(-41.5272201184209,37.0987090938285,38.0949666149253));
#23665=CARTESIAN_POINT('Ctrl Pts',(-41.5369045459541,37.1114835657054,38.1088696810615));
#23666=CARTESIAN_POINT('Ctrl Pts',(-41.5465330573064,37.1243650025534,38.1227121022621));
#23667=CARTESIAN_POINT('Ctrl Pts',(-41.5561615686588,37.1372464394014,38.1365545234628));
#23668=CARTESIAN_POINT('Ctrl Pts',(-41.5657341638218,37.1502348412093,38.1503362997158));
#23669=CARTESIAN_POINT('Ctrl Pts',(-41.5752500669993,37.1633291553525,38.1640563140985));
#23670=CARTESIAN_POINT('Ctrl Pts',(-41.584765970177,37.1764234694955,38.1777763284813));
#23671=CARTESIAN_POINT('Ctrl Pts',(-41.5942251813608,37.1896236959624,38.1914345809818));
#23672=CARTESIAN_POINT('Ctrl Pts',(-41.603626933944,37.2029287649612,38.2050299646883));
#23673=CARTESIAN_POINT('Ctrl Pts',(-41.6130286865272,37.21623383396,38.2186253483948));
#23674=CARTESIAN_POINT('Ctrl Pts',(-41.6223729805015,37.2296437454791,38.2321578632955));
#23675=CARTESIAN_POINT('Ctrl Pts',(-41.6316590585731,37.2431574127333,38.2456264126687));
#23676=CARTESIAN_POINT('Ctrl Pts',(-41.1011101036101,36.6502795787638,37.5238998065825));
#23677=CARTESIAN_POINT('Ctrl Pts',(-41.1128226894475,36.6605765007378,37.5400330698273));
#23678=CARTESIAN_POINT('Ctrl Pts',(-41.1244859253969,36.6710068480659,37.5561168876949));
#23679=CARTESIAN_POINT('Ctrl Pts',(-41.1360987645382,36.6815696816458,37.5721498151081));
#23680=CARTESIAN_POINT('Ctrl Pts',(-41.1477012920175,36.6921231359199,37.588168506026));
#23681=CARTESIAN_POINT('Ctrl Pts',(-41.1592535121368,36.7028088412558,37.6041363968091));
#23682=CARTESIAN_POINT('Ctrl Pts',(-41.1707543897573,36.7136258374508,37.620052055312));
#23683=CARTESIAN_POINT('Ctrl Pts',(-41.1822552673778,36.7244428336459,37.6359677138148));
#23684=CARTESIAN_POINT('Ctrl Pts',(-41.1937048024874,36.7353911206887,37.6518311400204));
#23685=CARTESIAN_POINT('Ctrl Pts',(-41.2051019691261,36.7464697149479,37.6676409111236));
#23686=CARTESIAN_POINT('Ctrl Pts',(-41.2164991357649,36.757548309207,37.6834506822268));
#23687=CARTESIAN_POINT('Ctrl Pts',(-41.2278439339207,36.7687572106707,37.6992067982107));
#23688=CARTESIAN_POINT('Ctrl Pts',(-41.2391353469947,36.7800954124541,37.7149078458632));
#23689=CARTESIAN_POINT('Ctrl Pts',(-41.2504267600686,36.7914336142374,37.7306088935157));
#23690=CARTESIAN_POINT('Ctrl Pts',(-41.2616647880488,36.8029011163283,37.74625487282));
#23691=CARTESIAN_POINT('Ctrl Pts',(-41.2728484238777,36.8144968887672,37.7618443804082));
#23692=CARTESIAN_POINT('Ctrl Pts',(-41.2840320597066,36.8260926612061,37.7774338879964));
#23693=CARTESIAN_POINT('Ctrl Pts',(-41.2951613033725,36.8378167039806,37.792966923852));
#23694=CARTESIAN_POINT('Ctrl Pts',(-41.3062351575383,36.8496679642399,37.8084420947004));
#23695=CARTESIAN_POINT('Ctrl Pts',(-41.3173090117041,36.8615192244992,37.8239172655489));
#23696=CARTESIAN_POINT('Ctrl Pts',(-41.328327476358,36.8734977022308,37.8393345713738));
#23697=CARTESIAN_POINT('Ctrl Pts',(-41.3392895640606,36.8856023218798,37.8546926292421));
#23698=CARTESIAN_POINT('Ctrl Pts',(-41.3502516517632,36.8977069415287,37.8700506871105));
#23699=CARTESIAN_POINT('Ctrl Pts',(-41.3611573625028,36.9099377030822,37.8853494970058));
#23700=CARTESIAN_POINT('Ctrl Pts',(-41.3720057189127,36.9222935084728,37.9005876865821));
#23701=CARTESIAN_POINT('Ctrl Pts',(-41.3828540753226,36.9346493138634,37.9158258761585));
#23702=CARTESIAN_POINT('Ctrl Pts',(-41.3936450773913,36.9471301630778,37.9310034453995));
#23703=CARTESIAN_POINT('Ctrl Pts',(-41.4043777579986,36.9597349357315,37.9461190327902));
#23704=CARTESIAN_POINT('Ctrl Pts',(-41.4151104386059,36.9723397083851,37.9612346201809));
#23705=CARTESIAN_POINT('Ctrl Pts',(-41.4257847977404,36.9850684044644,37.9762882257051));
#23706=CARTESIAN_POINT('Ctrl Pts',(-41.4363998786999,36.9979198814664,37.9912784989207));
#23707=CARTESIAN_POINT('Ctrl Pts',(-41.4470149596595,37.0107713584684,38.0062687721363));
#23708=CARTESIAN_POINT('Ctrl Pts',(-41.4575707624329,37.0237456163795,38.0211957130272));
#23709=CARTESIAN_POINT('Ctrl Pts',(-41.4680663409063,37.0368414907819,38.0360579824644));
#23710=CARTESIAN_POINT('Ctrl Pts',(-41.4785619193796,37.0499373651843,38.0509202519016));
#23711=CARTESIAN_POINT('Ctrl Pts',(-41.4889972735417,37.0631548560639,38.0657178498691));
#23712=CARTESIAN_POINT('Ctrl Pts',(-41.4993714680348,37.0764927772949,38.0804494487889));
#23713=CARTESIAN_POINT('Ctrl Pts',(-41.5097456625279,37.0898306985261,38.0951810477086));
#23714=CARTESIAN_POINT('Ctrl Pts',(-41.520058697341,37.1032890500945,38.109846647565));
#23715=CARTESIAN_POINT('Ctrl Pts',(-41.5303096480385,37.1168666243775,38.1244449325666));
#23716=CARTESIAN_POINT('Ctrl Pts',(-41.5405605987361,37.1304441986604,38.1390432175682));
#23717=CARTESIAN_POINT('Ctrl Pts',(-41.5507494653073,37.1441409956436,38.1535741876996));
#23718=CARTESIAN_POINT('Ctrl Pts',(-41.5608753344032,37.1579557864216,38.1680365391905));
#23719=CARTESIAN_POINT('Ctrl Pts',(-41.571001203499,37.1717705771997,38.1824988906814));
#23720=CARTESIAN_POINT('Ctrl Pts',(-41.5810640751088,37.1857033617581,38.1968926235164));
#23721=CARTESIAN_POINT('Ctrl Pts',(-41.5910630471322,37.1997528901279,38.2112164461778));
#23722=CARTESIAN_POINT('Ctrl Pts',(-41.6010620191556,37.2138024184976,38.2255402688393));
#23723=CARTESIAN_POINT('Ctrl Pts',(-41.6109970915822,37.2279686906637,38.2397941813121));
#23724=CARTESIAN_POINT('Ctrl Pts',(-41.6208673737205,37.2422504358157,38.2539769045607));
#23725=CARTESIAN_POINT('Ctrl Pts',(-41.0590044066045,36.6245107757466,37.4950828317286));
#23726=CARTESIAN_POINT('Ctrl Pts',(-41.0714514561137,36.6351027502924,37.5120743871615));
#23727=CARTESIAN_POINT('Ctrl Pts',(-41.0838450412698,36.6458429750105,37.529012572385));
#23728=CARTESIAN_POINT('Ctrl Pts',(-41.0961839313899,36.6567303801302,37.5458957042908));
#23729=CARTESIAN_POINT('Ctrl Pts',(-41.1085118651484,36.6676081177397,37.5627638447592));
#23730=CARTESIAN_POINT('Ctrl Pts',(-41.1207852011292,36.6786327745861,37.5795770297387));
#23731=CARTESIAN_POINT('Ctrl Pts',(-41.13300272309,36.6898032549803,37.5963335917226));
#23732=CARTESIAN_POINT('Ctrl Pts',(-41.1452202450508,36.7009737353744,37.6130901537065));
#23733=CARTESIAN_POINT('Ctrl Pts',(-41.1573819529757,36.7122900393016,37.6297900926729));
#23734=CARTESIAN_POINT('Ctrl Pts',(-41.1694866416616,36.7237510422997,37.6464317523176));
#23735=CARTESIAN_POINT('Ctrl Pts',(-41.1815913303475,36.7352120452978,37.6630734119624));
#23736=CARTESIAN_POINT('Ctrl Pts',(-41.1936389997787,36.7468177473517,37.6796567922638));
#23737=CARTESIAN_POINT('Ctrl Pts',(-41.2056284560277,36.7585669954476,37.6961802484455));
#23738=CARTESIAN_POINT('Ctrl Pts',(-41.2176179122767,36.7703162435434,37.7127037046271));
#23739=CARTESIAN_POINT('Ctrl Pts',(-41.2295491553279,36.7822090376658,37.7291672366675));
#23740=CARTESIAN_POINT('Ctrl Pts',(-41.2414210027637,36.7942441964755,37.7455692116409));
#23741=CARTESIAN_POINT('Ctrl Pts',(-41.2532928501995,36.8062793552852,37.7619711866143));
#23742=CARTESIAN_POINT('Ctrl Pts',(-41.2651053020044,36.8184568787666,37.7783116044994));
#23743=CARTESIAN_POINT('Ctrl Pts',(-41.2768571875023,36.830775557488,37.7945888445415));
#23744=CARTESIAN_POINT('Ctrl Pts',(-41.2886090730003,36.8430942362094,37.8108660845837));
#23745=CARTESIAN_POINT('Ctrl Pts',(-41.300300392176,36.8555540701548,37.8270801467617));
#23746=CARTESIAN_POINT('Ctrl Pts',(-41.3119299863247,36.8681538220374,37.8432294228106));
#23747=CARTESIAN_POINT('Ctrl Pts',(-41.3235595804735,36.8807535739201,37.8593786988595));
#23748=CARTESIAN_POINT('Ctrl Pts',(-41.3351274494821,36.8934932436479,37.8754631886912));
#23749=CARTESIAN_POINT('Ctrl Pts',(-41.3466324470441,36.9063715664765,37.8914812969822));
#23750=CARTESIAN_POINT('Ctrl Pts',(-41.3581374446061,36.9192498893049,37.9074994052732));
#23751=CARTESIAN_POINT('Ctrl Pts',(-41.3695795706916,36.9322668652086,37.9234511319931));
#23752=CARTESIAN_POINT('Ctrl Pts',(-41.3809576910404,36.9454212017859,37.9393348946783));
#23753=CARTESIAN_POINT('Ctrl Pts',(-41.3923358113892,36.9585755383631,37.9552186573635));
#23754=CARTESIAN_POINT('Ctrl Pts',(-41.4036499260769,36.9718672356681,37.9710344560556));
#23755=CARTESIAN_POINT('Ctrl Pts',(-41.4148989136667,36.9852949743307,37.9867807218423));
#23756=CARTESIAN_POINT('Ctrl Pts',(-41.4261479012565,36.9987227129934,38.0025269876289));
#23757=CARTESIAN_POINT('Ctrl Pts',(-41.4373317617337,37.0122864929962,38.0182037204896));
#23758=CARTESIAN_POINT('Ctrl Pts',(-41.4484493865271,37.0259849681195,38.0338093652491));
#23759=CARTESIAN_POINT('Ctrl Pts',(-41.4595670113204,37.0396834432429,38.0494150100086));
#23760=CARTESIAN_POINT('Ctrl Pts',(-41.4706184004156,37.0535166134687,38.0649495666467));
#23761=CARTESIAN_POINT('Ctrl Pts',(-41.4816024583245,37.0674831059924,38.0804114940307));
#23762=CARTESIAN_POINT('Ctrl Pts',(-41.4925865162334,37.081449598516,38.0958734214147));
#23763=CARTESIAN_POINT('Ctrl Pts',(-41.503503242942,37.0955494133191,38.1112627195244));
#23764=CARTESIAN_POINT('Ctrl Pts',(-41.5143515562604,37.1097811512812,38.1265778615725));
#23765=CARTESIAN_POINT('Ctrl Pts',(-41.5251998695787,37.1240128892433,38.1418930036207));
#23766=CARTESIAN_POINT('Ctrl Pts',(-41.5359797694928,37.1383765503461,38.1571339895872));
#23767=CARTESIAN_POINT('Ctrl Pts',(-41.5466901873235,37.1528707094282,38.1722993073297));
#23768=CARTESIAN_POINT('Ctrl Pts',(-41.5574006051541,37.1673648685103,38.1874646250722));
#23769=CARTESIAN_POINT('Ctrl Pts',(-41.5680415408875,37.181989525553,38.2025542745711));
#23770=CARTESIAN_POINT('Ctrl Pts',(-41.5786119395645,37.1967432296344,38.2175667586257));
#23771=CARTESIAN_POINT('Ctrl Pts',(-41.5891823382414,37.2114969337158,38.2325792426804));
#23772=CARTESIAN_POINT('Ctrl Pts',(-41.5996821998361,37.2263796848018,38.2475145612583));
#23773=CARTESIAN_POINT('Ctrl Pts',(-41.6101104833444,37.2413900065276,38.2623712324232));
#23774=CARTESIAN_POINT('Ctrl Pts',(-41.0179887248003,36.6005789209292,37.4678003654629));
#23775=CARTESIAN_POINT('Ctrl Pts',(-41.0311471669881,36.6114222484506,37.485617698704));
#23776=CARTESIAN_POINT('Ctrl Pts',(-41.0442481894302,36.6224290791273,37.503377932541));
#23777=CARTESIAN_POINT('Ctrl Pts',(-41.0572903576435,36.6335982078395,37.5210791225655));
#23778=CARTESIAN_POINT('Ctrl Pts',(-41.0703209450169,36.6447574188839,37.538764594755));
#23779=CARTESIAN_POINT('Ctrl Pts',(-41.0832927827835,36.656078639948,37.5563911280262));
#23780=CARTESIAN_POINT('Ctrl Pts',(-41.096204453453,36.6675606339116,37.5739567962497));
#23781=CARTESIAN_POINT('Ctrl Pts',(-41.1091161241225,36.6790426278752,37.5915224644731));
#23782=CARTESIAN_POINT('Ctrl Pts',(-41.1219676276744,36.6906853947201,37.6090272676208));
#23783=CARTESIAN_POINT('Ctrl Pts',(-41.1347575597677,36.7024876621894,37.6264692928652));
#23784=CARTESIAN_POINT('Ctrl Pts',(-41.147547491861,36.7142899296587,37.6439113181096));
#23785=CARTESIAN_POINT('Ctrl Pts',(-41.1602758524755,36.7262516977336,37.6612905654229));
#23786=CARTESIAN_POINT('Ctrl Pts',(-41.1729412507266,36.7383716592988,37.6786051356975));
#23787=CARTESIAN_POINT('Ctrl Pts',(-41.1856066489777,36.7504916208638,37.6959197059722));
#23788=CARTESIAN_POINT('Ctrl Pts',(-41.1982090848453,36.7627697758997,37.7131695991807));
#23789=CARTESIAN_POINT('Ctrl Pts',(-41.2107471812052,36.775204782718,37.7303529303506));
#23790=CARTESIAN_POINT('Ctrl Pts',(-41.2232852775651,36.7876397895362,37.7475362615205));
#23791=CARTESIAN_POINT('Ctrl Pts',(-41.2357590343974,36.800231648117,37.7646530306244));
#23792=CARTESIAN_POINT('Ctrl Pts',(-41.2481670886393,36.8129789824919,37.781701367237));
#23793=CARTESIAN_POINT('Ctrl Pts',(-41.2605751428813,36.8257263168669,37.7987497038497));
#23794=CARTESIAN_POINT('Ctrl Pts',(-41.272917494513,36.8386291270158,37.8157296079438));
#23795=CARTESIAN_POINT('Ctrl Pts',(-41.285192794831,36.8516860029913,37.8326392240499));
#23796=CARTESIAN_POINT('Ctrl Pts',(-41.2974680951491,36.8647428789668,37.8495488401561));
#23797=CARTESIAN_POINT('Ctrl Pts',(-41.3096763440434,36.8779538206795,37.8663881681866));
#23798=CARTESIAN_POINT('Ctrl Pts',(-41.3218162076488,36.8913173846502,37.883155368157));
#23799=CARTESIAN_POINT('Ctrl Pts',(-41.3339560712541,36.9046809486209,37.8999225681274));
#23800=CARTESIAN_POINT('Ctrl Pts',(-41.3460275495374,36.9181971348206,37.9166176400022));
#23801=CARTESIAN_POINT('Ctrl Pts',(-41.358029323231,36.9318644661482,37.9332387593263));
#23802=CARTESIAN_POINT('Ctrl Pts',(-41.3700310969245,36.9455317974758,37.9498598786504));
#23803=CARTESIAN_POINT('Ctrl Pts',(-41.3819631660927,36.9593502739742,37.9664070454536));
#23804=CARTESIAN_POINT('Ctrl Pts',(-41.3938242268655,36.9733183856371,37.9828784515537));
#23805=CARTESIAN_POINT('Ctrl Pts',(-41.4056852876383,36.9872864973001,37.9993498576536));
#23806=CARTESIAN_POINT('Ctrl Pts',(-41.4174753399967,37.0014042441052,38.0157455030242));
#23807=CARTESIAN_POINT('Ctrl Pts',(-41.4291930955894,37.0156700833438,38.0320635960404));
#23808=CARTESIAN_POINT('Ctrl Pts',(-41.440910851182,37.0299359225824,38.0483816890565));
#23809=CARTESIAN_POINT('Ctrl Pts',(-41.4525563099903,37.0443498542317,38.0646222296922));
#23810=CARTESIAN_POINT('Ctrl Pts',(-41.4641281994632,37.0589103032173,38.0807834432716));
#23811=CARTESIAN_POINT('Ctrl Pts',(-41.4757000889362,37.073470752203,38.096944656851));
#23812=CARTESIAN_POINT('Ctrl Pts',(-41.4871984090552,37.0881777185019,38.1130265433482));
#23813=CARTESIAN_POINT('Ctrl Pts',(-41.498621903348,37.1030295950185,38.1290273454241));
#23814=CARTESIAN_POINT('Ctrl Pts',(-41.5100453976408,37.117881471535,38.1450281475001));
#23815=CARTESIAN_POINT('Ctrl Pts',(-41.5213940660891,37.1328782582455,38.1609478651294));
#23816=CARTESIAN_POINT('Ctrl Pts',(-41.5326666685735,37.1480183163847,38.1767847586936));
#23817=CARTESIAN_POINT('Ctrl Pts',(-41.5439392710579,37.1631583745239,38.1926216522579));
#23818=CARTESIAN_POINT('Ctrl Pts',(-41.5551358075605,37.1784417040676,38.2083757217319));
#23819=CARTESIAN_POINT('Ctrl Pts',(-41.566255054586,37.1938666349384,38.2240452455987));
#23820=CARTESIAN_POINT('Ctrl Pts',(-41.5773743016115,37.2092915658092,38.2397147694655));
#23821=CARTESIAN_POINT('Ctrl Pts',(-41.5884162591307,37.2248580979685,38.2552997476876));
#23822=CARTESIAN_POINT('Ctrl Pts',(-41.5993797205659,37.2405645304232,38.2707984772518));
#23823=CARTESIAN_POINT('Ctrl Pts',(-40.9769730429962,36.5766470661117,37.4405178991973));
#23824=CARTESIAN_POINT('Ctrl Pts',(-40.9908428778625,36.5877417466088,37.4591610102465));
#23825=CARTESIAN_POINT('Ctrl Pts',(-41.0046513375907,36.5990151832441,37.4777432926971));
#23826=CARTESIAN_POINT('Ctrl Pts',(-41.0183967838972,36.6104660355487,37.4962625408402));
#23827=CARTESIAN_POINT('Ctrl Pts',(-41.0321300248855,36.6219067200281,37.5147653447508));
#23828=CARTESIAN_POINT('Ctrl Pts',(-41.0458003644378,36.6335245053098,37.5332052263138));
#23829=CARTESIAN_POINT('Ctrl Pts',(-41.0594061838161,36.645318012843,37.5515800007768));
#23830=CARTESIAN_POINT('Ctrl Pts',(-41.0730120031943,36.6571115203761,37.5699547752398));
#23831=CARTESIAN_POINT('Ctrl Pts',(-41.0865533023731,36.6690807501385,37.5882644425688));
#23832=CARTESIAN_POINT('Ctrl Pts',(-41.1000284778738,36.6812242820791,37.6065068334128));
#23833=CARTESIAN_POINT('Ctrl Pts',(-41.1135036533746,36.6933678140196,37.6247492242568));
#23834=CARTESIAN_POINT('Ctrl Pts',(-41.1269127051723,36.7056856481155,37.6429243385819));
#23835=CARTESIAN_POINT('Ctrl Pts',(-41.1402540454255,36.7181763231499,37.6610300229497));
#23836=CARTESIAN_POINT('Ctrl Pts',(-41.1535953856787,36.7306669981843,37.6791357073173));
#23837=CARTESIAN_POINT('Ctrl Pts',(-41.1668690143625,36.7433305141338,37.6971719616938));
#23838=CARTESIAN_POINT('Ctrl Pts',(-41.1800733596466,36.7561653689606,37.7151366490602));
#23839=CARTESIAN_POINT('Ctrl Pts',(-41.1932777049307,36.7690002237873,37.7331013364267));
#23840=CARTESIAN_POINT('Ctrl Pts',(-41.2064127667905,36.7820064174673,37.7509944567495));
#23841=CARTESIAN_POINT('Ctrl Pts',(-41.2194769897764,36.7951824074959,37.7688138899326));
#23842=CARTESIAN_POINT('Ctrl Pts',(-41.2325412127622,36.8083583975245,37.7866333231157));
#23843=CARTESIAN_POINT('Ctrl Pts',(-41.24553459685,36.821704183877,37.8043790691258));
#23844=CARTESIAN_POINT('Ctrl Pts',(-41.2584556033373,36.8352181839453,37.8220490252892));
#23845=CARTESIAN_POINT('Ctrl Pts',(-41.2713766098246,36.8487321840136,37.8397189814527));
#23846=CARTESIAN_POINT('Ctrl Pts',(-41.2842252386047,36.8624143977111,37.857313147682));
#23847=CARTESIAN_POINT('Ctrl Pts',(-41.2969999682534,36.8762632028239,37.8748294393318));
#23848=CARTESIAN_POINT('Ctrl Pts',(-41.3097746979022,36.8901120079368,37.8923457309815));
#23849=CARTESIAN_POINT('Ctrl Pts',(-41.3224755283832,36.9041274044326,37.9097841480114));
#23850=CARTESIAN_POINT('Ctrl Pts',(-41.3351009554215,36.9183077305106,37.9271426239743));
#23851=CARTESIAN_POINT('Ctrl Pts',(-41.3477263824598,36.9324880565886,37.9445010999372));
#23852=CARTESIAN_POINT('Ctrl Pts',(-41.3602764061085,36.9468333122803,37.9617796348516));
#23853=CARTESIAN_POINT('Ctrl Pts',(-41.3727495400643,36.9613417969435,37.978976181265));
#23854=CARTESIAN_POINT('Ctrl Pts',(-41.3852226740201,36.9758502816067,37.9961727276784));
#23855=CARTESIAN_POINT('Ctrl Pts',(-41.3976189182597,36.9905219952142,38.0132872855588));
#23856=CARTESIAN_POINT('Ctrl Pts',(-41.4099368046517,37.0053551985681,38.0303178268316));
#23857=CARTESIAN_POINT('Ctrl Pts',(-41.4222546910436,37.0201884019219,38.0473483681044));
#23858=CARTESIAN_POINT('Ctrl Pts',(-41.4344942195651,37.0351830949946,38.0642948927377));
#23859=CARTESIAN_POINT('Ctrl Pts',(-41.4466539406019,37.0503375004424,38.0811553925125));
#23860=CARTESIAN_POINT('Ctrl Pts',(-41.4588136616388,37.0654919058901,38.0980158922873));
#23861=CARTESIAN_POINT('Ctrl Pts',(-41.4708935751684,37.0808060236847,38.1147903671719));
#23862=CARTESIAN_POINT('Ctrl Pts',(-41.4828922504357,37.0962780387556,38.1314768292758));
#23863=CARTESIAN_POINT('Ctrl Pts',(-41.4948909257029,37.1117500538266,38.1481632913796));
#23864=CARTESIAN_POINT('Ctrl Pts',(-41.5068083626853,37.1273799661451,38.1647617406715));
#23865=CARTESIAN_POINT('Ctrl Pts',(-41.5186431498235,37.1431659233413,38.1812702100575));
#23866=CARTESIAN_POINT('Ctrl Pts',(-41.5304779369617,37.1589518805375,38.1977786794435));
#23867=CARTESIAN_POINT('Ctrl Pts',(-41.5422300742335,37.1748938825821,38.2141971688928));
#23868=CARTESIAN_POINT('Ctrl Pts',(-41.5538981696076,37.1909900402423,38.2305237325717));
#23869=CARTESIAN_POINT('Ctrl Pts',(-41.5655662649816,37.2070861979025,38.2468502962505));
#23870=CARTESIAN_POINT('Ctrl Pts',(-41.5771503184253,37.2233365111352,38.2630849341168));
#23871=CARTESIAN_POINT('Ctrl Pts',(-41.5886489577874,37.2397390543188,38.2792257220803));
#23872=CARTESIAN_POINT('Ctrl Pts',(-40.9370413012329,36.5545511456659,37.4147676065073));
#23873=CARTESIAN_POINT('Ctrl Pts',(-40.9515996140237,36.5658534553905,37.434204060764));
#23874=CARTESIAN_POINT('Ctrl Pts',(-40.9660927536195,36.5773502054972,37.4535761511003));
#23875=CARTESIAN_POINT('Ctrl Pts',(-40.9805188577964,36.5890399153777,37.4728813871476));
#23876=CARTESIAN_POINT('Ctrl Pts',(-40.9949321522625,36.6007192453386,37.4921694810415));
#23877=CARTESIAN_POINT('Ctrl Pts',(-41.0092785302739,36.612591192521,37.5113908392785));
#23878=CARTESIAN_POINT('Ctrl Pts',(-41.0235561517129,36.6246542309846,37.530542995226));
#23879=CARTESIAN_POINT('Ctrl Pts',(-41.0378337731518,36.6367172694482,37.5496951511735));
#23880=CARTESIAN_POINT('Ctrl Pts',(-41.0520426379871,36.6489713991667,37.5687781047898));
#23881=CARTESIAN_POINT('Ctrl Pts',(-41.0661809237201,36.6614150453174,37.5877894071794));
#23882=CARTESIAN_POINT('Ctrl Pts',(-41.080319209453,36.6738586914682,37.6068007095689));
#23883=CARTESIAN_POINT('Ctrl Pts',(-41.094386916053,36.6864918540241,37.6257403606905));
#23884=CARTESIAN_POINT('Ctrl Pts',(-41.1083822391043,36.6993129096823,37.6446059300101));
#23885=CARTESIAN_POINT('Ctrl Pts',(-41.1223775621556,36.7121339653404,37.6634714993296));
#23886=CARTESIAN_POINT('Ctrl Pts',(-41.1363005016279,36.7251429140727,37.6822629868061));
#23887=CARTESIAN_POINT('Ctrl Pts',(-41.1501492716497,36.7383380845113,37.7009779808874));
#23888=CARTESIAN_POINT('Ctrl Pts',(-41.1639980416715,36.7515332549499,37.7196929749687));
#23889=CARTESIAN_POINT('Ctrl Pts',(-41.1777726422125,36.7649146470659,37.7383314756139));
#23890=CARTESIAN_POINT('Ctrl Pts',(-41.1914713063994,36.7784805418522,37.7568910908672));
#23891=CARTESIAN_POINT('Ctrl Pts',(-41.2051699705863,36.7920464366385,37.7754507061205));
#23892=CARTESIAN_POINT('Ctrl Pts',(-41.2187926983892,36.8057968340656,37.7939314359414));
#23893=CARTESIAN_POINT('Ctrl Pts',(-41.2323377423839,36.8197299679269,37.8123309085804));
#23894=CARTESIAN_POINT('Ctrl Pts',(-41.2458827863786,36.8336631017881,37.8307303812194));
#23895=CARTESIAN_POINT('Ctrl Pts',(-41.2593501465357,36.847778972053,37.8490485966365));
#23896=CARTESIAN_POINT('Ctrl Pts',(-41.2727380953247,36.8620757657659,37.8672832038934));
#23897=CARTESIAN_POINT('Ctrl Pts',(-41.2861260441138,36.8763725594786,37.8855178111503));
#23898=CARTESIAN_POINT('Ctrl Pts',(-41.2994345815056,36.8908502766081,37.9036688102071));
#23899=CARTESIAN_POINT('Ctrl Pts',(-41.312662000305,36.9055070579126,37.9217338715366));
#23900=CARTESIAN_POINT('Ctrl Pts',(-41.3258894191044,36.9201638392171,37.9397989328662));
#23901=CARTESIAN_POINT('Ctrl Pts',(-41.3390357192823,36.9349996846645,37.957778056429));
#23902=CARTESIAN_POINT('Ctrl Pts',(-41.3520992144129,36.9500126892013,37.9756689347026));
#23903=CARTESIAN_POINT('Ctrl Pts',(-41.3651627095435,36.965025693738,37.9935598129762));
#23904=CARTESIAN_POINT('Ctrl Pts',(-41.3781433995983,36.9802158573313,38.0113624459216));
#23905=CARTESIAN_POINT('Ctrl Pts',(-41.3910396193511,36.995581229602,38.0290745486096));
#23906=CARTESIAN_POINT('Ctrl Pts',(-41.4039358391038,37.0109466018728,38.0467866512976));
#23907=CARTESIAN_POINT('Ctrl Pts',(-41.4167475885263,37.0264871827876,38.0644082236895));
#23908=CARTESIAN_POINT('Ctrl Pts',(-41.4294732240162,37.0422009771393,38.0819370040326));
#23909=CARTESIAN_POINT('Ctrl Pts',(-41.4421988595062,37.0579147714911,38.0994657843757));
#23910=CARTESIAN_POINT('Ctrl Pts',(-41.4548383810359,37.0738017792454,38.1169017726317));
#23911=CARTESIAN_POINT('Ctrl Pts',(-41.4673901670459,37.0898599608768,38.1342427308005));
#23912=CARTESIAN_POINT('Ctrl Pts',(-41.479941953056,37.105918142508,38.1515836889694));
#23913=CARTESIAN_POINT('Ctrl Pts',(-41.492406003519,37.1221474979812,38.1688296170134));
#23914=CARTESIAN_POINT('Ctrl Pts',(-41.504780719332,37.1385459439719,38.1859783012565));
#23915=CARTESIAN_POINT('Ctrl Pts',(-41.517155435145,37.1549443899626,38.2031269854997));
#23916=CARTESIAN_POINT('Ctrl Pts',(-41.529440816281,37.171511926435,38.2201784259045));
#23917=CARTESIAN_POINT('Ctrl Pts',(-41.541635286501,37.1882464267978,38.2371304336835));
#23918=CARTESIAN_POINT('Ctrl Pts',(-41.553829756721,37.2049809271606,38.2540824414625));
#23919=CARTESIAN_POINT('Ctrl Pts',(-41.5659333159984,37.2218823913772,38.2709350165786));
#23920=CARTESIAN_POINT('Ctrl Pts',(-41.57794441136,37.2389486501317,38.2876859956913));
#23921=CARTESIAN_POINT('Ctrl Pts',(-40.898041328523,36.5339186748625,37.3902570496062));
#23922=CARTESIAN_POINT('Ctrl Pts',(-40.9132677638581,36.5453941770888,37.4104598746157));
#23923=CARTESIAN_POINT('Ctrl Pts',(-40.9284254085022,36.5570801166835,37.4305950141167));
#23924=CARTESIAN_POINT('Ctrl Pts',(-40.9435121571034,36.5689748704718,37.4506596713947));
#23925=CARTESIAN_POINT('Ctrl Pts',(-40.9585855093722,36.5808590622711,37.4707065121886));
#23926=CARTESIAN_POINT('Ctrl Pts',(-40.9735880914081,36.5929516975633,37.4906829958224));
#23927=CARTESIAN_POINT('Ctrl Pts',(-40.988517823087,36.6052510996916,37.5105863525352));
#23928=CARTESIAN_POINT('Ctrl Pts',(-41.0034475547659,36.61755050182,37.530489709248));
#23929=CARTESIAN_POINT('Ctrl Pts',(-41.0183044360495,36.630056670753,37.5503199389887));
#23930=CARTESIAN_POINT('Ctrl Pts',(-41.0330864070153,36.6427678724969,37.5700742922747));
#23931=CARTESIAN_POINT('Ctrl Pts',(-41.0478683779811,36.6554790742407,37.5898286455607));
#23932=CARTESIAN_POINT('Ctrl Pts',(-41.0625754385914,36.6683953087629,37.6095071223416));
#23933=CARTESIAN_POINT('Ctrl Pts',(-41.0772055496959,36.6815147852136,37.6291069941749));
#23934=CARTESIAN_POINT('Ctrl Pts',(-41.0918356608005,36.6946342616642,37.6487068660083));
#23935=CARTESIAN_POINT('Ctrl Pts',(-41.1063888223619,36.7079569800095,37.668228132844));
#23936=CARTESIAN_POINT('Ctrl Pts',(-41.120863016569,36.7214810930406,37.6876680880377));
#23937=CARTESIAN_POINT('Ctrl Pts',(-41.1353372107762,36.7350052060716,37.7071080432314));
#23938=CARTESIAN_POINT('Ctrl Pts',(-41.1497324375917,36.7487307137537,37.7264666867331));
#23939=CARTESIAN_POINT('Ctrl Pts',(-41.164046701102,36.7626557130303,37.7457413344461));
#23940=CARTESIAN_POINT('Ctrl Pts',(-41.1783609646123,36.7765807123069,37.7650159821591));
#23941=CARTESIAN_POINT('Ctrl Pts',(-41.1925942647807,36.7907052031424,37.7842066340339));
#23942=CARTESIAN_POINT('Ctrl Pts',(-41.2067446281447,36.805027227161,37.8033106292661));
#23943=CARTESIAN_POINT('Ctrl Pts',(-41.2208949915087,36.8193492511795,37.8224146244984));
#23944=CARTESIAN_POINT('Ctrl Pts',(-41.2349624180324,36.8338688083445,37.8414319630391));
#23945=CARTESIAN_POINT('Ctrl Pts',(-41.2489449572515,36.8485838855035,37.8603600081137));
#23946=CARTESIAN_POINT('Ctrl Pts',(-41.2629274964706,36.8632989626625,37.8792880531883));
#23947=CARTESIAN_POINT('Ctrl Pts',(-41.2768251483493,36.8782095597778,37.8981268047483));
#23948=CARTESIAN_POINT('Ctrl Pts',(-41.2906359859636,36.8933136094794,37.9168736507806));
#23949=CARTESIAN_POINT('Ctrl Pts',(-41.3044468235779,36.9084176591809,37.935620496813));
#23950=CARTESIAN_POINT('Ctrl Pts',(-41.3181708468922,36.9237151614297,37.9542754372696));
#23951=CARTESIAN_POINT('Ctrl Pts',(-41.3318061530559,36.939203995211,37.9728358856229));
#23952=CARTESIAN_POINT('Ctrl Pts',(-41.3454414592196,36.9546928289921,37.9913963339763));
#23953=CARTESIAN_POINT('Ctrl Pts',(-41.3589880481978,36.9703729942658,38.0098622901787));
#23954=CARTESIAN_POINT('Ctrl Pts',(-41.3724440417414,36.9862423169603,38.0282311939057));
#23955=CARTESIAN_POINT('Ctrl Pts',(-41.385900035285,37.0021116396548,38.0466000976326));
#23956=CARTESIAN_POINT('Ctrl Pts',(-41.3992654333594,37.0181701197294,38.0648719488369));
#23957=CARTESIAN_POINT('Ctrl Pts',(-41.4125383828378,37.0344155306586,38.0830442141068));
#23958=CARTESIAN_POINT('Ctrl Pts',(-41.4258113323163,37.0506609415878,38.1012164793766));
#23959=CARTESIAN_POINT('Ctrl Pts',(-41.4389918331648,37.0670932833299,38.1192891586655));
#23960=CARTESIAN_POINT('Ctrl Pts',(-41.4520780578928,37.0837102775231,38.137259746177));
#23961=CARTESIAN_POINT('Ctrl Pts',(-41.4651642826207,37.1003272717164,38.1552303336884));
#23962=CARTESIAN_POINT('Ctrl Pts',(-41.4781562311946,37.1171289183182,38.1730988293764));
#23963=CARTESIAN_POINT('Ctrl Pts',(-41.4910521022666,37.1341128877621,38.1908627557548));
#23964=CARTESIAN_POINT('Ctrl Pts',(-41.5039479733387,37.151096857206,38.2086266821332));
#23965=CARTESIAN_POINT('Ctrl Pts',(-41.516747766876,37.1682631494485,38.2262860391564));
#23966=CARTESIAN_POINT('Ctrl Pts',(-41.5294497081733,37.1856093843648,38.2438383783356));
#23967=CARTESIAN_POINT('Ctrl Pts',(-41.5421516494707,37.2029556192811,38.2613907175148));
#23968=CARTESIAN_POINT('Ctrl Pts',(-41.5547557384956,37.2204817968266,38.2788360388052));
#23969=CARTESIAN_POINT('Ctrl Pts',(-41.5672602276774,37.2381854869781,38.2961719233939));
#23970=CARTESIAN_POINT('Ctrl Pts',(-40.8590413558131,36.513286204059,37.3657464927051));
#23971=CARTESIAN_POINT('Ctrl Pts',(-40.8749359136926,36.5249348987871,37.3867156884675));
#23972=CARTESIAN_POINT('Ctrl Pts',(-40.8907580633849,36.5368100278699,37.407613877133));
#23973=CARTESIAN_POINT('Ctrl Pts',(-40.9065054564103,36.548909825566,37.4284379556418));
#23974=CARTESIAN_POINT('Ctrl Pts',(-40.9222388664818,36.5609988792036,37.4492435433357));
#23975=CARTESIAN_POINT('Ctrl Pts',(-40.9378976525422,36.5733122026056,37.4699751523663));
#23976=CARTESIAN_POINT('Ctrl Pts',(-40.9534794944611,36.5858479683988,37.4906297098443));
#23977=CARTESIAN_POINT('Ctrl Pts',(-40.9690613363799,36.5983837341919,37.5112842673223));
#23978=CARTESIAN_POINT('Ctrl Pts',(-40.9845662341119,36.6111419423394,37.5318617731876));
#23979=CARTESIAN_POINT('Ctrl Pts',(-40.9999918903106,36.6241206996763,37.5523591773701));
#23980=CARTESIAN_POINT('Ctrl Pts',(-41.0154175465092,36.6370994570133,37.5728565815525));
#23981=CARTESIAN_POINT('Ctrl Pts',(-41.0307639611298,36.6502987635018,37.5932738839926));
#23982=CARTESIAN_POINT('Ctrl Pts',(-41.0460288602876,36.6637166607449,37.6136080583398));
#23983=CARTESIAN_POINT('Ctrl Pts',(-41.0612937594454,36.677134557988,37.6339422326869));
#23984=CARTESIAN_POINT('Ctrl Pts',(-41.076477143096,36.6907710459463,37.654193278882));
#23985=CARTESIAN_POINT('Ctrl Pts',(-41.0915767614884,36.7046241015698,37.674358195188));
#23986=CARTESIAN_POINT('Ctrl Pts',(-41.1066763798808,36.7184771571934,37.6945231114941));
#23987=CARTESIAN_POINT('Ctrl Pts',(-41.121692232971,36.7325467804415,37.7146018978523));
#23988=CARTESIAN_POINT('Ctrl Pts',(-41.1366220958047,36.7468308842084,37.734591578025));
#23989=CARTESIAN_POINT('Ctrl Pts',(-41.1515519586384,36.7611149879753,37.7545812581977));
#23990=CARTESIAN_POINT('Ctrl Pts',(-41.1663958311721,36.7756135722191,37.7744818321265));
#23991=CARTESIAN_POINT('Ctrl Pts',(-41.1811515139055,36.7903244863951,37.7942903499519));
#23992=CARTESIAN_POINT('Ctrl Pts',(-41.1959071966389,36.8050354005709,37.8140988677773));
#23993=CARTESIAN_POINT('Ctrl Pts',(-41.210574689529,36.8199586446359,37.8338153294417));
#23994=CARTESIAN_POINT('Ctrl Pts',(-41.2251518191782,36.8350920052412,37.853436812334));
#23995=CARTESIAN_POINT('Ctrl Pts',(-41.2397289488273,36.8502253658463,37.8730582952263));
#23996=CARTESIAN_POINT('Ctrl Pts',(-41.254215715193,36.8655688429475,37.8925847992895));
#23997=CARTESIAN_POINT('Ctrl Pts',(-41.2686099716222,36.8811201610461,37.9120134300246));
#23998=CARTESIAN_POINT('Ctrl Pts',(-41.2830042280514,36.8966714791447,37.9314420607598));
#23999=CARTESIAN_POINT('Ctrl Pts',(-41.2973059745021,36.912430638195,37.9507728181102));
#24000=CARTESIAN_POINT('Ctrl Pts',(-41.3115130916989,36.9283953012207,37.9700028365432));
#24001=CARTESIAN_POINT('Ctrl Pts',(-41.3257202088957,36.9443599642462,37.9892328549763));
#24002=CARTESIAN_POINT('Ctrl Pts',(-41.3398326967973,36.9605301312003,38.0083621344359));
#24003=CARTESIAN_POINT('Ctrl Pts',(-41.3538484641317,36.9769034043186,38.0273878392017));
#24004=CARTESIAN_POINT('Ctrl Pts',(-41.3678642314661,36.9932766774368,38.0464135439676));
#24005=CARTESIAN_POINT('Ctrl Pts',(-41.3817832781924,37.0098530566712,38.0653356739843));
#24006=CARTESIAN_POINT('Ctrl Pts',(-41.3956035416594,37.0266300841779,38.0841514241809));
#24007=CARTESIAN_POINT('Ctrl Pts',(-41.4094238051265,37.0434071116845,38.1029671743776));
#24008=CARTESIAN_POINT('Ctrl Pts',(-41.4231452852938,37.0603847874144,38.1216765446994));
#24009=CARTESIAN_POINT('Ctrl Pts',(-41.4367659487396,37.0775605941696,38.1402767615534));
#24010=CARTESIAN_POINT('Ctrl Pts',(-41.4503866121855,37.0947364009248,38.1588769784074));
#24011=CARTESIAN_POINT('Ctrl Pts',(-41.4639064588701,37.1121103386552,38.1773680417394));
#24012=CARTESIAN_POINT('Ctrl Pts',(-41.4773234852013,37.1296798315523,38.195747210253));
#24013=CARTESIAN_POINT('Ctrl Pts',(-41.4907405115324,37.1472493244494,38.2141263787666));
#24014=CARTESIAN_POINT('Ctrl Pts',(-41.504054717471,37.165014372462,38.2323936524082));
#24015=CARTESIAN_POINT('Ctrl Pts',(-41.5172641298457,37.1829723419318,38.2505463229878));
#24016=CARTESIAN_POINT('Ctrl Pts',(-41.5304735422203,37.2009303114016,38.2686989935672));
#24017=CARTESIAN_POINT('Ctrl Pts',(-41.5435781609927,37.2190812022761,38.2867370610317));
#24018=CARTESIAN_POINT('Ctrl Pts',(-41.5565760439949,37.2374223238246,38.3046578510965));
#24019=CARTESIAN_POINT('Ctrl Pts',(-40.8209716822033,36.4941186642374,37.3424762704269));
#24020=CARTESIAN_POINT('Ctrl Pts',(-40.8375140519548,36.5059060599091,37.3641848666864));
#24021=CARTESIAN_POINT('Ctrl Pts',(-40.8539805753213,36.5179362010818,37.3858193469145));
#24022=CARTESIAN_POINT('Ctrl Pts',(-40.8703686424312,36.5302071774958,37.4073762805876));
#24023=CARTESIAN_POINT('Ctrl Pts',(-40.8867421576984,36.5424672578523,37.4289140727044));
#24024=CARTESIAN_POINT('Ctrl Pts',(-40.9030373558039,36.5549677458436,37.4503744557762));
#24025=CARTESIAN_POINT('Ctrl Pts',(-40.9192516575975,36.5677066598323,37.4717540322971));
#24026=CARTESIAN_POINT('Ctrl Pts',(-40.9354659593912,36.5804455738209,37.4931336088181));
#24027=CARTESIAN_POINT('Ctrl Pts',(-40.9515993648368,36.593422913768,37.5144323787275));
#24028=CARTESIAN_POINT('Ctrl Pts',(-40.9676493211198,36.6066366231236,37.5356469705377));
#24029=CARTESIAN_POINT('Ctrl Pts',(-40.9836992774029,36.6198503324791,37.5568615623479));
#24030=CARTESIAN_POINT('Ctrl Pts',(-40.9996657844525,36.6333004111949,37.5779919759778));
#24031=CARTESIAN_POINT('Ctrl Pts',(-41.0155463151547,36.6469847276582,37.5990348661468));
#24032=CARTESIAN_POINT('Ctrl Pts',(-41.031426845857,36.6606690441215,37.6200777563158));
#24033=CARTESIAN_POINT('Ctrl Pts',(-41.0472214001766,36.6745875982916,37.6410331229643));
#24034=CARTESIAN_POINT('Ctrl Pts',(-41.0629274788306,36.6887381849399,37.6618976488843));
#24035=CARTESIAN_POINT('Ctrl Pts',(-41.0786335574846,36.7028887715881,37.6827621748045));
#24036=CARTESIAN_POINT('Ctrl Pts',(-41.0942511602649,36.7172713905735,37.7035358598319));
#24037=CARTESIAN_POINT('Ctrl Pts',(-41.1097778155592,36.7318837631807,37.7242154153001));
#24038=CARTESIAN_POINT('Ctrl Pts',(-41.1253044708535,36.7464961357878,37.7448949707684));
#24039=CARTESIAN_POINT('Ctrl Pts',(-41.1407401786102,36.761338261968,37.7654803966087));
#24040=CARTESIAN_POINT('Ctrl Pts',(-41.1560824959735,36.7764077904247,37.7859684339199));
#24041=CARTESIAN_POINT('Ctrl Pts',(-41.1714248133369,36.7914773188815,37.8064564712311));
#24042=CARTESIAN_POINT('Ctrl Pts',(-41.186673740424,36.806774249681,37.8268471200493));
#24043=CARTESIAN_POINT('Ctrl Pts',(-41.2018268635633,36.8222961594514,37.8471371520539));
#24044=CARTESIAN_POINT('Ctrl Pts',(-41.2169799867026,36.8378180692218,37.8674271840586));
#24045=CARTESIAN_POINT('Ctrl Pts',(-41.2320373058687,36.8535649579224,37.8876165991963));
#24046=CARTESIAN_POINT('Ctrl Pts',(-41.2469964383245,36.8695343315615,37.9077022013597));
#24047=CARTESIAN_POINT('Ctrl Pts',(-41.2619555707802,36.8855037052005,37.9277878035232));
#24048=CARTESIAN_POINT('Ctrl Pts',(-41.2768165163203,36.9016955636138,37.9477695925484));
#24049=CARTESIAN_POINT('Ctrl Pts',(-41.2915769229406,36.918107342302,37.9676444049552));
#24050=CARTESIAN_POINT('Ctrl Pts',(-41.3063373295609,36.9345191209902,37.9875192173619));
#24051=CARTESIAN_POINT('Ctrl Pts',(-41.3209971972124,36.9511508198986,38.0072870530841));
#24052=CARTESIAN_POINT('Ctrl Pts',(-41.3355542056702,36.9679998050485,38.0269447824567));
#24053=CARTESIAN_POINT('Ctrl Pts',(-41.3501112141281,36.9848487901984,38.0466025118293));
#24054=CARTESIAN_POINT('Ctrl Pts',(-41.3645653633439,37.0019150615336,38.0661501347871));
#24055=CARTESIAN_POINT('Ctrl Pts',(-41.3789143656034,37.0191959164268,38.0855845564669));
#24056=CARTESIAN_POINT('Ctrl Pts',(-41.3932633678628,37.0364767713199,38.1050189781468));
#24057=CARTESIAN_POINT('Ctrl Pts',(-41.4075072231182,37.0539722097134,38.1243401984841));
#24058=CARTESIAN_POINT('Ctrl Pts',(-41.4216436768867,37.0716794611833,38.1435451583937));
#24059=CARTESIAN_POINT('Ctrl Pts',(-41.4357801306552,37.0893867126534,38.1627501183033));
#24060=CARTESIAN_POINT('Ctrl Pts',(-41.4498091828898,37.1073057771408,38.1818388177213));
#24061=CARTESIAN_POINT('Ctrl Pts',(-41.4637286130497,37.1254338172992,38.2008082343046));
#24062=CARTESIAN_POINT('Ctrl Pts',(-41.4776480432095,37.1435618574576,38.2197776508878));
#24063=CARTESIAN_POINT('Ctrl Pts',(-41.4914578512484,37.1618988732265,38.2386277845733));
#24064=CARTESIAN_POINT('Ctrl Pts',(-41.5051558512673,37.1804419612312,38.2573556507129));
#24065=CARTESIAN_POINT('Ctrl Pts',(-41.5188538512862,37.1989850492358,38.2760835168526));
#24066=CARTESIAN_POINT('Ctrl Pts',(-41.5324400432657,37.2177342094461,38.2946891154127));
#24067=CARTESIAN_POINT('Ctrl Pts',(-41.5459122765801,37.2366864733069,38.3131695003217));
#24068=CARTESIAN_POINT('Ctrl Pts',(-40.783693232143,36.4761376056301,37.3202208879071));
#24069=CARTESIAN_POINT('Ctrl Pts',(-40.8008656922496,36.4880359432873,37.3426462956984));
#24070=CARTESIAN_POINT('Ctrl Pts',(-40.817959055311,36.5001935767271,37.3649946966318));
#24071=CARTESIAN_POINT('Ctrl Pts',(-40.834970431829,36.5126084506244,37.3872623124709));
#24072=CARTESIAN_POINT('Ctrl Pts',(-40.8519667030344,36.5250123006901,37.4095101557009));
#24073=CARTESIAN_POINT('Ctrl Pts',(-40.8688811330549,36.5376729344845,37.4316773570879));
#24074=CARTESIAN_POINT('Ctrl Pts',(-40.8857108667677,36.5505882150004,37.4537601751103));
#24075=CARTESIAN_POINT('Ctrl Pts',(-40.9025406004804,36.5635034955164,37.4758429931327));
#24076=CARTESIAN_POINT('Ctrl Pts',(-40.9192856378381,36.5766734227079,37.4978414277164));
#24077=CARTESIAN_POINT('Ctrl Pts',(-40.9359431530081,36.5900957739832,37.5197517662424));
#24078=CARTESIAN_POINT('Ctrl Pts',(-40.9526006681781,36.6035181252586,37.5416621047685));
#24079=CARTESIAN_POINT('Ctrl Pts',(-40.9691706610809,36.6171929005631,37.5634843471441));
#24080=CARTESIAN_POINT('Ctrl Pts',(-40.9856503347759,36.6311177917365,37.5852148100976));
#24081=CARTESIAN_POINT('Ctrl Pts',(-41.0021300084708,36.6450426829098,37.6069452730511));
#24082=CARTESIAN_POINT('Ctrl Pts',(-41.0185193629119,36.6592176899033,37.6285839565095));
#24083=CARTESIAN_POINT('Ctrl Pts',(-41.0348156322482,36.6736404204794,37.6501272085428));
#24084=CARTESIAN_POINT('Ctrl Pts',(-41.0511119015846,36.6880631510554,37.6716704605762));
#24085=CARTESIAN_POINT('Ctrl Pts',(-41.0673150856079,36.7027336050728,37.6931182810147));
#24086=CARTESIAN_POINT('Ctrl Pts',(-41.0834224495998,36.717649306502,37.7144670499681));
#24087=CARTESIAN_POINT('Ctrl Pts',(-41.0995298135917,36.7325650079314,37.7358158189215));
#24088=CARTESIAN_POINT('Ctrl Pts',(-41.1155413574911,36.7477259567159,37.7570655363088));
#24089=CARTESIAN_POINT('Ctrl Pts',(-41.1314543789239,36.7631295940424,37.7782126156749));
#24090=CARTESIAN_POINT('Ctrl Pts',(-41.1473674003568,36.7785332313689,37.799359695041));
#24091=CARTESIAN_POINT('Ctrl Pts',(-41.1631818994208,36.7941795572869,37.8204041364024));
#24092=CARTESIAN_POINT('Ctrl Pts',(-41.1788952066766,36.8100659308439,37.841342387753));
#24093=CARTESIAN_POINT('Ctrl Pts',(-41.1946085139324,36.8259523044009,37.8622806391035));
#24094=CARTESIAN_POINT('Ctrl Pts',(-41.2102206293435,36.8420787255466,37.8831127003765));
#24095=CARTESIAN_POINT('Ctrl Pts',(-41.2257289182373,36.8584424727222,37.9038350557851));
#24096=CARTESIAN_POINT('Ctrl Pts',(-41.2412372071311,36.8748062198979,37.9245574111936));
#24097=CARTESIAN_POINT('Ctrl Pts',(-41.2566416693023,36.8914072929382,37.9451700605687));
#24098=CARTESIAN_POINT('Ctrl Pts',(-41.2719397048379,36.9082428899705,37.9656695249773));
#24099=CARTESIAN_POINT('Ctrl Pts',(-41.2872377403735,36.9250784870027,37.9861689893859));
#24100=CARTESIAN_POINT('Ctrl Pts',(-41.3024293492156,36.942148607963,38.0065552687502));
#24101=CARTESIAN_POINT('Ctrl Pts',(-41.3175119673761,36.9594503718142,38.0268249223433));
#24102=CARTESIAN_POINT('Ctrl Pts',(-41.3325945855365,36.9767521356655,38.0470945759364));
#24103=CARTESIAN_POINT('Ctrl Pts',(-41.347568212958,36.9942855423421,38.0672476036812));
#24104=CARTESIAN_POINT('Ctrl Pts',(-41.3624303224426,37.0120476326152,38.0872806042184));
#24105=CARTESIAN_POINT('Ctrl Pts',(-41.3772924319271,37.0298097228883,38.1073136047554));
#24106=CARTESIAN_POINT('Ctrl Pts',(-41.3920430234184,37.0478004966904,38.1272265780087));
#24107=CARTESIAN_POINT('Ctrl Pts',(-41.4066796073615,37.0660169176001,38.1470161631342));
#24108=CARTESIAN_POINT('Ctrl Pts',(-41.4213161913047,37.0842333385096,38.1668057482597));
#24109=CARTESIAN_POINT('Ctrl Pts',(-41.4358387676443,37.1026754064574,38.1864719451823));
#24110=CARTESIAN_POINT('Ctrl Pts',(-41.4502448853092,37.1213400088539,38.2060114347081));
#24111=CARTESIAN_POINT('Ctrl Pts',(-41.4646510029741,37.1400046112504,38.2255509242339));
#24112=CARTESIAN_POINT('Ctrl Pts',(-41.4789406619095,37.1588917480246,38.2449637062886));
#24113=CARTESIAN_POINT('Ctrl Pts',(-41.4931114503555,37.1779982314699,38.264246504449));
#24114=CARTESIAN_POINT('Ctrl Pts',(-41.5072822388015,37.1971047149152,38.2835293026094));
#24115=CARTESIAN_POINT('Ctrl Pts',(-41.5213341567292,37.2164305449896,38.3026821168296));
#24116=CARTESIAN_POINT('Ctrl Pts',(-41.5352648324485,37.23597245988,38.3217017145054));
#24117=CARTESIAN_POINT('Ctrl Pts',(-40.7464147820825,36.4581565470228,37.2979655053874));
#24118=CARTESIAN_POINT('Ctrl Pts',(-40.7642173325444,36.4701658266656,37.3211077247104));
#24119=CARTESIAN_POINT('Ctrl Pts',(-40.7819375353008,36.4824509523723,37.3441700463492));
#24120=CARTESIAN_POINT('Ctrl Pts',(-40.7995722212268,36.4950097237531,37.3671483443542));
#24121=CARTESIAN_POINT('Ctrl Pts',(-40.8171912483704,36.5075573435279,37.3901062386973));
#24122=CARTESIAN_POINT('Ctrl Pts',(-40.834724910306,36.5203781231252,37.4129802583996));
#24123=CARTESIAN_POINT('Ctrl Pts',(-40.8521700759379,36.5334697701685,37.4357663179235));
#24124=CARTESIAN_POINT('Ctrl Pts',(-40.8696152415697,36.5465614172118,37.4585523774474));
#24125=CARTESIAN_POINT('Ctrl Pts',(-40.8869719108393,36.5599239316479,37.4812504767052));
#24126=CARTESIAN_POINT('Ctrl Pts',(-40.9042369848963,36.573554924843,37.5038565619471));
#24127=CARTESIAN_POINT('Ctrl Pts',(-40.9215020589534,36.5871859180381,37.526462647189));
#24128=CARTESIAN_POINT('Ctrl Pts',(-40.9386755377092,36.6010853899314,37.5489767183103));
#24129=CARTESIAN_POINT('Ctrl Pts',(-40.955754354397,36.6152508558148,37.5713947540483));
#24130=CARTESIAN_POINT('Ctrl Pts',(-40.9728331710848,36.629416321698,37.5938127897864));
#24131=CARTESIAN_POINT('Ctrl Pts',(-40.9898173256472,36.643847781515,37.6161347900547));
#24132=CARTESIAN_POINT('Ctrl Pts',(-41.0067037856659,36.6585426560188,37.6383567682013));
#24133=CARTESIAN_POINT('Ctrl Pts',(-41.0235902456846,36.6732375305227,37.6605787463478));
#24134=CARTESIAN_POINT('Ctrl Pts',(-41.0403790109508,36.6881958195721,37.6827007021974));
#24135=CARTESIAN_POINT('Ctrl Pts',(-41.0570670836403,36.7034148498235,37.7047186846361));
#24136=CARTESIAN_POINT('Ctrl Pts',(-41.0737551563299,36.7186338800749,37.7267366670747));
#24137=CARTESIAN_POINT('Ctrl Pts',(-41.0903425363719,36.7341136514639,37.748650676009));
#24138=CARTESIAN_POINT('Ctrl Pts',(-41.1068262618743,36.7498513976601,37.77045679743));
#24139=CARTESIAN_POINT('Ctrl Pts',(-41.1233099873767,36.7655891438563,37.792262918851));
#24140=CARTESIAN_POINT('Ctrl Pts',(-41.1396900584178,36.7815848648927,37.8139611527556));
#24141=CARTESIAN_POINT('Ctrl Pts',(-41.15596354979,36.7978357022364,37.835547623452));
#24142=CARTESIAN_POINT('Ctrl Pts',(-41.1722370411622,36.8140865395801,37.8571340941484));
#24143=CARTESIAN_POINT('Ctrl Pts',(-41.1884039528183,36.8305924931708,37.8786088015567));
#24144=CARTESIAN_POINT('Ctrl Pts',(-41.2044613981502,36.847350613883,37.8999679102104));
#24145=CARTESIAN_POINT('Ctrl Pts',(-41.220518843482,36.8641087345953,37.9213270188641));
#24146=CARTESIAN_POINT('Ctrl Pts',(-41.2364668222842,36.8811190222625,37.942570528589));
#24147=CARTESIAN_POINT('Ctrl Pts',(-41.2523024867352,36.8983784376388,37.9636946449994));
#24148=CARTESIAN_POINT('Ctrl Pts',(-41.2681381511862,36.9156378530152,37.9848187614099));
#24149=CARTESIAN_POINT('Ctrl Pts',(-41.2838615012189,36.9331463960273,38.0058234844164));
#24150=CARTESIAN_POINT('Ctrl Pts',(-41.2994697290819,36.9509009385799,38.0267050622299));
#24151=CARTESIAN_POINT('Ctrl Pts',(-41.3150779569449,36.9686554811326,38.0475866400434));
#24152=CARTESIAN_POINT('Ctrl Pts',(-41.330571062572,36.9866560231506,38.0683450725754));
#24153=CARTESIAN_POINT('Ctrl Pts',(-41.3459462792817,37.0048993488036,38.0889766519698));
#24154=CARTESIAN_POINT('Ctrl Pts',(-41.3613214959914,37.0231426744568,38.1096082313641));
#24155=CARTESIAN_POINT('Ctrl Pts',(-41.3765788237185,37.0416287836675,38.1301129575333));
#24156=CARTESIAN_POINT('Ctrl Pts',(-41.3917155378364,37.0603543740167,38.1504871678747));
#24157=CARTESIAN_POINT('Ctrl Pts',(-41.4068522519543,37.0790799643659,38.1708613782161));
#24158=CARTESIAN_POINT('Ctrl Pts',(-41.4218683523989,37.098045035774,38.1911050726434));
#24159=CARTESIAN_POINT('Ctrl Pts',(-41.4367611575687,37.1172462004086,38.2112146351116));
#24160=CARTESIAN_POINT('Ctrl Pts',(-41.4516539627386,37.1364473650431,38.2313241975799));
#24161=CARTESIAN_POINT('Ctrl Pts',(-41.4664234725707,37.1558846228228,38.251299628004));
#24162=CARTESIAN_POINT('Ctrl Pts',(-41.4810670494437,37.1755545017087,38.2711373581851));
#24163=CARTESIAN_POINT('Ctrl Pts',(-41.4957106263168,37.1952243805947,38.2909750883661));
#24164=CARTESIAN_POINT('Ctrl Pts',(-41.5102282701928,37.2151268805331,38.3106751182465));
#24165=CARTESIAN_POINT('Ctrl Pts',(-41.5246173883169,37.235258446453,38.330233928689));
#24166=CARTESIAN_POINT('Ctrl Pts',(-40.709927446472,36.4413634896317,37.2767259574961));
#24167=CARTESIAN_POINT('Ctrl Pts',(-40.7283423747484,36.4534559082533,37.3005623856167));
#24168=CARTESIAN_POINT('Ctrl Pts',(-40.7466718917616,36.4658409631829,37.324316242929));
#24169=CARTESIAN_POINT('Ctrl Pts',(-40.7649125306715,36.4785163085151,37.3479830356273));
#24170=CARTESIAN_POINT('Ctrl Pts',(-40.7831369727409,36.4911803987291,37.3716288133124));
#24171=CARTESIAN_POINT('Ctrl Pts',(-40.8012726943898,36.5041342639858,37.3951876808215));
#24172=CARTESIAN_POINT('Ctrl Pts',(-40.8193162714995,36.5173754553539,37.418655189126));
#24173=CARTESIAN_POINT('Ctrl Pts',(-40.8373598486091,36.530616646722,37.4421226974304));
#24174=CARTESIAN_POINT('Ctrl Pts',(-40.855311281094,36.5441451641385,37.465498846419));
#24175=CARTESIAN_POINT('Ctrl Pts',(-40.8731671796206,36.5579584503267,37.4887792215566));
#24176=CARTESIAN_POINT('Ctrl Pts',(-40.8910230781472,36.5717717365149,37.5120595966941));
#24177=CARTESIAN_POINT('Ctrl Pts',(-40.9087834426309,36.585869791409,37.5352441978702));
#24178=CARTESIAN_POINT('Ctrl Pts',(-40.9264449197973,36.6002499503495,37.5583286467043));
#24179=CARTESIAN_POINT('Ctrl Pts',(-40.9441063969636,36.6146301092899,37.5814130955383));
#24180=CARTESIAN_POINT('Ctrl Pts',(-40.961668986729,36.6292923722084,37.6043973919208));
#24181=CARTESIAN_POINT('Ctrl Pts',(-40.9791293731422,36.6442339680676,37.627277195275));
#24182=CARTESIAN_POINT('Ctrl Pts',(-40.9965897595554,36.6591755639269,37.6501569986292));
#24183=CARTESIAN_POINT('Ctrl Pts',(-41.0139479425334,36.674396492656,37.6729323088466));
#24184=CARTESIAN_POINT('Ctrl Pts',(-41.0312006446953,36.6898938778835,37.695598824788));
#24185=CARTESIAN_POINT('Ctrl Pts',(-41.0484533468572,36.7053912631111,37.7182653407295));
#24186=CARTESIAN_POINT('Ctrl Pts',(-41.0656005681211,36.7211651047637,37.7408230622875));
#24187=CARTESIAN_POINT('Ctrl Pts',(-41.0826390709103,36.7372124222201,37.7632677293804));
#24188=CARTESIAN_POINT('Ctrl Pts',(-41.0996775736996,36.7532597396764,37.7857123964734));
#24189=CARTESIAN_POINT('Ctrl Pts',(-41.1166073579336,36.7695805328605,37.8080440089949));
#24190=CARTESIAN_POINT('Ctrl Pts',(-41.1334252270582,36.7861717180241,37.8302583495245));
#24191=CARTESIAN_POINT('Ctrl Pts',(-41.1502430961829,36.8027629031877,37.852472690054));
#24192=CARTESIAN_POINT('Ctrl Pts',(-41.1669490501186,36.819624480252,37.8745697584863));
#24193=CARTESIAN_POINT('Ctrl Pts',(-41.1835399345382,36.8367532635039,37.8965453816507));
#24194=CARTESIAN_POINT('Ctrl Pts',(-41.2001308189578,36.8538820467558,37.9185210048151));
#24195=CARTESIAN_POINT('Ctrl Pts',(-41.2166066337826,36.871278036114,37.9403751826072));
#24196=CARTESIAN_POINT('Ctrl Pts',(-41.2329642680989,36.8889379451001,37.962103787677));
#24197=CARTESIAN_POINT('Ctrl Pts',(-41.2493219024152,36.9065978540862,37.9838323927467));
#24198=CARTESIAN_POINT('Ctrl Pts',(-41.2655613561456,36.9245216826165,38.005435424991));
#24199=CARTESIAN_POINT('Ctrl Pts',(-41.2816795629613,36.9427060446854,38.0269088044348));
#24200=CARTESIAN_POINT('Ctrl Pts',(-41.297797769777,36.9608904067542,38.0483821838785));
#24201=CARTESIAN_POINT('Ctrl Pts',(-41.3137947296017,36.9793353022755,38.0697259104199));
#24202=CARTESIAN_POINT('Ctrl Pts',(-41.3296674218458,36.998037246992,38.0909359529947));
#24203=CARTESIAN_POINT('Ctrl Pts',(-41.3455401140899,37.0167391917085,38.1121459955696));
#24204=CARTESIAN_POINT('Ctrl Pts',(-41.3612885386784,37.0356981855315,38.1332223540776));
#24205=CARTESIAN_POINT('Ctrl Pts',(-41.3769097218979,37.0549106472643,38.1541610478837));
#24206=CARTESIAN_POINT('Ctrl Pts',(-41.3925309051175,37.0741231089972,38.1750997416898));
#24207=CARTESIAN_POINT('Ctrl Pts',(-41.4080248468942,37.0935890385488,38.1959007706948));
#24208=CARTESIAN_POINT('Ctrl Pts',(-41.4233886215108,37.1133047591318,38.2165602061919));
#24209=CARTESIAN_POINT('Ctrl Pts',(-41.4387523961274,37.1330204797148,38.2372196416891));
#24210=CARTESIAN_POINT('Ctrl Pts',(-41.4539860035111,37.1529859912358,38.2577374835804));
#24211=CARTESIAN_POINT('Ctrl Pts',(-41.4690865670421,37.1731975227013,38.2781098565668));
#24212=CARTESIAN_POINT('Ctrl Pts',(-41.4841871305731,37.1934090541668,38.2984822295532));
#24213=CARTESIAN_POINT('Ctrl Pts',(-41.4991546501799,37.213866605481,38.318709133538));
#24214=CARTESIAN_POINT('Ctrl Pts',(-41.5139862994228,37.2345663128649,38.3387867480889));
#24215=CARTESIAN_POINT('Ctrl Pts',(-40.6741154471756,36.4255506093119,37.2563306872475));
#24216=CARTESIAN_POINT('Ctrl Pts',(-40.6931272967145,36.4377032948823,37.28084213635));
#24217=CARTESIAN_POINT('Ctrl Pts',(-40.7120508587019,36.4501655961227,37.3052685576269));
#24218=CARTESIAN_POINT('Ctrl Pts',(-40.7308823526258,36.4629350232734,37.3296050712103));
#24219=CARTESIAN_POINT('Ctrl Pts',(-40.7496971250573,36.4756931117658,37.3539199750994));
#24220=CARTESIAN_POINT('Ctrl Pts',(-40.7684199927572,36.488757780916,37.3781451307628));
#24221=CARTESIAN_POINT('Ctrl Pts',(-40.7870472219303,36.5021264253115,37.4022757071157));
#24222=CARTESIAN_POINT('Ctrl Pts',(-40.8056744511035,36.515495069707,37.4264062834685));
#24223=CARTESIAN_POINT('Ctrl Pts',(-40.8242060416511,36.5291676892768,37.4504422803829));
#24224=CARTESIAN_POINT('Ctrl Pts',(-40.8426382979243,36.5431415573687,37.4743789044973));
#24225=CARTESIAN_POINT('Ctrl Pts',(-40.8610705541975,36.5571154254606,37.4983155286117));
#24226=CARTESIAN_POINT('Ctrl Pts',(-40.8794034760984,36.5713905420004,37.5221527797991));
#24227=CARTESIAN_POINT('Ctrl Pts',(-40.8976334075967,36.585964060183,37.5458859043325));
#24228=CARTESIAN_POINT('Ctrl Pts',(-40.9158633390951,36.6005375783655,37.5696190288658));
#24229=CARTESIAN_POINT('Ctrl Pts',(-40.9339902800941,36.6154094981135,37.593248026619));
#24230=CARTESIAN_POINT('Ctrl Pts',(-40.9520106156417,36.6305768536049,37.6167681853963));
#24231=CARTESIAN_POINT('Ctrl Pts',(-40.9700309511894,36.6457442090964,37.6402883441736));
#24232=CARTESIAN_POINT('Ctrl Pts',(-40.98794468119,36.6612070002508,37.66369966385));
#24233=CARTESIAN_POINT('Ctrl Pts',(-41.0057482332104,36.6769621434121,37.6869974756397));
#24234=CARTESIAN_POINT('Ctrl Pts',(-41.0235517852309,36.6927172865733,37.7102952874294));
#24235=CARTESIAN_POINT('Ctrl Pts',(-41.041245159177,36.7087647816577,37.7334795912088));
#24236=CARTESIAN_POINT('Ctrl Pts',(-41.0588248265598,36.7251014284049,37.7565457634644));
#24237=CARTESIAN_POINT('Ctrl Pts',(-41.0764044939427,36.7414380751521,37.77961193572));
#24238=CARTESIAN_POINT('Ctrl Pts',(-41.0938704546694,36.7580638734756,37.8025599763297));
#24239=CARTESIAN_POINT('Ctrl Pts',(-41.1112192256027,36.7749755077871,37.8253853088963));
#24240=CARTESIAN_POINT('Ctrl Pts',(-41.1285679965361,36.7918871420986,37.848210641463));
#24241=CARTESIAN_POINT('Ctrl Pts',(-41.1457995775841,36.8090846123084,37.8709132658657));
#24242=CARTESIAN_POINT('Ctrl Pts',(-41.162910532351,36.8265644888233,37.8934886546498));
#24243=CARTESIAN_POINT('Ctrl Pts',(-41.180021487118,36.8440443653383,37.9160640434337));
#24244=CARTESIAN_POINT('Ctrl Pts',(-41.1970118155131,36.8618066480654,37.9385121964793));
#24245=CARTESIAN_POINT('Ctrl Pts',(-41.2138781292521,36.8798477947743,37.9608286370792));
#24246=CARTESIAN_POINT('Ctrl Pts',(-41.2307444429911,36.8978889414832,37.9831450776791));
#24247=CARTESIAN_POINT('Ctrl Pts',(-41.2474867419845,36.9162089520781,38.0053298057151));
#24248=CARTESIAN_POINT('Ctrl Pts',(-41.2641016874112,36.9348041731036,38.0273783970134));
#24249=CARTESIAN_POINT('Ctrl Pts',(-41.2807166328378,36.9533993941293,38.0494269883118));
#24250=CARTESIAN_POINT('Ctrl Pts',(-41.2972042246096,36.972269825487,38.0713394427555));
#24251=CARTESIAN_POINT('Ctrl Pts',(-41.3135611747002,36.9914117039544,38.0931113904688));
#24252=CARTESIAN_POINT('Ctrl Pts',(-41.3299181247909,37.0105535824219,38.1148833381822));
#24253=CARTESIAN_POINT('Ctrl Pts',(-41.3461444331136,37.0299669078974,38.1365147790498));
#24254=CARTESIAN_POINT('Ctrl Pts',(-41.3622368637482,37.0496478088925,38.1580013992367));
#24255=CARTESIAN_POINT('Ctrl Pts',(-41.3783292943828,37.0693287098876,38.1794880194235));
#24256=CARTESIAN_POINT('Ctrl Pts',(-41.3942878472441,37.0892771862976,38.2008298188158));
#24257=CARTESIAN_POINT('Ctrl Pts',(-41.4101093398088,37.109489259912,38.2220225413402));
#24258=CARTESIAN_POINT('Ctrl Pts',(-41.4259308323735,37.1297013335263,38.2432152638646));
#24259=CARTESIAN_POINT('Ctrl Pts',(-41.4416152645578,37.1501770042377,38.2642589094087));
#24260=CARTESIAN_POINT('Ctrl Pts',(-41.4571595085048,37.1709121886999,38.2851492813583));
#24261=CARTESIAN_POINT('Ctrl Pts',(-41.4727037524518,37.1916473731622,38.306039653308));
#24262=CARTESIAN_POINT('Ctrl Pts',(-41.4881078080792,37.2126420712653,38.3267767515524));
#24263=CARTESIAN_POINT('Ctrl Pts',(-41.5033686034439,37.2338920961565,38.3473564406104));
#24264=CARTESIAN_POINT('Ctrl Pts',(-40.6383034478792,36.4097377289922,37.2359354169989));
#24265=CARTESIAN_POINT('Ctrl Pts',(-40.6579122186806,36.4219506815113,37.2611218870834));
#24266=CARTESIAN_POINT('Ctrl Pts',(-40.6774298256422,36.4344902290624,37.2862208723249));
#24267=CARTESIAN_POINT('Ctrl Pts',(-40.69685217458,36.4473537380318,37.3112271067932));
#24268=CARTESIAN_POINT('Ctrl Pts',(-40.7162572773736,36.4602058248024,37.3362111368863));
#24269=CARTESIAN_POINT('Ctrl Pts',(-40.7355672911245,36.4733812978462,37.361102580704));
#24270=CARTESIAN_POINT('Ctrl Pts',(-40.7547781723612,36.4868773952691,37.3858962251053));
#24271=CARTESIAN_POINT('Ctrl Pts',(-40.7739890535979,36.500373492692,37.4106898695066));
#24272=CARTESIAN_POINT('Ctrl Pts',(-40.7931008022082,36.514190214415,37.4353857143468));
#24273=CARTESIAN_POINT('Ctrl Pts',(-40.812109416228,36.5283246644106,37.4599785874381));
#24274=CARTESIAN_POINT('Ctrl Pts',(-40.8311180302477,36.5424591144063,37.4845714605293));
#24275=CARTESIAN_POINT('Ctrl Pts',(-40.8500235095659,36.5569112925918,37.509061361728));
#24276=CARTESIAN_POINT('Ctrl Pts',(-40.8688218953962,36.5716781700165,37.5334431619606));
#24277=CARTESIAN_POINT('Ctrl Pts',(-40.8876202812265,36.5864450474411,37.5578249621932));
#24278=CARTESIAN_POINT('Ctrl Pts',(-40.9063115734591,36.6015266240186,37.5820986613173));
#24279=CARTESIAN_POINT('Ctrl Pts',(-40.9248918581412,36.6169197391423,37.6062591755176));
#24280=CARTESIAN_POINT('Ctrl Pts',(-40.9434721428234,36.6323128542659,37.630419689718));
#24281=CARTESIAN_POINT('Ctrl Pts',(-40.9619414198465,36.6480175078458,37.6544670188535));
#24282=CARTESIAN_POINT('Ctrl Pts',(-40.9802958217256,36.6640304089406,37.6783961264914));
#24283=CARTESIAN_POINT('Ctrl Pts',(-40.9986502236047,36.6800433100354,37.7023252341293));
#24284=CARTESIAN_POINT('Ctrl Pts',(-41.0168897502328,36.6963644585517,37.72613612013));
#24285=CARTESIAN_POINT('Ctrl Pts',(-41.0350105822093,36.7129904345898,37.7498237975483));
#24286=CARTESIAN_POINT('Ctrl Pts',(-41.0531314141859,36.7296164106278,37.7735114749666));
#24287=CARTESIAN_POINT('Ctrl Pts',(-41.0711335514053,36.7465472140907,37.7970759436644));
#24288=CARTESIAN_POINT('Ctrl Pts',(-41.0890132241472,36.7637792975502,37.8205122682682));
#24289=CARTESIAN_POINT('Ctrl Pts',(-41.1068928968892,36.7810113810095,37.843948592872));
#24290=CARTESIAN_POINT('Ctrl Pts',(-41.1246501050495,36.7985447443649,37.8672567732451));
#24291=CARTESIAN_POINT('Ctrl Pts',(-41.1422811301639,36.8163757141427,37.8904319276488));
#24292=CARTESIAN_POINT('Ctrl Pts',(-41.1599121552782,36.8342066839207,37.9136070820524));
#24293=CARTESIAN_POINT('Ctrl Pts',(-41.1774169972437,36.8523352600169,37.9366492103513));
#24294=CARTESIAN_POINT('Ctrl Pts',(-41.1947919904053,36.8707576444486,37.9595534864814));
#24295=CARTESIAN_POINT('Ctrl Pts',(-41.2121669835669,36.8891800288803,37.9824577626115));
#24296=CARTESIAN_POINT('Ctrl Pts',(-41.2294121278233,36.9078962215397,38.0052241864391));
#24297=CARTESIAN_POINT('Ctrl Pts',(-41.246523811861,36.926902301522,38.0278479895921));
#24298=CARTESIAN_POINT('Ctrl Pts',(-41.2636354958986,36.9459083815043,38.050471792745));
#24299=CARTESIAN_POINT('Ctrl Pts',(-41.2806137196176,36.9652043486984,38.0729529750912));
#24300=CARTESIAN_POINT('Ctrl Pts',(-41.2974549275547,36.9847861609168,38.095286827943));
#24301=CARTESIAN_POINT('Ctrl Pts',(-41.3142961354918,37.0043679731352,38.1176206807948));
#24302=CARTESIAN_POINT('Ctrl Pts',(-41.3310003275487,37.0242356302634,38.139807204022));
#24303=CARTESIAN_POINT('Ctrl Pts',(-41.3475640055984,37.0443849705206,38.1618417505897));
#24304=CARTESIAN_POINT('Ctrl Pts',(-41.3641276836481,37.0645343107778,38.1838762971574));
#24305=CARTESIAN_POINT('Ctrl Pts',(-41.380550847594,37.0849653340465,38.2057588669369));
#24306=CARTESIAN_POINT('Ctrl Pts',(-41.3968300581068,37.1056737606922,38.2274848764885));
#24307=CARTESIAN_POINT('Ctrl Pts',(-41.4131092686196,37.1263821873379,38.2492108860401));
#24308=CARTESIAN_POINT('Ctrl Pts',(-41.4292445256044,37.1473680172397,38.2707803352369));
#24309=CARTESIAN_POINT('Ctrl Pts',(-41.4452324499675,37.1686268546986,38.2921887061499));
#24310=CARTESIAN_POINT('Ctrl Pts',(-41.4612203743306,37.1898856921576,38.3135970770628));
#24311=CARTESIAN_POINT('Ctrl Pts',(-41.4770609659786,37.2114175370495,38.3348443695669));
#24312=CARTESIAN_POINT('Ctrl Pts',(-41.492750907465,37.2332178794481,38.3559261331319));
#24313=CARTESIAN_POINT('Ctrl Pts',(-40.6031670153025,36.3949061682344,37.2163852571093));
#24314=CARTESIAN_POINT('Ctrl Pts',(-40.623357249323,36.407156485292,37.2422275464382));
#24315=CARTESIAN_POINT('Ctrl Pts',(-40.643453630599,36.4197505664764,37.2679801100193));
#24316=CARTESIAN_POINT('Ctrl Pts',(-40.6634517347483,36.4326856357027,37.2936372773184));
#24317=CARTESIAN_POINT('Ctrl Pts',(-40.6834320815095,36.445609219188,37.319271662244));
#24318=CARTESIAN_POINT('Ctrl Pts',(-40.7033143254858,36.458873185345,37.3448108200719));
#24319=CARTESIAN_POINT('Ctrl Pts',(-40.7230940972037,36.4724746160314,37.3702491372292));
#24320=CARTESIAN_POINT('Ctrl Pts',(-40.7428738689217,36.4860760467178,37.3956874543864));
#24321=CARTESIAN_POINT('Ctrl Pts',(-40.7625511682547,36.5000149418463,37.4210249307097));
#24322=CARTESIAN_POINT('Ctrl Pts',(-40.78212167078,36.5142882351113,37.4462559969579));
#24323=CARTESIAN_POINT('Ctrl Pts',(-40.8016921733053,36.5285615283763,37.4714870632061));
#24324=CARTESIAN_POINT('Ctrl Pts',(-40.8211558789267,36.5431692197013,37.4966117192332));
#24325=CARTESIAN_POINT('Ctrl Pts',(-40.8405085100752,36.5581080959174,37.5216244425211));
#24326=CARTESIAN_POINT('Ctrl Pts',(-40.8598611412237,36.5730469721334,37.546637165809));
#24327=CARTESIAN_POINT('Ctrl Pts',(-40.8791026977786,36.5883170331452,37.571537956199));
#24328=CARTESIAN_POINT('Ctrl Pts',(-40.8982289511076,36.603914920437,37.5963213404317));
#24329=CARTESIAN_POINT('Ctrl Pts',(-40.9173552044367,36.6195128077287,37.6211047246645));
#24330=CARTESIAN_POINT('Ctrl Pts',(-40.9363661543852,36.6354385211834,37.6457707025633));
#24331=CARTESIAN_POINT('Ctrl Pts',(-40.9552576229183,36.6516885583113,37.6703138524221));
#24332=CARTESIAN_POINT('Ctrl Pts',(-40.9741490914513,36.6679385954392,37.6948570022809));
#24333=CARTESIAN_POINT('Ctrl Pts',(-40.9929210784476,36.6845129561356,37.719277323942));
#24334=CARTESIAN_POINT('Ctrl Pts',(-41.0115694583644,36.7014079955075,37.7435694496648));
#24335=CARTESIAN_POINT('Ctrl Pts',(-41.0302178382813,36.7183030348793,37.7678615753875));
#24336=CARTESIAN_POINT('Ctrl Pts',(-41.0487426109916,36.7355187528129,37.7920255050113));
#24337=CARTESIAN_POINT('Ctrl Pts',(-41.0671397052689,36.7530513636207,37.8160559271245));
#24338=CARTESIAN_POINT('Ctrl Pts',(-41.0855367995463,36.7705839744285,37.8400863492377));
#24339=CARTESIAN_POINT('Ctrl Pts',(-41.1038062152716,36.7884334779974,37.8639832636854));
#24340=CARTESIAN_POINT('Ctrl Pts',(-41.1219439372768,36.8065959494778,37.8877414176876));
#24341=CARTESIAN_POINT('Ctrl Pts',(-41.1400816592819,36.8247584209582,37.9114995716897));
#24342=CARTESIAN_POINT('Ctrl Pts',(-41.1580876874573,36.8432338602379,37.9351189650979));
#24343=CARTESIAN_POINT('Ctrl Pts',(-41.1759580644957,36.8620182050557,37.9585944060939));
#24344=CARTESIAN_POINT('Ctrl Pts',(-41.1938284415342,36.8808025498736,37.9820698470898));
#24345=CARTESIAN_POINT('Ctrl Pts',(-41.2115631673208,36.8998958001088,38.0054013355226));
#24346=CARTESIAN_POINT('Ctrl Pts',(-41.2291583441313,36.9192937578614,38.0285837428043));
#24347=CARTESIAN_POINT('Ctrl Pts',(-41.2467535209419,36.938691715614,38.051766150086));
#24348=CARTESIAN_POINT('Ctrl Pts',(-41.2642091486756,36.9583943807689,38.0747994760747));
#24349=CARTESIAN_POINT('Ctrl Pts',(-41.2815213908748,36.9783974216099,38.0976786576474));
#24350=CARTESIAN_POINT('Ctrl Pts',(-41.2988336330739,36.9984004624509,38.1205578392202));
#24351=CARTESIAN_POINT('Ctrl Pts',(-41.3160024896306,37.0187038788512,38.1432828762316));
#24352=CARTESIAN_POINT('Ctrl Pts',(-41.3330241871075,37.0393032072343,38.1658487732862));
#24353=CARTESIAN_POINT('Ctrl Pts',(-41.3500458845845,37.0599025356174,38.1884146703408));
#24354=CARTESIAN_POINT('Ctrl Pts',(-41.3669204228617,37.080797775842,38.2108214272873));
#24355=CARTESIAN_POINT('Ctrl Pts',(-41.3836440931108,37.1019843343765,38.2330641186097));
#24356=CARTESIAN_POINT('Ctrl Pts',(-41.4003677633599,37.1231708929111,38.2553068099321));
#24357=CARTESIAN_POINT('Ctrl Pts',(-41.4169405654734,37.1446487696193,38.2773854354873));
#24358=CARTESIAN_POINT('Ctrl Pts',(-41.4333588568789,37.1664132430457,38.2992951418114));
#24359=CARTESIAN_POINT('Ctrl Pts',(-41.4497771482844,37.1881777164722,38.3212048481356));
#24360=CARTESIAN_POINT('Ctrl Pts',(-41.4660409288741,37.2102287864741,38.3429456350853));
#24361=CARTESIAN_POINT('Ctrl Pts',(-41.4821466239335,37.2325616057495,38.3645127233828));
#24362=CARTESIAN_POINT('Ctrl Pts',(-40.5686122648838,36.3808986978976,37.1975487055119));
#24363=CARTESIAN_POINT('Ctrl Pts',(-40.5893703835316,36.3931671620808,37.2240302748371));
#24364=CARTESIAN_POINT('Ctrl Pts',(-40.6100321454547,36.4057967134211,37.2504200896056));
#24365=CARTESIAN_POINT('Ctrl Pts',(-40.630592780513,36.4187844360772,37.2767120572633));
#24366=CARTESIAN_POINT('Ctrl Pts',(-40.6511351586819,36.4317606262385,37.3029806788743));
#24367=CARTESIAN_POINT('Ctrl Pts',(-40.6715765893685,36.4450943518338,37.3291516268873));
#24368=CARTESIAN_POINT('Ctrl Pts',(-40.6919123616709,36.4587825399943,37.3552188699908));
#24369=CARTESIAN_POINT('Ctrl Pts',(-40.7122481339734,36.4724707281547,37.3812861130943));
#24370=CARTESIAN_POINT('Ctrl Pts',(-40.7324782477483,36.4865133787835,37.4072496511039));
#24371=CARTESIAN_POINT('Ctrl Pts',(-40.7525980408097,36.5009072556416,37.4331035005162));
#24372=CARTESIAN_POINT('Ctrl Pts',(-40.7727178338711,36.5153011324998,37.4589573499286));
#24373=CARTESIAN_POINT('Ctrl Pts',(-40.7927273061048,36.5300462354996,37.4847015105758));
#24374=CARTESIAN_POINT('Ctrl Pts',(-40.8126218461008,36.5451391664803,37.5103300494723));
#24375=CARTESIAN_POINT('Ctrl Pts',(-40.8325163860967,36.5602320974612,37.5359585883689));
#24376=CARTESIAN_POINT('Ctrl Pts',(-40.8522959937176,36.5756728563167,37.5614715053352));
#24377=CARTESIAN_POINT('Ctrl Pts',(-40.8719561106524,36.5914578846304,37.5868629207453));
#24378=CARTESIAN_POINT('Ctrl Pts',(-40.8916162275871,36.607242912944,37.6122543361554));
#24379=CARTESIAN_POINT('Ctrl Pts',(-40.9111568536662,36.6233722105883,37.6375242498129));
#24380=CARTESIAN_POINT('Ctrl Pts',(-40.9305734855941,36.6398420604359,37.6626668380618));
#24381=CARTESIAN_POINT('Ctrl Pts',(-40.949990117522,36.6563119102835,37.6878094263107));
#24382=CARTESIAN_POINT('Ctrl Pts',(-40.9692827551612,36.6731223122178,37.7128246889728));
#24383=CARTESIAN_POINT('Ctrl Pts',(-40.9884469523672,36.6902693921455,37.7377068610782));
#24384=CARTESIAN_POINT('Ctrl Pts',(-41.0076111495731,36.7074164720732,37.7625890331836));
#24385=CARTESIAN_POINT('Ctrl Pts',(-41.026646906203,36.7249002298684,37.7873381145518));
#24386=CARTESIAN_POINT('Ctrl Pts',(-41.0455498353268,36.7427166362666,37.8119484015653));
#24387=CARTESIAN_POINT('Ctrl Pts',(-41.0644527644507,36.7605330426647,37.8365586885788));
#24388=CARTESIAN_POINT('Ctrl Pts',(-41.0832228659336,36.7786820975395,37.861030181063));
#24389=CARTESIAN_POINT('Ctrl Pts',(-41.1018558140411,36.7971596182853,37.885357239356));
#24390=CARTESIAN_POINT('Ctrl Pts',(-41.1204887621484,36.8156371390313,37.909684297649));
#24391=CARTESIAN_POINT('Ctrl Pts',(-41.1389845567548,36.8344431255219,37.9338669215827));
#24392=CARTESIAN_POINT('Ctrl Pts',(-41.1573389353545,36.8535732437653,37.9578995380755));
#24393=CARTESIAN_POINT('Ctrl Pts',(-41.1756933139542,36.8727033620086,37.9819321545683));
#24394=CARTESIAN_POINT('Ctrl Pts',(-41.1939062764172,36.8921576118694,38.0058147634501));
#24395=CARTESIAN_POINT('Ctrl Pts',(-41.2119736254189,36.911931509958,38.0295418607802));
#24396=CARTESIAN_POINT('Ctrl Pts',(-41.2300409744206,36.9317054080466,38.0532689581103));
#24397=CARTESIAN_POINT('Ctrl Pts',(-41.2479627098447,36.951798954232,38.0768405437274));
#24398=CARTESIAN_POINT('Ctrl Pts',(-41.2657347014578,36.9722075177754,38.1002511853549));
#24399=CARTESIAN_POINT('Ctrl Pts',(-41.283506693071,36.9926160813189,38.1236618269823));
#24400=CARTESIAN_POINT('Ctrl Pts',(-41.3011289407505,37.0133396620775,38.1469115244559));
#24401=CARTESIAN_POINT('Ctrl Pts',(-41.3185973833262,37.0343734841502,38.169994919706));
#24402=CARTESIAN_POINT('Ctrl Pts',(-41.336065825902,37.0554073062227,38.1930783149561));
#24403=CARTESIAN_POINT('Ctrl Pts',(-41.3533804632401,37.0767513694522,38.2159954078134));
#24404=CARTESIAN_POINT('Ctrl Pts',(-41.3705373050422,37.0984007549263,38.2387409168482));
#24405=CARTESIAN_POINT('Ctrl Pts',(-41.3876941468442,37.1200501404005,38.2614864258829));
#24406=CARTESIAN_POINT('Ctrl Pts',(-41.4046931929887,37.142004847966,38.284060350934));
#24407=CARTESIAN_POINT('Ctrl Pts',(-41.4215305259077,37.1642598179827,38.3064574896577));
#24408=CARTESIAN_POINT('Ctrl Pts',(-41.4383678588268,37.1865147879992,38.3288546283815));
#24409=CARTESIAN_POINT('Ctrl Pts',(-41.455043478399,37.2090700203066,38.3510749806165));
#24410=CARTESIAN_POINT('Ctrl Pts',(-41.4715535415974,37.2319203168746,38.3731134255079));
#24411=CARTESIAN_POINT('Ctrl Pts',(-40.4995027640465,36.3528837572238,37.1598756023172));
#24412=CARTESIAN_POINT('Ctrl Pts',(-40.5213966519487,36.3651885156582,37.187635731635));
#24413=CARTESIAN_POINT('Ctrl Pts',(-40.5431891751662,36.3778890073104,37.2153000487784));
#24414=CARTESIAN_POINT('Ctrl Pts',(-40.5648748720426,36.3909820368262,37.2428616171533));
#24415=CARTESIAN_POINT('Ctrl Pts',(-40.5865413130269,36.4040634403395,37.2703987121349));
#24416=CARTESIAN_POINT('Ctrl Pts',(-40.6081011171338,36.4175366848114,37.297833240518));
#24417=CARTESIAN_POINT('Ctrl Pts',(-40.6295488906053,36.43139838792,37.325158335514));
#24418=CARTESIAN_POINT('Ctrl Pts',(-40.6509966640768,36.4452600910285,37.35248343051));
#24419=CARTESIAN_POINT('Ctrl Pts',(-40.6723324067354,36.459510252658,37.3796990918922));
#24420=CARTESIAN_POINT('Ctrl Pts',(-40.6935507808691,36.4741452967023,37.4067985076328));
#24421=CARTESIAN_POINT('Ctrl Pts',(-40.7147691550028,36.4887803407466,37.4338979233734));
#24422=CARTESIAN_POINT('Ctrl Pts',(-40.7358701604611,36.5038002670961,37.4608810932608));
#24423=CARTESIAN_POINT('Ctrl Pts',(-40.756848518152,36.5192013076064,37.4877412633747));
#24424=CARTESIAN_POINT('Ctrl Pts',(-40.7778268758429,36.5346023481166,37.5146014334885));
#24425=CARTESIAN_POINT('Ctrl Pts',(-40.7986825855956,36.5503845026598,37.5413386036076));
#24426=CARTESIAN_POINT('Ctrl Pts',(-40.8194104297418,36.5665438130171,37.5679460813723));
#24427=CARTESIAN_POINT('Ctrl Pts',(-40.840138273888,36.5827031233745,37.5945535591371));
#24428=CARTESIAN_POINT('Ctrl Pts',(-40.8607382522283,36.5992395893979,37.6210313443123));
#24429=CARTESIAN_POINT('Ctrl Pts',(-40.8812052109459,36.6161490646851,37.6473728093412));
#24430=CARTESIAN_POINT('Ctrl Pts',(-40.9016721696634,36.6330585399722,37.6737142743702));
#24431=CARTESIAN_POINT('Ctrl Pts',(-40.9220061085886,36.6503410243821,37.6999194190343));
#24432=CARTESIAN_POINT('Ctrl Pts',(-40.9422019403726,36.6679921854215,37.725981683905));
#24433=CARTESIAN_POINT('Ctrl Pts',(-40.9623977721567,36.6856433464611,37.7520439487757));
#24434=CARTESIAN_POINT('Ctrl Pts',(-40.9824554966259,36.7036631839793,37.7779633336328));
#24435=CARTESIAN_POINT('Ctrl Pts',(-41.0023700954427,36.7220471815582,37.8037333504469));
#24436=CARTESIAN_POINT('Ctrl Pts',(-41.0222846942595,36.740431179137,37.8295033672612));
#24437=CARTESIAN_POINT('Ctrl Pts',(-41.0420561672579,36.7591793366235,37.8551240158183));
#24438=CARTESIAN_POINT('Ctrl Pts',(-41.0616795675697,36.7782869559004,37.8805888826929));
#24439=CARTESIAN_POINT('Ctrl Pts',(-41.0813029678815,36.7973945751773,37.9060537495676));
#24440=CARTESIAN_POINT('Ctrl Pts',(-41.1007782953498,36.8168616560897,37.9313628345522));
#24441=CARTESIAN_POINT('Ctrl Pts',(-41.1201006770721,36.8366833211842,37.9565098020388));
#24442=CARTESIAN_POINT('Ctrl Pts',(-41.1394230587942,36.8565049862788,37.9816567695253));
#24443=CARTESIAN_POINT('Ctrl Pts',(-41.15859249461,36.8766812353907,38.006641619305));
#24444=CARTESIAN_POINT('Ctrl Pts',(-41.1776041879939,36.8972070141512,38.0314580967319));
#24445=CARTESIAN_POINT('Ctrl Pts',(-41.1966158813778,36.9177327929118,38.0562745741588));
#24446=CARTESIAN_POINT('Ctrl Pts',(-41.2154698321827,36.9386081011583,38.0809226790329));
#24447=CARTESIAN_POINT('Ctrl Pts',(-41.2341613226239,36.9598277101066,38.1053962407698));
#24448=CARTESIAN_POINT('Ctrl Pts',(-41.2528528130651,36.9810473190549,38.1298698025067));
#24449=CARTESIAN_POINT('Ctrl Pts',(-41.2713818429903,37.0026112285302,38.1541688209045));
#24450=CARTESIAN_POINT('Ctrl Pts',(-41.2897437757637,37.0245140379819,38.1782872125456));
#24451=CARTESIAN_POINT('Ctrl Pts',(-41.308105708537,37.0464168474336,38.2024056041867));
#24452=CARTESIAN_POINT('Ctrl Pts',(-41.3263005439969,37.0686585566726,38.2263433688655));
#24453=CARTESIAN_POINT('Ctrl Pts',(-41.3443237289049,37.0912335960259,38.250094513325));
#24454=CARTESIAN_POINT('Ctrl Pts',(-41.3623469138128,37.1138086353793,38.2738456577845));
#24455=CARTESIAN_POINT('Ctrl Pts',(-41.3801984480191,37.1367170046594,38.2974101818276));
#24456=CARTESIAN_POINT('Ctrl Pts',(-41.3978738639654,37.1599529678564,38.3207821853503));
#24457=CARTESIAN_POINT('Ctrl Pts',(-41.4155492799117,37.1831889310534,38.3441541888731));
#24458=CARTESIAN_POINT('Ctrl Pts',(-41.433048577449,37.2067524879717,38.3673336716789));
#24459=CARTESIAN_POINT('Ctrl Pts',(-41.4503673769252,37.2306377391247,38.3903148297581));
#24460=CARTESIAN_POINT('Ctrl Pts',(-40.4327066305705,36.3281417176076,37.1250374865186));
#24461=CARTESIAN_POINT('Ctrl Pts',(-40.4556822337068,36.3404064517208,37.1540104055611));
#24462=CARTESIAN_POINT('Ctrl Pts',(-40.4785522041448,36.3531021756841,37.1828843032254));
#24463=CARTESIAN_POINT('Ctrl Pts',(-40.5013103265027,36.3662254256052,37.2116513292939));
#24464=CARTESIAN_POINT('Ctrl Pts',(-40.5240482407043,36.3793370226897,37.2403928115787));
#24465=CARTESIAN_POINT('Ctrl Pts',(-40.5466745051614,36.3928753866999,37.2690276117041));
#24466=CARTESIAN_POINT('Ctrl Pts',(-40.5691829815726,36.4068368320582,37.2975479582549));
#24467=CARTESIAN_POINT('Ctrl Pts',(-40.591691457984,36.4207982774164,37.3260683048058));
#24468=CARTESIAN_POINT('Ctrl Pts',(-40.6140821461322,36.4351828039857,37.3544741975048));
#24469=CARTESIAN_POINT('Ctrl Pts',(-40.6363489717272,36.449986497345,37.3827579271217));
#24470=CARTESIAN_POINT('Ctrl Pts',(-40.6586157973222,36.4647901907043,37.4110416567386));
#24471=CARTESIAN_POINT('Ctrl Pts',(-40.680758760124,36.4800130506985,37.4392032229855));
#24472=CARTESIAN_POINT('Ctrl Pts',(-40.7027718529873,36.4956509361219,37.4672349829013));
#24473=CARTESIAN_POINT('Ctrl Pts',(-40.7247849458505,36.5112888215454,37.495266742817));
#24474=CARTESIAN_POINT('Ctrl Pts',(-40.7466681685606,36.5273417322445,37.5231686961282));
#24475=CARTESIAN_POINT('Ctrl Pts',(-40.7684155844015,36.543805302488,37.5509332702886));
#24476=CARTESIAN_POINT('Ctrl Pts',(-40.7901630002423,36.5602688727316,37.5786978444489));
#24477=CARTESIAN_POINT('Ctrl Pts',(-40.8117746090018,36.577143102358,37.6063250391875));
#24478=CARTESIAN_POINT('Ctrl Pts',(-40.8332445475919,36.5944234034702,37.6338073564561));
#24479=CARTESIAN_POINT('Ctrl Pts',(-40.8547144861819,36.6117037045823,37.6612896737247));
#24480=CARTESIAN_POINT('Ctrl Pts',(-40.8760427543934,36.6293900770107,37.6886271132553));
#24481=CARTESIAN_POINT('Ctrl Pts',(-40.897223565927,36.6474777131718,37.7158122555411));
#24482=CARTESIAN_POINT('Ctrl Pts',(-40.9184043774606,36.6655653493329,37.7429973978269));
#24483=CARTESIAN_POINT('Ctrl Pts',(-40.9394377321161,36.684054249053,37.7700302426063));
#24484=CARTESIAN_POINT('Ctrl Pts',(-40.9603179234896,36.7029393876519,37.7969034529082));
#24485=CARTESIAN_POINT('Ctrl Pts',(-40.9811981148631,36.7218245262507,37.8237766632102));
#24486=CARTESIAN_POINT('Ctrl Pts',(-41.0019251427519,36.7411059035437,37.8504902387728));
#24487=CARTESIAN_POINT('Ctrl Pts',(-41.0224933837594,36.7607782804895,37.8770369291384));
#24488=CARTESIAN_POINT('Ctrl Pts',(-41.0430616247668,36.7804506574353,37.9035836195039));
#24489=CARTESIAN_POINT('Ctrl Pts',(-41.0634710786868,36.800514033838,37.9299634244099));
#24490=CARTESIAN_POINT('Ctrl Pts',(-41.0837162081265,36.820962959103,37.9561691838015));
#24491=CARTESIAN_POINT('Ctrl Pts',(-41.1039613375662,36.841411884368,37.9823749431932));
#24492=CARTESIAN_POINT('Ctrl Pts',(-41.1240421423282,36.8622463582954,38.0084066568147));
#24493=CARTESIAN_POINT('Ctrl Pts',(-41.1439531740197,36.8834607216871,38.0342572588823));
#24494=CARTESIAN_POINT('Ctrl Pts',(-41.1638642057111,36.9046750850788,38.0601078609499));
#24495=CARTESIAN_POINT('Ctrl Pts',(-41.1836054641379,36.9262693377276,38.0857773512114));
#24496=CARTESIAN_POINT('Ctrl Pts',(-41.2031715928443,36.9482376148864,38.1112587619649));
#24497=CARTESIAN_POINT('Ctrl Pts',(-41.2227377215506,36.9702058920454,38.1367401727183));
#24498=CARTESIAN_POINT('Ctrl Pts',(-41.2421287203456,36.9925481934999,38.1620335037149));
#24499=CARTESIAN_POINT('Ctrl Pts',(-41.2613393275985,37.0152584521198,38.1871318890929));
#24500=CARTESIAN_POINT('Ctrl Pts',(-41.2805499348514,37.0379687107396,38.2122302744709));
#24501=CARTESIAN_POINT('Ctrl Pts',(-41.2995801503747,37.061046926303,38.2371337139852));
#24502=CARTESIAN_POINT('Ctrl Pts',(-41.3184248101988,37.0844868325701,38.2618354473172));
#24503=CARTESIAN_POINT('Ctrl Pts',(-41.3372694700231,37.1079267388372,38.2865371806492));
#24504=CARTESIAN_POINT('Ctrl Pts',(-41.3559285739644,37.131728335579,38.3110372075577));
#24505=CARTESIAN_POINT('Ctrl Pts',(-41.3743970584991,37.1558851608273,38.3353288769137));
#24506=CARTESIAN_POINT('Ctrl Pts',(-41.3928655430338,37.1800419860756,38.3596205462697));
#24507=CARTESIAN_POINT('Ctrl Pts',(-41.4111434079833,37.2045540395965,38.3837038578382));
#24508=CARTESIAN_POINT('Ctrl Pts',(-41.4292256929962,37.2294146671748,38.4075722732637));
#24509=CARTESIAN_POINT('Ctrl Pts',(-40.3676750517867,36.3058114897981,37.0923047496203));
#24510=CARTESIAN_POINT('Ctrl Pts',(-40.3916895837106,36.3179798469043,37.1224397291744));
#24511=CARTESIAN_POINT('Ctrl Pts',(-40.4155949225065,36.3306148746499,37.1524732849664));
#24512=CARTESIAN_POINT('Ctrl Pts',(-40.4393840426075,36.3437128595723,37.1823965903769));
#24513=CARTESIAN_POINT('Ctrl Pts',(-40.4631520390742,36.3567992140922,37.2122933252813));
#24514=CARTESIAN_POINT('Ctrl Pts',(-40.4868040228878,36.3703477038401,37.2420800051752));
#24515=CARTESIAN_POINT('Ctrl Pts',(-40.5103330551856,36.384354354058,37.271747891473));
#24516=CARTESIAN_POINT('Ctrl Pts',(-40.5338620874834,36.3983610042759,37.3014157777707));
#24517=CARTESIAN_POINT('Ctrl Pts',(-40.5572681679973,36.4128258148029,37.3309648701328));
#24518=CARTESIAN_POINT('Ctrl Pts',(-40.5805444300924,36.4277445420935,37.3603864997192));
#24519=CARTESIAN_POINT('Ctrl Pts',(-40.6038206921875,36.4426632693841,37.3898081293055));
#24520=CARTESIAN_POINT('Ctrl Pts',(-40.6269671355757,36.4580359132583,37.4191022957678));
#24521=CARTESIAN_POINT('Ctrl Pts',(-40.6499769697499,36.4738579638206,37.4482604050325));
#24522=CARTESIAN_POINT('Ctrl Pts',(-40.6729868039241,36.4896800143829,37.4774185142971));
#24523=CARTESIAN_POINT('Ctrl Pts',(-40.6958600286203,36.5059514714516,37.5064405660295));
#24524=CARTESIAN_POINT('Ctrl Pts',(-40.7185899334867,36.5226675614453,37.5353180459871));
#24525=CARTESIAN_POINT('Ctrl Pts',(-40.741319838353,36.5393836514389,37.5641955259447));
#24526=CARTESIAN_POINT('Ctrl Pts',(-40.7639064231285,36.5565443741655,37.592928433796));
#24527=CARTESIAN_POINT('Ctrl Pts',(-40.786343061553,36.5741446951584,37.6215083401248));
#24528=CARTESIAN_POINT('Ctrl Pts',(-40.8087796999776,36.5917450161511,37.6500882464537));
#24529=CARTESIAN_POINT('Ctrl Pts',(-40.8310663917936,36.6097849352079,37.6785151509322));
#24530=CARTESIAN_POINT('Ctrl Pts',(-40.8531965987211,36.628259159931,37.7067807139168));
#24531=CARTESIAN_POINT('Ctrl Pts',(-40.8753268056486,36.646733384654,37.7350462769015));
#24532=CARTESIAN_POINT('Ctrl Pts',(-40.8973005274392,36.6656419148345,37.7631504980711));
#24533=CARTESIAN_POINT('Ctrl Pts',(-40.9191113176179,36.6849792032419,37.7910851324419));
#24534=CARTESIAN_POINT('Ctrl Pts',(-40.9409221077965,36.7043164916494,37.8190197668126));
#24535=CARTESIAN_POINT('Ctrl Pts',(-40.9625699661137,36.724082538062,37.8467848140641));
#24536=CARTESIAN_POINT('Ctrl Pts',(-40.9840485417151,36.7442715436917,37.8743721287291));
#24537=CARTESIAN_POINT('Ctrl Pts',(-41.0055271173165,36.7644605493214,37.9019594433941));
#24538=CARTESIAN_POINT('Ctrl Pts',(-41.0268364099504,36.7850725139334,37.9293690251529));
#24539=CARTESIAN_POINT('Ctrl Pts',(-41.0479701680778,36.8061013905645,37.9565928328155));
#24540=CARTESIAN_POINT('Ctrl Pts',(-41.0691039262052,36.8271302671957,37.9838166404781));
#24541=CARTESIAN_POINT('Ctrl Pts',(-41.0900621495836,36.8485760556048,38.0108546737322));
#24542=CARTESIAN_POINT('Ctrl Pts',(-41.1108386896676,36.8704324642089,38.0376990003894));
#24543=CARTESIAN_POINT('Ctrl Pts',(-41.1316152297516,36.892288872813,38.0645433270466));
#24544=CARTESIAN_POINT('Ctrl Pts',(-41.1522100863028,36.9145559013613,38.0911939467988));
#24545=CARTESIAN_POINT('Ctrl Pts',(-41.1726172173773,36.9372270173422,38.1176430411141));
#24546=CARTESIAN_POINT('Ctrl Pts',(-41.1930243484518,36.959898133323,38.1440921354294));
#24547=CARTESIAN_POINT('Ctrl Pts',(-41.2132437538154,36.9829733364764,38.170339704004));
#24548=CARTESIAN_POINT('Ctrl Pts',(-41.2332695016711,37.0064458571953,38.1963780465497));
#24549=CARTESIAN_POINT('Ctrl Pts',(-41.2532952495268,37.0299183779144,38.2224163890953));
#24550=CARTESIAN_POINT('Ctrl Pts',(-41.2731273396446,37.0537882159297,38.2482455053131));
#24551=CARTESIAN_POINT('Ctrl Pts',(-41.2927599538546,37.0780483685113,38.2738578176767));
#24552=CARTESIAN_POINT('Ctrl Pts',(-41.3123925680647,37.1023085210928,38.2994701300402));
#24553=CARTESIAN_POINT('Ctrl Pts',(-41.3318257061416,37.1269589879621,38.3248656382556));
#24554=CARTESIAN_POINT('Ctrl Pts',(-41.3510536669568,37.151992537375,38.3500368920045));
#24555=CARTESIAN_POINT('Ctrl Pts',(-41.3702816277719,37.1770260867878,38.3752081457535));
#24556=CARTESIAN_POINT('Ctrl Pts',(-41.3893044111062,37.202442718459,38.4001551447491));
#24557=CARTESIAN_POINT('Ctrl Pts',(-41.4081164362138,37.228234975869,38.4248705702491));
#24558=CARTESIAN_POINT('Ctrl Pts',(-40.3026434730029,36.2834812619887,37.0595720127219));
#24559=CARTESIAN_POINT('Ctrl Pts',(-40.3276969337144,36.2955532420878,37.0908690527878));
#24560=CARTESIAN_POINT('Ctrl Pts',(-40.3526376408682,36.3081275736156,37.1220622667074));
#24561=CARTESIAN_POINT('Ctrl Pts',(-40.3774577587123,36.3212002935394,37.1531418514599));
#24562=CARTESIAN_POINT('Ctrl Pts',(-40.402255837444,36.3342614054947,37.184193838984));
#24563=CARTESIAN_POINT('Ctrl Pts',(-40.4269335406142,36.3478200209803,37.2151323986463));
#24564=CARTESIAN_POINT('Ctrl Pts',(-40.4514831287985,36.3618718760578,37.245947824691));
#24565=CARTESIAN_POINT('Ctrl Pts',(-40.4760327169828,36.3759237311353,37.2767632507357));
#24566=CARTESIAN_POINT('Ctrl Pts',(-40.5004541898623,36.3904688256201,37.3074555427608));
#24567=CARTESIAN_POINT('Ctrl Pts',(-40.5247398884576,36.405502586842,37.3380150723166));
#24568=CARTESIAN_POINT('Ctrl Pts',(-40.5490255870529,36.4205363480638,37.3685746018725));
#24569=CARTESIAN_POINT('Ctrl Pts',(-40.5731755110274,36.436058775818,37.3990013685501));
#24570=CARTESIAN_POINT('Ctrl Pts',(-40.5971820865126,36.4520649915192,37.4292858271637));
#24571=CARTESIAN_POINT('Ctrl Pts',(-40.6211886619977,36.4680712072204,37.4595702857772));
#24572=CARTESIAN_POINT('Ctrl Pts',(-40.64505188868,36.4845612106588,37.4897124359308));
#24573=CARTESIAN_POINT('Ctrl Pts',(-40.6687642825718,36.5015298204025,37.5197028216856));
#24574=CARTESIAN_POINT('Ctrl Pts',(-40.6924766764637,36.5184984301463,37.5496932074404));
#24575=CARTESIAN_POINT('Ctrl Pts',(-40.7160382372553,36.535945645973,37.5795318284044));
#24576=CARTESIAN_POINT('Ctrl Pts',(-40.7394415755142,36.5538659868465,37.6092093237936));
#24577=CARTESIAN_POINT('Ctrl Pts',(-40.7628449137732,36.5717863277199,37.6388868191827));
#24578=CARTESIAN_POINT('Ctrl Pts',(-40.7860900291939,36.5901797934051,37.6684031886092));
#24579=CARTESIAN_POINT('Ctrl Pts',(-40.8091696315152,36.6090406066902,37.6977491722927));
#24580=CARTESIAN_POINT('Ctrl Pts',(-40.8322492338366,36.6279014199752,37.7270951559761));
#24581=CARTESIAN_POINT('Ctrl Pts',(-40.8551633227623,36.647229580616,37.756270753536));
#24582=CARTESIAN_POINT('Ctrl Pts',(-40.8779047117461,36.667019018832,37.7852668119755));
#24583=CARTESIAN_POINT('Ctrl Pts',(-40.9006461007299,36.686808457048,37.814262870415));
#24584=CARTESIAN_POINT('Ctrl Pts',(-40.9232147894755,36.7070591725803,37.8430793893553));
#24585=CARTESIAN_POINT('Ctrl Pts',(-40.9456036996708,36.7277648068939,37.8717073283198));
#24586=CARTESIAN_POINT('Ctrl Pts',(-40.9679926098661,36.7484704412076,37.9003352672843));
#24587=CARTESIAN_POINT('Ctrl Pts',(-40.990201741214,36.7696309940287,37.9287746258959));
#24588=CARTESIAN_POINT('Ctrl Pts',(-41.0122241280291,36.7912398220261,37.9570164818294));
#24589=CARTESIAN_POINT('Ctrl Pts',(-41.0342465148442,36.8128486500235,37.9852583377631));
#24590=CARTESIAN_POINT('Ctrl Pts',(-41.0560821568389,36.8349057529144,38.0133026906496));
#24591=CARTESIAN_POINT('Ctrl Pts',(-41.0777242053154,36.8574042067308,38.0411407418964));
#24592=CARTESIAN_POINT('Ctrl Pts',(-41.099366253792,36.8799026605473,38.0689787931431));
#24593=CARTESIAN_POINT('Ctrl Pts',(-41.1208147084676,36.902842464995,38.0966105423863));
#24594=CARTESIAN_POINT('Ctrl Pts',(-41.1420628419104,36.9262164197978,38.1240273202634));
#24595=CARTESIAN_POINT('Ctrl Pts',(-41.1633109753531,36.9495903746006,38.1514440981405));
#24596=CARTESIAN_POINT('Ctrl Pts',(-41.1843587872853,36.9733984794528,38.1786459042931));
#24597=CARTESIAN_POINT('Ctrl Pts',(-41.2051996757437,36.997633262271,38.2056242040064));
#24598=CARTESIAN_POINT('Ctrl Pts',(-41.2260405642022,37.0218680450892,38.2326025037197));
#24599=CARTESIAN_POINT('Ctrl Pts',(-41.2466745289145,37.0465295055564,38.259357296641));
#24600=CARTESIAN_POINT('Ctrl Pts',(-41.2670950975103,37.0716099044525,38.2858801880361));
#24601=CARTESIAN_POINT('Ctrl Pts',(-41.2875156661062,37.0966903033485,38.3124030794313));
#24602=CARTESIAN_POINT('Ctrl Pts',(-41.3077228383188,37.1221896403453,38.3386940689535));
#24603=CARTESIAN_POINT('Ctrl Pts',(-41.3277102754144,37.1480999139227,38.3647449070954));
#24604=CARTESIAN_POINT('Ctrl Pts',(-41.34769771251,37.1740101875002,38.3907957452372));
#24605=CARTESIAN_POINT('Ctrl Pts',(-41.367465414229,37.2003313973215,38.41660643166));
#24606=CARTESIAN_POINT('Ctrl Pts',(-41.3870071794313,37.2270552845631,38.4421688672345));
#24607=CARTESIAN_POINT('Ctrl Pts',(-40.2393823361708,36.2635753108104,37.028954656999));
#24608=CARTESIAN_POINT('Ctrl Pts',(-40.2654318337543,36.2754942589355,37.061362837691));
#24609=CARTESIAN_POINT('Ctrl Pts',(-40.2913657242679,36.2879516667465,37.09366559612));
#24610=CARTESIAN_POINT('Ctrl Pts',(-40.3171753053395,36.3009433405593,37.1258520900638));
#24611=CARTESIAN_POINT('Ctrl Pts',(-40.3429619687014,36.3139234783688,37.1580100038952));
#24612=CARTESIAN_POINT('Ctrl Pts',(-40.3686245428996,36.3274369336001,37.1900518591446));
#24613=CARTESIAN_POINT('Ctrl Pts',(-40.3941544318464,36.3414791671208,37.2219669202645));
#24614=CARTESIAN_POINT('Ctrl Pts',(-40.4196843207932,36.3555214006416,37.2538819813845));
#24615=CARTESIAN_POINT('Ctrl Pts',(-40.4450815241101,36.3700924122414,37.2856702479001));
#24616=CARTESIAN_POINT('Ctrl Pts',(-40.4703375347057,36.3851873092645,37.3173210693114));
#24617=CARTESIAN_POINT('Ctrl Pts',(-40.4955935453012,36.4002822062877,37.3489718907226));
#24618=CARTESIAN_POINT('Ctrl Pts',(-40.5207083627977,36.415900988508,37.3804852665568));
#24619=CARTESIAN_POINT('Ctrl Pts',(-40.5456735746448,36.4320384129698,37.4118506384062));
#24620=CARTESIAN_POINT('Ctrl Pts',(-40.570638786492,36.4481758374317,37.4432160102556));
#24621=CARTESIAN_POINT('Ctrl Pts',(-40.5954543923197,36.4648319038938,37.4744333776537));
#24622=CARTESIAN_POINT('Ctrl Pts',(-40.62011207985,36.4820010226548,37.5054922813855));
#24623=CARTESIAN_POINT('Ctrl Pts',(-40.6447697673802,36.4991701414158,37.5365511851173));
#24624=CARTESIAN_POINT('Ctrl Pts',(-40.6692695362319,36.5168523122129,37.5674516247135));
#24625=CARTESIAN_POINT('Ctrl Pts',(-40.6936031798588,36.5350416022997,37.5981832470913));
#24626=CARTESIAN_POINT('Ctrl Pts',(-40.7179368234858,36.5532308923865,37.6289148694691));
#24627=CARTESIAN_POINT('Ctrl Pts',(-40.7421043415256,36.571927301491,37.6594776741706));
#24628=CARTESIAN_POINT('Ctrl Pts',(-40.7660976386655,36.5911245577982,37.6898614211653));
#24629=CARTESIAN_POINT('Ctrl Pts',(-40.7900909358055,36.6103218141056,37.7202451681601));
#24630=CARTESIAN_POINT('Ctrl Pts',(-40.8139100116979,36.630019917334,37.7504498569997));
#24631=CARTESIAN_POINT('Ctrl Pts',(-40.8375468876434,36.6502122607802,37.7804653675298));
#24632=CARTESIAN_POINT('Ctrl Pts',(-40.8611837635889,36.6704046042263,37.8104808780598));
#24633=CARTESIAN_POINT('Ctrl Pts',(-40.8846384392368,36.6910911875891,37.8403072098336));
#24634=CARTESIAN_POINT('Ctrl Pts',(-40.9079030578806,36.7122650737206,37.8699343693509));
#24635=CARTESIAN_POINT('Ctrl Pts',(-40.9311676765242,36.7334389598521,37.8995615288682));
#24636=CARTESIAN_POINT('Ctrl Pts',(-40.9542422378081,36.7551001484313,37.9289895156833));
#24637=CARTESIAN_POINT('Ctrl Pts',(-40.9771190122039,36.7772413764693,37.9582084695932));
#24638=CARTESIAN_POINT('Ctrl Pts',(-40.9999957865997,36.7993826045072,37.9874274235032));
#24639=CARTESIAN_POINT('Ctrl Pts',(-41.0226747737666,36.8220038716734,38.0164373440725));
#24640=CARTESIAN_POINT('Ctrl Pts',(-41.0451483765286,36.8450975939977,38.0452285109826));
#24641=CARTESIAN_POINT('Ctrl Pts',(-41.0676219792906,36.8681913163219,38.0740196778928));
#24642=CARTESIAN_POINT('Ctrl Pts',(-41.0898901973128,36.8917574934596,38.1025920907146));
#24643=CARTESIAN_POINT('Ctrl Pts',(-41.1119455708393,36.915788225523,38.1309361755002));
#24644=CARTESIAN_POINT('Ctrl Pts',(-41.1340009443657,36.9398189575865,38.1592802602858));
#24645=CARTESIAN_POINT('Ctrl Pts',(-41.1558434730678,36.9643142442173,38.1873960166126));
#24646=CARTESIAN_POINT('Ctrl Pts',(-41.177465839586,36.9892658748842,38.2152740232916));
#24647=CARTESIAN_POINT('Ctrl Pts',(-41.1990882061042,37.0142175055512,38.2431520299707));
#24648=CARTESIAN_POINT('Ctrl Pts',(-41.2204904101162,37.0396254798822,38.2707922865863));
#24649=CARTESIAN_POINT('Ctrl Pts',(-41.2416652815407,37.0654812821836,38.2981855309956));
#24650=CARTESIAN_POINT('Ctrl Pts',(-41.2628401529652,37.0913370844849,38.3255787754048));
#24651=CARTESIAN_POINT('Ctrl Pts',(-41.2837876914865,37.1176407143712,38.352725007199));
#24652=CARTESIAN_POINT('Ctrl Pts',(-41.3045008790847,37.1443833566698,38.379615129462));
#24653=CARTESIAN_POINT('Ctrl Pts',(-41.3252140666829,37.1711259989686,38.406505251725));
#24654=CARTESIAN_POINT('Ctrl Pts',(-41.3456929030499,37.1983076532818,38.4331392640561));
#24655=CARTESIAN_POINT('Ctrl Pts',(-41.3659305269077,37.2259192108402,38.4595082408353));
#24656=CARTESIAN_POINT('Ctrl Pts',(-40.1775226142824,36.2455460982534,36.9999832962673));
#24657=CARTESIAN_POINT('Ctrl Pts',(-40.2045330088359,36.2572679658112,37.0334615519984));
#24658=CARTESIAN_POINT('Ctrl Pts',(-40.2314256153529,36.2695647115615,37.0668335548053));
#24659=CARTESIAN_POINT('Ctrl Pts',(-40.2581908128651,36.2824319360754,37.1000873656423));
#24660=CARTESIAN_POINT('Ctrl Pts',(-40.2849322441245,36.2952877350911,37.1333116486391));
#24661=CARTESIAN_POINT('Ctrl Pts',(-40.3115464920889,36.3087129999843,37.1664179489049));
#24662=CARTESIAN_POINT('Ctrl Pts',(-40.3380240521681,36.3227029362742,37.1993944434065));
#24663=CARTESIAN_POINT('Ctrl Pts',(-40.3645016122471,36.3366928725642,37.2323709379081));
#24664=CARTESIAN_POINT('Ctrl Pts',(-40.3908424839922,36.351247480013,37.2652176260855));
#24665=CARTESIAN_POINT('Ctrl Pts',(-40.4170372605052,36.3663615608482,37.2979227776481));
#24666=CARTESIAN_POINT('Ctrl Pts',(-40.4432320370181,36.3814756416834,37.3306279292107));
#24667=CARTESIAN_POINT('Ctrl Pts',(-40.4692807178519,36.3971491956478,37.3631915436014));
#24668=CARTESIAN_POINT('Ctrl Pts',(-40.495174000398,36.4133766253454,37.3956019915952));
#24669=CARTESIAN_POINT('Ctrl Pts',(-40.5210672829441,36.4296040550429,37.4280124395889));
#24670=CARTESIAN_POINT('Ctrl Pts',(-40.5468051667636,36.4463853601978,37.4602697206352));
#24671=CARTESIAN_POINT('Ctrl Pts',(-40.5723784602946,36.4637145478324,37.4923623149318));
#24672=CARTESIAN_POINT('Ctrl Pts',(-40.5979517538256,36.481043735467,37.5244549092285));
#24673=CARTESIAN_POINT('Ctrl Pts',(-40.62336045662,36.4989208052812,37.5563828162238));
#24674=CARTESIAN_POINT('Ctrl Pts',(-40.6485954946484,36.517339372964,37.588134633731));
#24675=CARTESIAN_POINT('Ctrl Pts',(-40.6738305326767,36.5357579406467,37.6198864512383));
#24676=CARTESIAN_POINT('Ctrl Pts',(-40.6988919055097,36.5547180058848,37.6514621787174));
#24677=CARTESIAN_POINT('Ctrl Pts',(-40.7237706631572,36.5742127976047,37.682850539753));
#24678=CARTESIAN_POINT('Ctrl Pts',(-40.7486494208046,36.5937075893247,37.7142389007886));
#24679=CARTESIAN_POINT('Ctrl Pts',(-40.7733455628527,36.6137371071996,37.7454398948509));
#24680=CARTESIAN_POINT('Ctrl Pts',(-40.7978502697247,36.6342941982205,37.7764423793422));
#24681=CARTESIAN_POINT('Ctrl Pts',(-40.8223549765967,36.6548512892413,37.8074448638336));
#24682=CARTESIAN_POINT('Ctrl Pts',(-40.8466682478773,36.6759359530588,37.8382488382272));
#24683=CARTESIAN_POINT('Ctrl Pts',(-40.8707814007572,36.6975406598657,37.8688433017258));
#24684=CARTESIAN_POINT('Ctrl Pts',(-40.8948945536371,36.7191453666726,37.8994377652244));
#24685=CARTESIAN_POINT('Ctrl Pts',(-40.9188075876976,36.741270116097,37.9298227173039));
#24686=CARTESIAN_POINT('Ctrl Pts',(-40.9425119630467,36.763907006884,37.9599873068021));
#24687=CARTESIAN_POINT('Ctrl Pts',(-40.9662163383959,36.7865438976709,37.9901518963003));
#24688=CARTESIAN_POINT('Ctrl Pts',(-40.9897120546304,36.8096929294357,38.0200961227041));
#24689=CARTESIAN_POINT('Ctrl Pts',(-41.0129907208921,36.8333458351287,38.0498092922445));
#24690=CARTESIAN_POINT('Ctrl Pts',(-41.0362693871538,36.8569987408218,38.079522461785));
#24691=CARTESIAN_POINT('Ctrl Pts',(-41.0593310030467,36.8811555200408,38.1090045739568));
#24692=CARTESIAN_POINT('Ctrl Pts',(-41.0821673327396,36.905807545847,38.1382451000225));
#24693=CARTESIAN_POINT('Ctrl Pts',(-41.1050036624325,36.9304595716531,38.1674856260882));
#24694=CARTESIAN_POINT('Ctrl Pts',(-41.1276147055371,36.955606843627,38.1964845655505));
#24695=CARTESIAN_POINT('Ctrl Pts',(-41.149992387132,36.9812403811018,38.2252315622241));
#24696=CARTESIAN_POINT('Ctrl Pts',(-41.1723700687269,37.0068739185767,38.2539785588976));
#24697=CARTESIAN_POINT('Ctrl Pts',(-41.1945143884316,37.0329937211167,38.2824736122934));
#24698=CARTESIAN_POINT('Ctrl Pts',(-41.2164174380024,37.059590460742,38.3107065461755));
#24699=CARTESIAN_POINT('Ctrl Pts',(-41.2383204875732,37.0861872003675,38.3389394800575));
#24700=CARTESIAN_POINT('Ctrl Pts',(-41.2599822666375,37.1132608766259,38.3669102939456));
#24701=CARTESIAN_POINT('Ctrl Pts',(-41.2813950392781,37.1408018208876,38.3946089988215));
#24702=CARTESIAN_POINT('Ctrl Pts',(-41.3028078119186,37.1683427651494,38.4223077036974));
#24703=CARTESIAN_POINT('Ctrl Pts',(-41.3239715777718,37.1963509769467,38.4497342990905));
#24704=CARTESIAN_POINT('Ctrl Pts',(-41.3448787787706,37.2248164539041,38.4768789903345));
#24705=CARTESIAN_POINT('Ctrl Pts',(-40.115662892394,36.2275168856964,36.9710119355355));
#24706=CARTESIAN_POINT('Ctrl Pts',(-40.1436341839173,36.2390416726869,37.0055602663057));
#24707=CARTESIAN_POINT('Ctrl Pts',(-40.1714855064378,36.2511777563766,37.0400015134906));
#24708=CARTESIAN_POINT('Ctrl Pts',(-40.1992063203907,36.2639205315914,37.0743226412208));
#24709=CARTESIAN_POINT('Ctrl Pts',(-40.2269025195477,36.2766519918134,37.108613293383));
#24710=CARTESIAN_POINT('Ctrl Pts',(-40.2544684412783,36.2899890663684,37.1427840386652));
#24711=CARTESIAN_POINT('Ctrl Pts',(-40.2818936724897,36.3039267054276,37.1768219665485));
#24712=CARTESIAN_POINT('Ctrl Pts',(-40.3093189037011,36.3178643444868,37.2108598944317));
#24713=CARTESIAN_POINT('Ctrl Pts',(-40.3366034438743,36.3324025477847,37.2447650042708));
#24714=CARTESIAN_POINT('Ctrl Pts',(-40.3637369863047,36.3475358124319,37.2785244859848));
#24715=CARTESIAN_POINT('Ctrl Pts',(-40.390870528735,36.3626690770792,37.3122839676987));
#24716=CARTESIAN_POINT('Ctrl Pts',(-40.4178530729061,36.3783974027877,37.3458978206461));
#24717=CARTESIAN_POINT('Ctrl Pts',(-40.4446744261511,36.3947148377209,37.3793533447841));
#24718=CARTESIAN_POINT('Ctrl Pts',(-40.4714957793961,36.4110322726542,37.4128088689221));
#24719=CARTESIAN_POINT('Ctrl Pts',(-40.4981559412074,36.4279388165018,37.4461060636166));
#24720=CARTESIAN_POINT('Ctrl Pts',(-40.5246448407391,36.44542807301,37.4792323484781));
#24721=CARTESIAN_POINT('Ctrl Pts',(-40.5511337402709,36.4629173295182,37.5123586333397));
#24722=CARTESIAN_POINT('Ctrl Pts',(-40.5774513770083,36.4809892983495,37.5453140077341));
#24723=CARTESIAN_POINT('Ctrl Pts',(-40.603587809438,36.4996371436282,37.5780860203707));
#24724=CARTESIAN_POINT('Ctrl Pts',(-40.6297242418677,36.518284988907,37.6108580330073));
#24725=CARTESIAN_POINT('Ctrl Pts',(-40.6556794694938,36.5375087102787,37.6434466832641));
#24726=CARTESIAN_POINT('Ctrl Pts',(-40.6814436876488,36.5573010374112,37.6758396583406));
#24727=CARTESIAN_POINT('Ctrl Pts',(-40.7072079058038,36.5770933645438,37.7082326334171));
#24728=CARTESIAN_POINT('Ctrl Pts',(-40.7327811140074,36.5974542970652,37.7404299327021));
#24729=CARTESIAN_POINT('Ctrl Pts',(-40.7581536518059,36.6183761356608,37.7724193911547));
#24730=CARTESIAN_POINT('Ctrl Pts',(-40.7835261896044,36.6392979742563,37.8044088496072));
#24731=CARTESIAN_POINT('Ctrl Pts',(-40.8086980565178,36.6607807185286,37.8361904666208));
#24732=CARTESIAN_POINT('Ctrl Pts',(-40.8336597436339,36.6828162460109,37.8677522341008));
#24733=CARTESIAN_POINT('Ctrl Pts',(-40.8586214307499,36.7048517734931,37.8993140015807));
#24734=CARTESIAN_POINT('Ctrl Pts',(-40.8833729375871,36.7274400837625,37.9306559189246));
#24735=CARTESIAN_POINT('Ctrl Pts',(-40.9079049138896,36.7505726372986,37.961766144011));
#24736=CARTESIAN_POINT('Ctrl Pts',(-40.9324368901921,36.7737051908346,37.9928763690974));
#24737=CARTESIAN_POINT('Ctrl Pts',(-40.9567493354943,36.7973819871978,38.0237549013357));
#24738=CARTESIAN_POINT('Ctrl Pts',(-40.9808330652556,36.8215940762597,38.0543900735065));
#24739=CARTESIAN_POINT('Ctrl Pts',(-41.004916795017,36.8458061653216,38.0850252456773));
#24740=CARTESIAN_POINT('Ctrl Pts',(-41.0287718087805,36.8705535466221,38.115417057199));
#24741=CARTESIAN_POINT('Ctrl Pts',(-41.0523890946399,36.8958268661709,38.1455540245448));
#24742=CARTESIAN_POINT('Ctrl Pts',(-41.0760063804993,36.9211001857197,38.1756909918906));
#24743=CARTESIAN_POINT('Ctrl Pts',(-41.0993859380063,36.9468994430366,38.2055731144884));
#24744=CARTESIAN_POINT('Ctrl Pts',(-41.122518934678,36.9732148873195,38.2351891011565));
#24745=CARTESIAN_POINT('Ctrl Pts',(-41.1456519313497,36.9995303316023,38.2648050878245));
#24746=CARTESIAN_POINT('Ctrl Pts',(-41.168538366747,37.0263619623512,38.2941549380004));
#24747=CARTESIAN_POINT('Ctrl Pts',(-41.1911695944641,37.0536996393006,38.3232275613553));
#24748=CARTESIAN_POINT('Ctrl Pts',(-41.2138008221812,37.0810373162499,38.3523001847102));
#24749=CARTESIAN_POINT('Ctrl Pts',(-41.2361768417885,37.1088810388806,38.3810955806921));
#24750=CARTESIAN_POINT('Ctrl Pts',(-41.2582891994715,37.1372202851054,38.4096028681809));
#24751=CARTESIAN_POINT('Ctrl Pts',(-41.2804015571544,37.1655595313302,38.4381101556698));
#24752=CARTESIAN_POINT('Ctrl Pts',(-41.3022502524937,37.1943943006115,38.4663293341249));
#24753=CARTESIAN_POINT('Ctrl Pts',(-41.3238270306336,37.223713696968,38.4942497398337));
#24754=CARTESIAN_POINT('Ctrl Pts',(-40.0552080328795,36.2113706699628,36.9436917252841));
#24755=CARTESIAN_POINT('Ctrl Pts',(-40.0841050153821,36.2226541801109,36.9792689639886));
#24756=CARTESIAN_POINT('Ctrl Pts',(-40.1128805203379,36.2345857171285,37.0147390538272));
#24757=CARTESIAN_POINT('Ctrl Pts',(-40.1415230375772,36.2471604949643,37.0500878044519));
#24758=CARTESIAN_POINT('Ctrl Pts',(-40.1701401215908,36.2597241069812,37.0854051670272));
#24759=CARTESIAN_POINT('Ctrl Pts',(-40.1986244533505,36.27292981772,37.1206014050315));
#24760=CARTESIAN_POINT('Ctrl Pts',(-40.2269646594312,36.286772341823,37.1556624627514));
#24761=CARTESIAN_POINT('Ctrl Pts',(-40.255304865512,36.300614865926,37.1907235204712));
#24762=CARTESIAN_POINT('Ctrl Pts',(-40.2835009453131,36.3150942030985,37.2256493971632));
#24763=CARTESIAN_POINT('Ctrl Pts',(-40.3115416405743,36.3302045601569,37.2604261451727));
#24764=CARTESIAN_POINT('Ctrl Pts',(-40.3395823358355,36.3453149172154,37.2952028931822));
#24765=CARTESIAN_POINT('Ctrl Pts',(-40.3674676459623,36.3610562938383,37.3298305117718));
#24766=CARTESIAN_POINT('Ctrl Pts',(-40.3951864368229,36.3774223936394,37.3642951724522));
#24767=CARTESIAN_POINT('Ctrl Pts',(-40.4229052276836,36.3937884934405,37.3987598331327));
#24768=CARTESIAN_POINT('Ctrl Pts',(-40.4504574986905,36.4107793160717,37.4330615351731));
#24769=CARTESIAN_POINT('Ctrl Pts',(-40.4778322487034,36.4283880669659,37.4671865802606));
#24770=CARTESIAN_POINT('Ctrl Pts',(-40.5052069987162,36.4459968178601,37.501311625348));
#24771=CARTESIAN_POINT('Ctrl Pts',(-40.5324042271549,36.4642234966432,37.5352600127589));
#24772=CARTESIAN_POINT('Ctrl Pts',(-40.55941307463,36.4830608159865,37.5690181852644));
#24773=CARTESIAN_POINT('Ctrl Pts',(-40.5864219221051,36.5018981353298,37.6027763577698));
#24774=CARTESIAN_POINT('Ctrl Pts',(-40.6132423880441,36.5213460948331,37.636344314654));
#24775=CARTESIAN_POINT('Ctrl Pts',(-40.6398637634536,36.5413969202162,37.6697086505675));
#24776=CARTESIAN_POINT('Ctrl Pts',(-40.6664851388631,36.5614477455992,37.703072986481));
#24777=CARTESIAN_POINT('Ctrl Pts',(-40.6929074231786,36.5821014364361,37.7362337007163));
#24778=CARTESIAN_POINT('Ctrl Pts',(-40.7191200663288,36.603349737693,37.7691775504777));
#24779=CARTESIAN_POINT('Ctrl Pts',(-40.745332709479,36.6245980389499,37.8021214002391));
#24780=CARTESIAN_POINT('Ctrl Pts',(-40.7713357109083,36.6464409501754,37.8348483848281));
#24781=CARTESIAN_POINT('Ctrl Pts',(-40.7971186878659,36.6688697421607,37.8673454345476));
#24782=CARTESIAN_POINT('Ctrl Pts',(-40.8229016648234,36.691298534146,37.899842484267));
#24783=CARTESIAN_POINT('Ctrl Pts',(-40.8484646167628,36.7143132064151,37.932109598428));
#24784=CARTESIAN_POINT('Ctrl Pts',(-40.8737973365208,36.7379045625412,37.9641338908396));
#24785=CARTESIAN_POINT('Ctrl Pts',(-40.8991300562788,36.7614959186673,37.9961581832512));
#24786=CARTESIAN_POINT('Ctrl Pts',(-40.9242325433185,36.7856639581496,38.0279396532343));
#24787=CARTESIAN_POINT('Ctrl Pts',(-40.9490947741904,36.8103990246712,38.0594656083655));
#24788=CARTESIAN_POINT('Ctrl Pts',(-40.9739570050623,36.8351340911929,38.0909915634966));
#24789=CARTESIAN_POINT('Ctrl Pts',(-40.9985789792395,36.8604361842288,38.1222620031072));
#24790=CARTESIAN_POINT('Ctrl Pts',(-41.0229508649667,36.8862951952653,38.1532644386485));
#24791=CARTESIAN_POINT('Ctrl Pts',(-41.0473227506939,36.9121542063018,38.1842668741896));
#24792=CARTESIAN_POINT('Ctrl Pts',(-41.0714445474545,36.9385701347902,38.215001305004));
#24793=CARTESIAN_POINT('Ctrl Pts',(-41.0953066230155,36.9655324280727,38.2454554563619));
#24794=CARTESIAN_POINT('Ctrl Pts',(-41.1191686985763,36.9924947213551,38.2759096077198));
#24795=CARTESIAN_POINT('Ctrl Pts',(-41.1427710524317,37.0200033788596,38.3060834789756));
#24796=CARTESIAN_POINT('Ctrl Pts',(-41.1661042595398,37.0480474121905,38.3359650189942));
#24797=CARTESIAN_POINT('Ctrl Pts',(-41.1894374666479,37.0760914455213,38.3658465590128));
#24798=CARTESIAN_POINT('Ctrl Pts',(-41.2125015265139,37.1046708540836,38.3954357671606));
#24799=CARTESIAN_POINT('Ctrl Pts',(-41.2352872287921,37.1337742224959,38.4247208254941));
#24800=CARTESIAN_POINT('Ctrl Pts',(-41.2580729310703,37.1628775909081,38.4540058838276));
#24801=CARTESIAN_POINT('Ctrl Pts',(-41.2805802752775,37.192504918553,38.4829867917259));
#24802=CARTESIAN_POINT('Ctrl Pts',(-41.3028002730974,37.2226443721554,38.5116519738488));
#24803=CARTESIAN_POINT('Ctrl Pts',(-39.995899860225,36.196737685331,36.9177032409763));
#24804=CARTESIAN_POINT('Ctrl Pts',(-40.0256928412121,36.2077442217939,36.9542750213889));
#24805=CARTESIAN_POINT('Ctrl Pts',(-40.0553634771827,36.2194357452618,36.9907403169737));
#24806=CARTESIAN_POINT('Ctrl Pts',(-40.0848992390629,36.2318073184586,37.0270837294477));
#24807=CARTESIAN_POINT('Ctrl Pts',(-40.1144087745578,36.2441679062727,37.0633948706585));
#24808=CARTESIAN_POINT('Ctrl Pts',(-40.1437836746807,36.257207336354,37.0995843442551));
#24809=CARTESIAN_POINT('Ctrl Pts',(-40.1730115572085,36.2709201122706,37.1356368955084));
#24810=CARTESIAN_POINT('Ctrl Pts',(-40.2022394397364,36.2846328881872,37.1716894467616));
#24811=CARTESIAN_POINT('Ctrl Pts',(-40.2313203039765,36.2990190096142,37.2076050748172));
#24812=CARTESIAN_POINT('Ctrl Pts',(-40.2602418916486,36.3140724124571,37.2433686403783));
#24813=CARTESIAN_POINT('Ctrl Pts',(-40.2891634793206,36.3291258153,37.2791322059394));
#24814=CARTESIAN_POINT('Ctrl Pts',(-40.3179257897392,36.3448464992021,37.3147437081585));
#24815=CARTESIAN_POINT('Ctrl Pts',(-40.3465166989024,36.361227837519,37.3501881359354));
#24816=CARTESIAN_POINT('Ctrl Pts',(-40.3751076080657,36.3776091758358,37.3856325637123));
#24817=CARTESIAN_POINT('Ctrl Pts',(-40.4035271152963,36.3946511681793,37.4209099162071));
#24818=CARTESIAN_POINT('Ctrl Pts',(-40.4317632410912,36.4123466309417,37.4560053231714));
#24819=CARTESIAN_POINT('Ctrl Pts',(-40.4599993668862,36.430042093704,37.4911007301356));
#24820=CARTESIAN_POINT('Ctrl Pts',(-40.4880521105766,36.4483910264661,37.5260141907377));
#24821=CARTESIAN_POINT('Ctrl Pts',(-40.5159096472599,36.4673856947134,37.5607309881186));
#24822=CARTESIAN_POINT('Ctrl Pts',(-40.5437671839431,36.4863803629608,37.5954477854994));
#24823=CARTESIAN_POINT('Ctrl Pts',(-40.5714295129589,36.5060207662435,37.6299679188363));
#24824=CARTESIAN_POINT('Ctrl Pts',(-40.5988849739737,36.5262986256614,37.664276837067));
#24825=CARTESIAN_POINT('Ctrl Pts',(-40.6263404349885,36.5465764850793,37.6985857552976));
#24826=CARTESIAN_POINT('Ctrl Pts',(-40.6535890273516,36.567491800152,37.732683457609));
#24827=CARTESIAN_POINT('Ctrl Pts',(-40.6806192651293,36.5890357545737,37.7665555710037));
#24828=CARTESIAN_POINT('Ctrl Pts',(-40.7076495029071,36.6105797089953,37.8004276843984));
#24829=CARTESIAN_POINT('Ctrl Pts',(-40.7344613854591,36.6327523022554,37.8340742080738));
#24830=CARTESIAN_POINT('Ctrl Pts',(-40.7610436109349,36.6555441880753,37.8674809592147));
#24831=CARTESIAN_POINT('Ctrl Pts',(-40.7876258364107,36.6783360738951,37.9008877103557));
#24832=CARTESIAN_POINT('Ctrl Pts',(-40.8139784041806,36.7017472517346,37.9340546881708));
#24833=CARTESIAN_POINT('Ctrl Pts',(-40.8400902060065,36.7257678532221,37.9669679119851));
#24834=CARTESIAN_POINT('Ctrl Pts',(-40.8662020078325,36.7497884547095,37.9998811357994));
#24835=CARTESIAN_POINT('Ctrl Pts',(-40.8920730430959,36.7744184792757,38.032540604833));
#24836=CARTESIAN_POINT('Ctrl Pts',(-40.917692406536,36.799647544776,38.0649325523381));
#24837=CARTESIAN_POINT('Ctrl Pts',(-40.9433117699762,36.8248766102762,38.0973244998432));
#24838=CARTESIAN_POINT('Ctrl Pts',(-40.9686794609861,36.8507047161126,38.1294489250522));
#24839=CARTESIAN_POINT('Ctrl Pts',(-40.993784786477,36.8771209751204,38.1612922867512));
#24840=CARTESIAN_POINT('Ctrl Pts',(-41.018890111968,36.9035372341282,38.1931356484502));
#24841=CARTESIAN_POINT('Ctrl Pts',(-41.043733071345,36.9305416456815,38.2246979458846));
#24842=CARTESIAN_POINT('Ctrl Pts',(-41.0683031927061,36.9581228267747,38.2559658747907));
#24843=CARTESIAN_POINT('Ctrl Pts',(-41.0928733140672,36.9857040078678,38.2872338036968));
#24844=CARTESIAN_POINT('Ctrl Pts',(-41.1171705968302,37.0138619578471,38.3182073633337));
#24845=CARTESIAN_POINT('Ctrl Pts',(-41.1411847991091,37.0425848074629,38.3488734976047));
#24846=CARTESIAN_POINT('Ctrl Pts',(-41.1651990013879,37.0713076570786,38.3795396318758));
#24847=CARTESIAN_POINT('Ctrl Pts',(-41.1889301226135,37.1005954056502,38.4098983400543));
#24848=CARTESIAN_POINT('Ctrl Pts',(-41.2123681595503,37.1304357076907,38.4399368252183));
#24849=CARTESIAN_POINT('Ctrl Pts',(-41.2358061964872,37.1602760097311,38.4699753103823));
#24850=CARTESIAN_POINT('Ctrl Pts',(-41.2589511485798,37.1906688645334,38.49969357182));
#24851=CARTESIAN_POINT('Ctrl Pts',(-41.2817932596771,37.2216014607819,38.529079082573));
#24852=CARTESIAN_POINT('Ctrl Pts',(-39.9365916875705,36.1821047006991,36.8917147566685));
#24853=CARTESIAN_POINT('Ctrl Pts',(-39.9672806670422,36.192834263477,36.9292810787893));
#24854=CARTESIAN_POINT('Ctrl Pts',(-39.9978464340274,36.2042857733951,36.9667415801203));
#24855=CARTESIAN_POINT('Ctrl Pts',(-40.0282754405486,36.2164541419529,37.0040796544433));
#24856=CARTESIAN_POINT('Ctrl Pts',(-40.0586774275246,36.2286117055642,37.0413845742898));
#24857=CARTESIAN_POINT('Ctrl Pts',(-40.0889428960108,36.241484854988,37.0785672834787));
#24858=CARTESIAN_POINT('Ctrl Pts',(-40.1190584549858,36.2550678827182,37.1156113282653));
#24859=CARTESIAN_POINT('Ctrl Pts',(-40.1491740139607,36.2686509104485,37.152655373052));
#24860=CARTESIAN_POINT('Ctrl Pts',(-40.1791396626399,36.28294381613,37.1895607524711));
#24861=CARTESIAN_POINT('Ctrl Pts',(-40.2089421427228,36.2979402647574,37.2263111355838));
#24862=CARTESIAN_POINT('Ctrl Pts',(-40.2387446228058,36.3129367133846,37.2630615186965));
#24863=CARTESIAN_POINT('Ctrl Pts',(-40.268383933516,36.3286367045658,37.2996569045451));
#24864=CARTESIAN_POINT('Ctrl Pts',(-40.297846960982,36.3450332813984,37.3360810994186));
#24865=CARTESIAN_POINT('Ctrl Pts',(-40.3273099884479,36.3614298582311,37.372505294292));
#24866=CARTESIAN_POINT('Ctrl Pts',(-40.356596731902,36.3785230202869,37.4087582972411));
#24867=CARTESIAN_POINT('Ctrl Pts',(-40.3856942334791,36.3963051949174,37.4448240660821));
#24868=CARTESIAN_POINT('Ctrl Pts',(-40.4147917350561,36.4140873695479,37.4808898349232));
#24869=CARTESIAN_POINT('Ctrl Pts',(-40.4436999939984,36.4325585562889,37.5167683687165));
#24870=CARTESIAN_POINT('Ctrl Pts',(-40.4724062198898,36.4517105734403,37.5524437909728));
#24871=CARTESIAN_POINT('Ctrl Pts',(-40.5011124457811,36.4708625905918,37.588119213229));
#24872=CARTESIAN_POINT('Ctrl Pts',(-40.5296166378738,36.4906954376539,37.6235915230185));
#24873=CARTESIAN_POINT('Ctrl Pts',(-40.5579061844939,36.5112003311067,37.6588450235664));
#24874=CARTESIAN_POINT('Ctrl Pts',(-40.586195731114,36.5317052245595,37.6940985241142));
#24875=CARTESIAN_POINT('Ctrl Pts',(-40.6142706315245,36.5528821638678,37.7291332145017));
#24876=CARTESIAN_POINT('Ctrl Pts',(-40.6421184639298,36.5747217714543,37.7639335915297));
#24877=CARTESIAN_POINT('Ctrl Pts',(-40.6699662963352,36.5965613790407,37.7987339685576));
#24878=CARTESIAN_POINT('Ctrl Pts',(-40.6975870600099,36.6190636543355,37.8333000313194));
#24879=CARTESIAN_POINT('Ctrl Pts',(-40.724968534004,36.6422186339898,37.8676164838819));
#24880=CARTESIAN_POINT('Ctrl Pts',(-40.7523500079981,36.6653736136441,37.9019329364444));
#24881=CARTESIAN_POINT('Ctrl Pts',(-40.7794921915984,36.6891812970541,37.9359997779136));
#24882=CARTESIAN_POINT('Ctrl Pts',(-40.8063830754924,36.7136311439029,37.9698019331306));
#24883=CARTESIAN_POINT('Ctrl Pts',(-40.8332739593863,36.7380809907517,38.0036040883476));
#24884=CARTESIAN_POINT('Ctrl Pts',(-40.8599135428732,36.7631730004019,38.0371415564316));
#24885=CARTESIAN_POINT('Ctrl Pts',(-40.8862900388817,36.7888960648807,38.0703994963107));
#24886=CARTESIAN_POINT('Ctrl Pts',(-40.9126665348901,36.8146191293595,38.1036574361897));
#24887=CARTESIAN_POINT('Ctrl Pts',(-40.9387799427328,36.8409732479963,38.1366358469971));
#24888=CARTESIAN_POINT('Ctrl Pts',(-40.9646187079874,36.8679467549755,38.169320134854));
#24889=CARTESIAN_POINT('Ctrl Pts',(-40.990457473242,36.8949202619546,38.2020044227108));
#24890=CARTESIAN_POINT('Ctrl Pts',(-41.0160215952354,36.922513156573,38.2343945867653));
#24891=CARTESIAN_POINT('Ctrl Pts',(-41.0412997623967,36.9507132254767,38.2664762932196));
#24892=CARTESIAN_POINT('Ctrl Pts',(-41.066577929558,36.9789132943805,38.2985579996738));
#24893=CARTESIAN_POINT('Ctrl Pts',(-41.0915701412288,37.0077205368345,38.3303312476919));
#24894=CARTESIAN_POINT('Ctrl Pts',(-41.1162653386783,37.0371222027352,38.3617819762153));
#24895=CARTESIAN_POINT('Ctrl Pts',(-41.140960536128,37.0665238686359,38.3932327047388));
#24896=CARTESIAN_POINT('Ctrl Pts',(-41.1653587187131,37.0965199572167,38.4243609129481));
#24897=CARTESIAN_POINT('Ctrl Pts',(-41.1894490903085,37.1270971928855,38.4551528249425));
#24898=CARTESIAN_POINT('Ctrl Pts',(-41.2135394619039,37.1576744285542,38.485944736937));
#24899=CARTESIAN_POINT('Ctrl Pts',(-41.2373220218821,37.1888328105138,38.5164003519141));
#24900=CARTESIAN_POINT('Ctrl Pts',(-41.2607862462568,37.2205585494085,38.5465061912972));
#24901=CARTESIAN_POINT('Ctrl Pts',(-39.8784322174862,36.1689883085647,36.8670608120083));
#24902=CARTESIAN_POINT('Ctrl Pts',(-39.9099874630055,36.1794051227783,36.9055872530872));
#24903=CARTESIAN_POINT('Ctrl Pts',(-39.9414192696731,36.1905810749234,36.9440092667769));
#24904=CARTESIAN_POINT('Ctrl Pts',(-39.9727130222373,36.2025109548909,36.9823089854244));
#24905=CARTESIAN_POINT('Ctrl Pts',(-40.003978987402,36.2144302416788,37.0205746956998));
#24906=CARTESIAN_POINT('Ctrl Pts',(-40.0351071426304,36.2271021176342,37.0587183269245));
#24907=CARTESIAN_POINT('Ctrl Pts',(-40.0660830396764,36.2405206886271,37.0967221725232));
#24908=CARTESIAN_POINT('Ctrl Pts',(-40.0970589367223,36.25393925962,37.1347260181219));
#24909=CARTESIAN_POINT('Ctrl Pts',(-40.1278825746968,36.2681045252642,37.1725900770043));
#24910=CARTESIAN_POINT('Ctrl Pts',(-40.1585396467511,36.2830098989899,37.2102967724828));
#24911=CARTESIAN_POINT('Ctrl Pts',(-40.1891967188056,36.2979152727155,37.2480034679613));
#24912=CARTESIAN_POINT('Ctrl Pts',(-40.2196872240624,36.3135607540937,37.2855527989552));
#24913=CARTESIAN_POINT('Ctrl Pts',(-40.2499970104069,36.3299390702522,37.3229273349807));
#24914=CARTESIAN_POINT('Ctrl Pts',(-40.2803067967514,36.3463173864108,37.3603018710062));
#24915=CARTESIAN_POINT('Ctrl Pts',(-40.3104358633138,36.3634285368788,37.3975016109911));
#24916=CARTESIAN_POINT('Ctrl Pts',(-40.340370225743,36.3812645692036,37.4345092867707));
#24917=CARTESIAN_POINT('Ctrl Pts',(-40.3703045881721,36.3991006015286,37.4715169625502));
#24918=CARTESIAN_POINT('Ctrl Pts',(-40.4000442456191,36.417661515201,37.5083325730667));
#24919=CARTESIAN_POINT('Ctrl Pts',(-40.4295753945039,36.4369386855833,37.5449390284921));
#24920=CARTESIAN_POINT('Ctrl Pts',(-40.4591065433887,36.4562158559656,37.5815454839174));
#24921=CARTESIAN_POINT('Ctrl Pts',(-40.4884291828649,36.4762092825039,37.617942783202));
#24922=CARTESIAN_POINT('Ctrl Pts',(-40.5175297028907,36.4969096763675,37.6541140306777));
#24923=CARTESIAN_POINT('Ctrl Pts',(-40.5466302229165,36.5176100702311,37.6902852781534));
#24924=CARTESIAN_POINT('Ctrl Pts',(-40.5755086226514,36.5390174308226,37.7262304727808));
#24925=CARTESIAN_POINT('Ctrl Pts',(-40.6041514982105,36.5611218137356,37.7619329287079));
#24926=CARTESIAN_POINT('Ctrl Pts',(-40.6327943737695,36.5832261966487,37.797635384635));
#24927=CARTESIAN_POINT('Ctrl Pts',(-40.6612017243305,36.6060276012486,37.8330951008377));
#24928=CARTESIAN_POINT('Ctrl Pts',(-40.6893603645431,36.6295154367558,37.8682956167224));
#24929=CARTESIAN_POINT('Ctrl Pts',(-40.7175190047557,36.6530032722632,37.9034961326072));
#24930=CARTESIAN_POINT('Ctrl Pts',(-40.7454289338183,36.6771775380065,37.9384374471669));
#24931=CARTESIAN_POINT('Ctrl Pts',(-40.7730771971629,36.7020270066669,37.9731033403279));
#24932=CARTESIAN_POINT('Ctrl Pts',(-40.8007254605076,36.7268764753273,38.0077692334889));
#24933=CARTESIAN_POINT('Ctrl Pts',(-40.8281120573416,36.7524011461916,38.0421597042572));
#24934=CARTESIAN_POINT('Ctrl Pts',(-40.855224275867,36.7785891658016,38.0762587881));
#24935=CARTESIAN_POINT('Ctrl Pts',(-40.8823364943923,36.8047771854116,38.1103578719428));
#24936=CARTESIAN_POINT('Ctrl Pts',(-40.9091743338317,36.8316285530159,38.1441655678822));
#24937=CARTESIAN_POINT('Ctrl Pts',(-40.935725336931,36.8591308000021,38.1776661817153));
#24938=CARTESIAN_POINT('Ctrl Pts',(-40.9622763400304,36.8866330469883,38.2111667955484));
#24939=CARTESIAN_POINT('Ctrl Pts',(-40.9885405060285,36.9147861725675,38.2443603263144));
#24940=CARTESIAN_POINT('Ctrl Pts',(-41.0145056437539,36.9435771045273,38.2772313646783));
#24941=CARTESIAN_POINT('Ctrl Pts',(-41.0404707814793,36.9723680364872,38.3101024030422));
#24942=CARTESIAN_POINT('Ctrl Pts',(-41.0661368901876,37.0017967740017,38.3426509480614));
#24943=CARTESIAN_POINT('Ctrl Pts',(-41.0914920560819,37.0318496533715,38.3748618895438));
#24944=CARTESIAN_POINT('Ctrl Pts',(-41.1168472219763,37.0619025327413,38.4070728310262));
#24945=CARTESIAN_POINT('Ctrl Pts',(-41.1418914443299,37.0925795531042,38.4389461680483));
#24946=CARTESIAN_POINT('Ctrl Pts',(-41.1666130977562,37.1238664719334,38.4704671035589));
#24947=CARTESIAN_POINT('Ctrl Pts',(-41.1913347511826,37.1551533907627,38.5019880390694));
#24948=CARTESIAN_POINT('Ctrl Pts',(-41.2157338349727,37.1870502071607,38.5331565721646));
#24949=CARTESIAN_POINT('Ctrl Pts',(-41.2397990229199,37.219542112969,38.5639582326428));
#24950=CARTESIAN_POINT('Ctrl Pts',(-39.8212339521721,36.1571263872747,36.843513753304));
#24951=CARTESIAN_POINT('Ctrl Pts',(-39.8536297885598,36.1672007132204,36.8829707943146));
#24952=CARTESIAN_POINT('Ctrl Pts',(-39.8859025733484,36.1780715372741,36.922325499607));
#24953=CARTESIAN_POINT('Ctrl Pts',(-39.9180365787514,36.1897335612995,36.9615586900972));
#24954=CARTESIAN_POINT('Ctrl Pts',(-39.9501420506494,36.201385229989,37.0007570433356));
#24955=CARTESIAN_POINT('Ctrl Pts',(-39.9821089884994,36.2138266938084,37.0398340962383));
#24956=CARTESIAN_POINT('Ctrl Pts',(-40.0139218412059,36.2270519003014,37.0787708388032));
#24957=CARTESIAN_POINT('Ctrl Pts',(-40.0457346939124,36.2402771067946,37.1177075813681));
#24958=CARTESIAN_POINT('Ctrl Pts',(-40.0773934604703,36.2542860555442,37.1565040123657));
#24959=CARTESIAN_POINT('Ctrl Pts',(-40.1088827396594,36.2690719315407,37.1951412582926));
#24960=CARTESIAN_POINT('Ctrl Pts',(-40.1403720188486,36.2838578075371,37.2337785042195));
#24961=CARTESIAN_POINT('Ctrl Pts',(-40.1716918096762,36.2994206103136,37.2722565638567));
#24962=CARTESIAN_POINT('Ctrl Pts',(-40.2028268758645,36.3157527689609,37.310556718596));
#24963=CARTESIAN_POINT('Ctrl Pts',(-40.2339619420527,36.3320849276083,37.3488568733352));
#24964=CARTESIAN_POINT('Ctrl Pts',(-40.2649122826178,36.349186441611,37.386979121967));
#24965=CARTESIAN_POINT('Ctrl Pts',(-40.2956628409744,36.3670489915034,37.4249049189625));
#24966=CARTESIAN_POINT('Ctrl Pts',(-40.3264133993311,36.3849115413958,37.462830715958));
#24967=CARTESIAN_POINT('Ctrl Pts',(-40.3569641745175,36.4035351266172,37.5005600601234));
#24968=CARTESIAN_POINT('Ctrl Pts',(-40.387300304344,36.422910687258,37.5380745970745));
#24969=CARTESIAN_POINT('Ctrl Pts',(-40.4176364341705,36.4422862478988,37.5755891340256));
#24970=CARTESIAN_POINT('Ctrl Pts',(-40.4477579176795,36.4624137833476,37.6128888625783));
#24971=CARTESIAN_POINT('Ctrl Pts',(-40.4776501015213,36.4832835020608,37.6499556373456));
#24972=CARTESIAN_POINT('Ctrl Pts',(-40.5075422853631,36.5041532207739,37.687022412113));
#24973=CARTESIAN_POINT('Ctrl Pts',(-40.537205168588,36.52576512209,37.7238562319229));
#24974=CARTESIAN_POINT('Ctrl Pts',(-40.5666243209561,36.5481086923639,37.7604391780458));
#24975=CARTESIAN_POINT('Ctrl Pts',(-40.5960434733241,36.5704522626378,37.7970221241688));
#24976=CARTESIAN_POINT('Ctrl Pts',(-40.6252188939058,36.5935275011641,37.8333541954497));
#24977=CARTESIAN_POINT('Ctrl Pts',(-40.6541363895764,36.61732318241,37.8694177172388));
#24978=CARTESIAN_POINT('Ctrl Pts',(-40.683053885247,36.641118863656,37.9054812390279));
#24979=CARTESIAN_POINT('Ctrl Pts',(-40.7117134550993,36.6656349868731,37.941276210189));
#24980=CARTESIAN_POINT('Ctrl Pts',(-40.7401011569678,36.6908596255793,37.976785217362));
#24981=CARTESIAN_POINT('Ctrl Pts',(-40.7684888588364,36.7160842642856,38.0122942245349));
#24982=CARTESIAN_POINT('Ctrl Pts',(-40.7966046918253,36.7420174176848,38.0475172665991));
#24983=CARTESIAN_POINT('Ctrl Pts',(-40.8244349782834,36.7686464699451,38.0824372084235));
#24984=CARTESIAN_POINT('Ctrl Pts',(-40.8522652647416,36.7952755222055,38.117357150248));
#24985=CARTESIAN_POINT('Ctrl Pts',(-40.8798100037906,36.8226004724864,38.1519739907306));
#24986=CARTESIAN_POINT('Ctrl Pts',(-40.9070557956025,36.8506080278818,38.1862708896424));
#24987=CARTESIAN_POINT('Ctrl Pts',(-40.9343015874144,36.8786155832771,38.2205677885543));
#24988=CARTESIAN_POINT('Ctrl Pts',(-40.9612484311292,36.9073057429028,38.2545447448129));
#24989=CARTESIAN_POINT('Ctrl Pts',(-40.98788321778,36.9366645497122,38.2881852294771));
#24990=CARTESIAN_POINT('Ctrl Pts',(-41.0145180044308,36.9660233565217,38.3218257141413));
#24991=CARTESIAN_POINT('Ctrl Pts',(-41.040840733177,36.9960508095882,38.3551297261493));
#24992=CARTESIAN_POINT('Ctrl Pts',(-41.0668385986679,37.0267323013055,38.3880810639305));
#24993=CARTESIAN_POINT('Ctrl Pts',(-41.0928364641588,37.0574137930227,38.4210324017117));
#24994=CARTESIAN_POINT('Ctrl Pts',(-41.118509465574,37.0887493224222,38.4536310642261));
#24995=CARTESIAN_POINT('Ctrl Pts',(-41.143845113639,37.120723645551,38.485861193038));
#24996=CARTESIAN_POINT('Ctrl Pts',(-41.1691807617039,37.1526979686799,38.5180913218498));
#24997=CARTESIAN_POINT('Ctrl Pts',(-41.1941790556189,37.1853110845287,38.5499529159419));
#24998=CARTESIAN_POINT('Ctrl Pts',(-41.2188278343383,37.2185471276312,38.5814304754439));
#24999=CARTESIAN_POINT('Ctrl Pts',(-39.7640356868581,36.1452644659848,36.8199666945997));
#25000=CARTESIAN_POINT('Ctrl Pts',(-39.7972721141141,36.1549963036626,36.8603543355419));
#25001=CARTESIAN_POINT('Ctrl Pts',(-39.8303858770236,36.1655619996249,36.900641732437));
#25002=CARTESIAN_POINT('Ctrl Pts',(-39.8633601352655,36.1769561677082,36.9408083947699));
#25003=CARTESIAN_POINT('Ctrl Pts',(-39.8963051138968,36.1883402182992,36.9809393909714));
#25004=CARTESIAN_POINT('Ctrl Pts',(-39.9291108343684,36.2005512699824,37.0209498655521));
#25005=CARTESIAN_POINT('Ctrl Pts',(-39.9617606427354,36.2135831119758,37.0608195050832));
#25006=CARTESIAN_POINT('Ctrl Pts',(-39.9944104511025,36.2266149539692,37.1006891446142));
#25007=CARTESIAN_POINT('Ctrl Pts',(-40.0269043462439,36.2404675858242,37.1404179477271));
#25008=CARTESIAN_POINT('Ctrl Pts',(-40.0592258325677,36.2551339640915,37.1799857441024));
#25009=CARTESIAN_POINT('Ctrl Pts',(-40.0915473188916,36.2698003423587,37.2195535404778));
#25010=CARTESIAN_POINT('Ctrl Pts',(-40.12369639529,36.2852804665335,37.2589603287583));
#25011=CARTESIAN_POINT('Ctrl Pts',(-40.155656741322,36.3015664676697,37.2981861022112));
#25012=CARTESIAN_POINT('Ctrl Pts',(-40.1876170873539,36.3178524688058,37.3374118756642));
#25013=CARTESIAN_POINT('Ctrl Pts',(-40.2193887019217,36.3349443463432,37.3764566329429));
#25014=CARTESIAN_POINT('Ctrl Pts',(-40.2509554562059,36.3528334138032,37.4153005511544));
#25015=CARTESIAN_POINT('Ctrl Pts',(-40.2825222104901,36.3707224812631,37.4541444693658));
#25016=CARTESIAN_POINT('Ctrl Pts',(-40.3138841034159,36.3894087380334,37.4927875471801));
#25017=CARTESIAN_POINT('Ctrl Pts',(-40.345025214184,36.4088826889328,37.5312101656569));
#25018=CARTESIAN_POINT('Ctrl Pts',(-40.3761663249522,36.4283566398322,37.5696327841337));
#25019=CARTESIAN_POINT('Ctrl Pts',(-40.4070866524941,36.4486182841913,37.6078349419546));
#25020=CARTESIAN_POINT('Ctrl Pts',(-40.4377705001518,36.4696573277541,37.6457972440136));
#25021=CARTESIAN_POINT('Ctrl Pts',(-40.4684543478096,36.4906963713168,37.6837595460726));
#25022=CARTESIAN_POINT('Ctrl Pts',(-40.4989017145245,36.5125128133576,37.721481991065));
#25023=CARTESIAN_POINT('Ctrl Pts',(-40.5290971437017,36.5350955709923,37.7589454273838));
#25024=CARTESIAN_POINT('Ctrl Pts',(-40.5592925728788,36.5576783286271,37.7964088637025));
#25025=CARTESIAN_POINT('Ctrl Pts',(-40.5892360634811,36.5810274010797,37.8336132900617));
#25026=CARTESIAN_POINT('Ctrl Pts',(-40.6189124146098,36.6051309280642,37.8705398177552));
#25027=CARTESIAN_POINT('Ctrl Pts',(-40.6485887657384,36.6292344550487,37.9074663454486));
#25028=CARTESIAN_POINT('Ctrl Pts',(-40.6779979763803,36.6540924357396,37.9441149732111));
#25029=CARTESIAN_POINT('Ctrl Pts',(-40.7071251167728,36.6796922444917,37.980467094396));
#25030=CARTESIAN_POINT('Ctrl Pts',(-40.7362522571653,36.7052920532438,38.016819215581));
#25031=CARTESIAN_POINT('Ctrl Pts',(-40.765097326309,36.7316336891779,38.052874828941));
#25032=CARTESIAN_POINT('Ctrl Pts',(-40.7936456806999,36.7587037740886,38.0886156287471));
#25033=CARTESIAN_POINT('Ctrl Pts',(-40.8221940350909,36.7857738589993,38.1243564285532));
#25034=CARTESIAN_POINT('Ctrl Pts',(-40.8504456737495,36.813572391957,38.1597824135788));
#25035=CARTESIAN_POINT('Ctrl Pts',(-40.878386254274,36.8420852557614,38.1948755975695));
#25036=CARTESIAN_POINT('Ctrl Pts',(-40.9063268347985,36.8705981195658,38.2299687815601));
#25037=CARTESIAN_POINT('Ctrl Pts',(-40.9339563562299,36.8998253132381,38.2647291633114));
#25038=CARTESIAN_POINT('Ctrl Pts',(-40.9612607918061,36.9297519948971,38.2991390942759));
#25039=CARTESIAN_POINT('Ctrl Pts',(-40.9885652273823,36.9596786765562,38.3335490252404));
#25040=CARTESIAN_POINT('Ctrl Pts',(-41.0155445761664,36.9903048451747,38.3676085042373));
#25041=CARTESIAN_POINT('Ctrl Pts',(-41.0421851412539,37.0216149492393,38.4013002383173));
#25042=CARTESIAN_POINT('Ctrl Pts',(-41.0688257063413,37.0529250533041,38.4349919723972));
#25043=CARTESIAN_POINT('Ctrl Pts',(-41.0951274868181,37.0849190917401,38.468315960404));
#25044=CARTESIAN_POINT('Ctrl Pts',(-41.1210771295217,37.1175808191686,38.5012552825171));
#25045=CARTESIAN_POINT('Ctrl Pts',(-41.1470267722253,37.1502425465971,38.5341946046302));
#25046=CARTESIAN_POINT('Ctrl Pts',(-41.172624276265,37.1835719618968,38.5667492597192));
#25047=CARTESIAN_POINT('Ctrl Pts',(-41.1978566457567,37.2175521422934,38.598902718245));
#25048=CARTESIAN_POINT('Ctrl Pts',(-39.7077998441206,36.1346589387687,36.7975281492573));
#25049=CARTESIAN_POINT('Ctrl Pts',(-39.7418511624317,36.144018504291,36.8388168379438));
#25050=CARTESIAN_POINT('Ctrl Pts',(-39.7757808173037,36.1542494580266,36.8800080725771));
#25051=CARTESIAN_POINT('Ctrl Pts',(-39.8095708106025,36.1653463593505,36.9210800011996));
#25052=CARTESIAN_POINT('Ctrl Pts',(-39.8433307999561,36.1764334071412,36.9621154598563));
#25053=CARTESIAN_POINT('Ctrl Pts',(-39.8769513743958,36.1883848649453,37.0030318227539));
#25054=CARTESIAN_POINT('Ctrl Pts',(-39.910414731496,36.201194391942,37.0438074224316));
#25055=CARTESIAN_POINT('Ctrl Pts',(-39.9438780885963,36.2140039189387,37.0845830221094));
#25056=CARTESIAN_POINT('Ctrl Pts',(-39.9771842271081,36.227671514648,37.125217857045));
#25057=CARTESIAN_POINT('Ctrl Pts',(-40.0103155112345,36.2421899302918,37.165690409025));
#25058=CARTESIAN_POINT('Ctrl Pts',(-40.0434467953608,36.2567083459355,37.206162961005));
#25059=CARTESIAN_POINT('Ctrl Pts',(-40.076403223862,36.2720775809692,37.2464732285173));
#25060=CARTESIAN_POINT('Ctrl Pts',(-40.1091673462115,36.2882894863336,37.2865998653457));
#25061=CARTESIAN_POINT('Ctrl Pts',(-40.1419314685611,36.304501391698,37.3267265021742));
#25062=CARTESIAN_POINT('Ctrl Pts',(-40.1745032835359,36.3215559667863,37.3666695068207));
#25063=CARTESIAN_POINT('Ctrl Pts',(-40.206865544319,36.339444170883,37.4064077276318));
#25064=CARTESIAN_POINT('Ctrl Pts',(-40.2392278051021,36.3573323749797,37.4461459484429));
#25065=CARTESIAN_POINT('Ctrl Pts',(-40.2713805104875,36.3760542074162,37.4856793839357));
#25066=CARTESIAN_POINT('Ctrl Pts',(-40.3033066356117,36.3955997453937,37.5249870993869));
#25067=CARTESIAN_POINT('Ctrl Pts',(-40.335232760736,36.4151452833711,37.5642948148381));
#25068=CARTESIAN_POINT('Ctrl Pts',(-40.3669323044075,36.4355145261586,37.6033768087801));
#25069=CARTESIAN_POINT('Ctrl Pts',(-40.3983884817113,36.4566966793738,37.642212385552));
#25070=CARTESIAN_POINT('Ctrl Pts',(-40.4298446590152,36.477878832589,37.6810479623239));
#25071=CARTESIAN_POINT('Ctrl Pts',(-40.461057468776,36.4998738954397,37.7196371204753));
#25072=CARTESIAN_POINT('Ctrl Pts',(-40.4920103837744,36.5226702133831,37.7579594252896));
#25073=CARTESIAN_POINT('Ctrl Pts',(-40.5229632987728,36.5454665313265,37.7962817301039));
#25074=CARTESIAN_POINT('Ctrl Pts',(-40.5536563178532,36.5690641035108,37.8343371801503));
#25075=CARTESIAN_POINT('Ctrl Pts',(-40.5840731889565,36.5934504275596,37.8721056232587));
#25076=CARTESIAN_POINT('Ctrl Pts',(-40.6144900600598,36.6178367516085,37.9098740663671));
#25077=CARTESIAN_POINT('Ctrl Pts',(-40.6446307820518,36.6430118266113,37.9473555011279));
#25078=CARTESIAN_POINT('Ctrl Pts',(-40.6744793952223,36.6689623155878,37.9845300792268));
#25079=CARTESIAN_POINT('Ctrl Pts',(-40.7043280083928,36.6949128045642,38.0217046573258));
#25080=CARTESIAN_POINT('Ctrl Pts',(-40.7338845116276,36.7216387065447,38.058572377375));
#25081=CARTESIAN_POINT('Ctrl Pts',(-40.7631332544355,36.7491258640507,38.0951137159004));
#25082=CARTESIAN_POINT('Ctrl Pts',(-40.7923819972434,36.7766130215566,38.1316550544258));
#25083=CARTESIAN_POINT('Ctrl Pts',(-40.821322978534,36.8048614335622,38.1678700100637));
#25084=CARTESIAN_POINT('Ctrl Pts',(-40.8499408735779,36.8338561370629,38.2037394048213));
#25085=CARTESIAN_POINT('Ctrl Pts',(-40.8785587686217,36.8628508405637,38.239608799579));
#25086=CARTESIAN_POINT('Ctrl Pts',(-40.9068535763509,36.8925918344768,38.2751326321173));
#25087=CARTESIAN_POINT('Ctrl Pts',(-40.9348103140075,36.9230633661018,38.3102920902048));
#25088=CARTESIAN_POINT('Ctrl Pts',(-40.9627670516641,36.9535348977268,38.3454515482923));
#25089=CARTESIAN_POINT('Ctrl Pts',(-40.9903857182032,36.9847369659249,38.3802466306157));
#25090=CARTESIAN_POINT('Ctrl Pts',(-41.0176516886709,37.0166530449538,38.4146589105926));
#25091=CARTESIAN_POINT('Ctrl Pts',(-41.0449176591385,37.0485691239827,38.4490711905695));
#25092=CARTESIAN_POINT('Ctrl Pts',(-41.0718309325168,37.0811992126505,38.4831006669151));
#25093=CARTESIAN_POINT('Ctrl Pts',(-41.0983772571203,37.1145260296501,38.5167293181798));
#25094=CARTESIAN_POINT('Ctrl Pts',(-41.1249235817238,37.1478528466497,38.5503579694445));
#25095=CARTESIAN_POINT('Ctrl Pts',(-41.1511029565612,37.1818763907364,38.5835857943725));
#25096=CARTESIAN_POINT('Ctrl Pts',(-41.1769015182838,37.2165786433123,38.6163951957028));
#25097=CARTESIAN_POINT('Ctrl Pts',(-39.6523857950171,36.125116607414,36.776029662523));
#25098=CARTESIAN_POINT('Ctrl Pts',(-39.6872293819169,36.1340785824282,36.818193511888));
#25099=CARTESIAN_POINT('Ctrl Pts',(-39.7219528960408,36.1439495968667,36.860263368761));
#25100=CARTESIAN_POINT('Ctrl Pts',(-39.7565371387752,36.154724192588,36.9022159727179));
#25101=CARTESIAN_POINT('Ctrl Pts',(-39.7910906723076,36.1654892209686,36.9441313247103));
#25102=CARTESIAN_POINT('Ctrl Pts',(-39.8255051802735,36.1771562262313,36.9859296302228));
#25103=CARTESIAN_POINT('Ctrl Pts',(-39.85976166862,36.1897187691237,37.0275878199396));
#25104=CARTESIAN_POINT('Ctrl Pts',(-39.8940181569666,36.2022813120162,37.0692460096564));
#25105=CARTESIAN_POINT('Ctrl Pts',(-39.9281166243022,36.2157393920279,37.1107640818852));
#25106=CARTESIAN_POINT('Ctrl Pts',(-39.9620382510075,36.2300855813778,37.1521191219778));
#25107=CARTESIAN_POINT('Ctrl Pts',(-39.9959598777127,36.2444317707276,37.1934741620704));
#25108=CARTESIAN_POINT('Ctrl Pts',(-40.0297046624065,36.2596660688321,37.2346661683455));
#25109=CARTESIAN_POINT('Ctrl Pts',(-40.0632539806756,36.2757800675803,37.2756724061182));
#25110=CARTESIAN_POINT('Ctrl Pts',(-40.0968032989448,36.2918940663284,37.316678643891));
#25111=CARTESIAN_POINT('Ctrl Pts',(-40.1301571494261,36.3088877650658,37.3574991114952));
#25112=CARTESIAN_POINT('Ctrl Pts',(-40.1632971234634,36.3267517846313,37.3981112793026));
#25113=CARTESIAN_POINT('Ctrl Pts',(-40.1964370975007,36.3446158041968,37.43872344711));
#25114=CARTESIAN_POINT('Ctrl Pts',(-40.2293631937494,36.3633501438654,37.4791273134714));
#25115=CARTESIAN_POINT('Ctrl Pts',(-40.262057239643,36.3829444637826,37.5193005786902));
#25116=CARTESIAN_POINT('Ctrl Pts',(-40.2947512855366,36.4025387836998,37.559473843909));
#25117=CARTESIAN_POINT('Ctrl Pts',(-40.3272132797466,36.4229930830697,37.5994165063532));
#25118=CARTESIAN_POINT('Ctrl Pts',(-40.3594253058539,36.4442960727581,37.6391065208739));
#25119=CARTESIAN_POINT('Ctrl Pts',(-40.3916373319611,36.4655990624466,37.6787965353945));
#25120=CARTESIAN_POINT('Ctrl Pts',(-40.4235993886555,36.4877507415875,37.7182339003787));
#25121=CARTESIAN_POINT('Ctrl Pts',(-40.4552938354456,36.5107388842303,37.7573968495623));
#25122=CARTESIAN_POINT('Ctrl Pts',(-40.4869882822357,36.5337270268732,37.7965597987459));
#25123=CARTESIAN_POINT('Ctrl Pts',(-40.5184151178338,36.5575516320839,37.8354483305377));
#25124=CARTESIAN_POINT('Ctrl Pts',(-40.5495569971425,36.5821995505885,37.8740409815837));
#25125=CARTESIAN_POINT('Ctrl Pts',(-40.5806988764513,36.6068474690932,37.9126336326297));
#25126=CARTESIAN_POINT('Ctrl Pts',(-40.6115557982068,36.6323186998909,37.9509304013623));
#25127=CARTESIAN_POINT('Ctrl Pts',(-40.6421107318609,36.6585991849036,37.9889101510342));
#25128=CARTESIAN_POINT('Ctrl Pts',(-40.6726656655151,36.6848796699162,38.0268899007062));
#25129=CARTESIAN_POINT('Ctrl Pts',(-40.7029186098265,36.711969408076,38.0645526297744));
#25130=CARTESIAN_POINT('Ctrl Pts',(-40.7328528675943,36.7398534480183,38.1018775514305));
#25131=CARTESIAN_POINT('Ctrl Pts',(-40.762787125362,36.7677374879607,38.1392024730866));
#25132=CARTESIAN_POINT('Ctrl Pts',(-40.7924026953714,36.7964158285534,38.1761895858147));
#25133=CARTESIAN_POINT('Ctrl Pts',(-40.8216832321981,36.8258726416493,38.2128184756916));
#25134=CARTESIAN_POINT('Ctrl Pts',(-40.8509637690248,36.8553294547451,38.2494473655685));
#25135=CARTESIAN_POINT('Ctrl Pts',(-40.8799092714797,36.8855647391474,38.2857180311063));
#25136=CARTESIAN_POINT('Ctrl Pts',(-40.9085037639673,36.9165618074033,38.3216104538048));
#25137=CARTESIAN_POINT('Ctrl Pts',(-40.9370982564548,36.9475588756594,38.3575028765032));
#25138=CARTESIAN_POINT('Ctrl Pts',(-40.965341737812,36.979317726509,38.3930170549038));
#25139=CARTESIAN_POINT('Ctrl Pts',(-40.9932186199006,37.0118208316117,38.4281333880261));
#25140=CARTESIAN_POINT('Ctrl Pts',(-41.0210955019892,37.0443239367144,38.4632497211483));
#25141=CARTESIAN_POINT('Ctrl Pts',(-41.0486057836766,37.0775712947497,38.4979682075655));
#25142=CARTESIAN_POINT('Ctrl Pts',(-41.0757342814917,37.1115445558401,38.5322696854552));
#25143=CARTESIAN_POINT('Ctrl Pts',(-41.1028627793069,37.1455178169305,38.566571163345));
#25144=CARTESIAN_POINT('Ctrl Pts',(-41.1296094921476,37.1802169796957,38.6004556313137));
#25145=CARTESIAN_POINT('Ctrl Pts',(-41.1559596579721,37.2156228929789,38.6339043878506));
#25146=CARTESIAN_POINT('Ctrl Pts',(-39.5969717459136,36.1155742760594,36.7545311757887));
#25147=CARTESIAN_POINT('Ctrl Pts',(-39.6326076014021,36.1241386605654,36.7975701858321));
#25148=CARTESIAN_POINT('Ctrl Pts',(-39.6681249747779,36.1336497357067,36.8405186649448));
#25149=CARTESIAN_POINT('Ctrl Pts',(-39.7035034669478,36.1441020258255,36.8833519442363));
#25150=CARTESIAN_POINT('Ctrl Pts',(-39.7388505446591,36.154545034796,36.9261471895641));
#25151=CARTESIAN_POINT('Ctrl Pts',(-39.7740589861511,36.1659275875173,36.9688274376917));
#25152=CARTESIAN_POINT('Ctrl Pts',(-39.809108605744,36.1782431463054,37.0113682174476));
#25153=CARTESIAN_POINT('Ctrl Pts',(-39.8441582253369,36.1905587050936,37.0539089972035));
#25154=CARTESIAN_POINT('Ctrl Pts',(-39.8790490214964,36.2038072694078,37.0963103067254));
#25155=CARTESIAN_POINT('Ctrl Pts',(-39.9137609907805,36.2179812324638,37.1385478349306));
#25156=CARTESIAN_POINT('Ctrl Pts',(-39.9484729600646,36.2321551955198,37.1807853631357));
#25157=CARTESIAN_POINT('Ctrl Pts',(-39.983006100951,36.2472545566949,37.2228591081738));
#25158=CARTESIAN_POINT('Ctrl Pts',(-40.0173406151398,36.2632706488268,37.2647449468908));
#25159=CARTESIAN_POINT('Ctrl Pts',(-40.0516751293285,36.2792867409589,37.3066307856078));
#25160=CARTESIAN_POINT('Ctrl Pts',(-40.0858110153162,36.2962195633453,37.3483287161697));
#25161=CARTESIAN_POINT('Ctrl Pts',(-40.1197287026078,36.3140593983796,37.3898148309734));
#25162=CARTESIAN_POINT('Ctrl Pts',(-40.1536463898993,36.331899233414,37.4313009457772));
#25163=CARTESIAN_POINT('Ctrl Pts',(-40.1873458770115,36.3506460803144,37.472575243007));
#25164=CARTESIAN_POINT('Ctrl Pts',(-40.2208078436743,36.3702891821715,37.5136140579935));
#25165=CARTESIAN_POINT('Ctrl Pts',(-40.2542698103372,36.3899322840284,37.55465287298));
#25166=CARTESIAN_POINT('Ctrl Pts',(-40.2874942550859,36.4104716399808,37.5954562039263));
#25167=CARTESIAN_POINT('Ctrl Pts',(-40.3204621299964,36.4318954661425,37.6360006561957));
#25168=CARTESIAN_POINT('Ctrl Pts',(-40.353430004907,36.4533192923041,37.6765451084652));
#25169=CARTESIAN_POINT('Ctrl Pts',(-40.386141308535,36.4756275877353,37.7168306802822));
#25170=CARTESIAN_POINT('Ctrl Pts',(-40.4185772871168,36.4988075550775,37.7568342738351));
#25171=CARTESIAN_POINT('Ctrl Pts',(-40.4510132656987,36.5219875224197,37.796837867388));
#25172=CARTESIAN_POINT('Ctrl Pts',(-40.4831739178143,36.546039160657,37.8365594809252));
#25173=CARTESIAN_POINT('Ctrl Pts',(-40.5150408053285,36.5709486736174,37.8759763399087));
#25174=CARTESIAN_POINT('Ctrl Pts',(-40.5469076928428,36.5958581865779,37.9153931988922));
#25175=CARTESIAN_POINT('Ctrl Pts',(-40.5784808143618,36.6216255731705,37.9545053015968));
#25176=CARTESIAN_POINT('Ctrl Pts',(-40.6097420684995,36.6482360542194,37.9932902228416));
#25177=CARTESIAN_POINT('Ctrl Pts',(-40.6410033226373,36.6748465352682,38.0320751440866));
#25178=CARTESIAN_POINT('Ctrl Pts',(-40.6719527080254,36.7023001096073,38.0705328821738));
#25179=CARTESIAN_POINT('Ctrl Pts',(-40.702572480753,36.730581031986,38.1086413869606));
#25180=CARTESIAN_POINT('Ctrl Pts',(-40.7331922534806,36.7588619543647,38.1467498917474));
#25181=CARTESIAN_POINT('Ctrl Pts',(-40.7634824122088,36.7879702235447,38.1845091615657));
#25182=CARTESIAN_POINT('Ctrl Pts',(-40.7934255908184,36.8178891462356,38.2218975465619));
#25183=CARTESIAN_POINT('Ctrl Pts',(-40.823368769428,36.8478080689265,38.2592859315581));
#25184=CARTESIAN_POINT('Ctrl Pts',(-40.8529649666086,36.878537643818,38.2963034300953));
#25185=CARTESIAN_POINT('Ctrl Pts',(-40.882197213927,36.9100602487049,38.3329288174047));
#25186=CARTESIAN_POINT('Ctrl Pts',(-40.9114294612455,36.9415828535918,38.3695542047142));
#25187=CARTESIAN_POINT('Ctrl Pts',(-40.9402977574209,36.9738984870931,38.405787479192));
#25188=CARTESIAN_POINT('Ctrl Pts',(-40.9687855511304,37.0069886182696,38.4416078654595));
#25189=CARTESIAN_POINT('Ctrl Pts',(-40.9972733448399,37.0400787494461,38.477428251727));
#25190=CARTESIAN_POINT('Ctrl Pts',(-41.0253806348363,37.0739433768488,38.5128357482158));
#25191=CARTESIAN_POINT('Ctrl Pts',(-41.0530913058632,37.10856308203,38.5478100527307));
#25192=CARTESIAN_POINT('Ctrl Pts',(-41.0808019768901,37.1431827872113,38.5827843572455));
#25193=CARTESIAN_POINT('Ctrl Pts',(-41.1081160277341,37.1785575686551,38.6173254682549));
#25194=CARTESIAN_POINT('Ctrl Pts',(-41.1350177976604,37.2146671426455,38.6514135799984));
#25195=CARTESIAN_POINT('Ctrl Pts',(-39.5423802548784,36.107096302736,36.7339737388304));
#25196=CARTESIAN_POINT('Ctrl Pts',(-39.5787857407974,36.1152377518645,36.7778620020655));
#25197=CARTESIAN_POINT('Ctrl Pts',(-39.6150749250676,36.1243636643348,36.8216638675484));
#25198=CARTESIAN_POINT('Ctrl Pts',(-39.6512261654248,36.1344685839076,36.8653532108844));
#25199=CARTESIAN_POINT('Ctrl Pts',(-39.6873453051588,36.144564530781,36.9090037601118));
#25200=CARTESIAN_POINT('Ctrl Pts',(-39.7233267441435,36.1556377464239,36.9525419848725));
#25201=CARTESIAN_POINT('Ctrl Pts',(-39.7591490619367,36.1676816263223,36.9959419643159));
#25202=CARTESIAN_POINT('Ctrl Pts',(-39.7949713797299,36.1797255062207,37.0393419437593));
#25203=CARTESIAN_POINT('Ctrl Pts',(-39.8306345746389,36.1927400498046,37.0826036758357));
#25204=CARTESIAN_POINT('Ctrl Pts',(-39.8661174157609,36.2067174976021,37.125701404476));
#25205=CARTESIAN_POINT('Ctrl Pts',(-39.9016002568831,36.2206949453995,37.1687991331163));
#25206=CARTESIAN_POINT('Ctrl Pts',(-39.9369027425454,36.2356352967486,37.2117328562867));
#25207=CARTESIAN_POINT('Ctrl Pts',(-39.9720038567691,36.2515296464936,37.2544770133768));
#25208=CARTESIAN_POINT('Ctrl Pts',(-40.0071049709929,36.2674239962385,37.2972211704668));
#25209=CARTESIAN_POINT('Ctrl Pts',(-40.0420047121196,36.2842723436275,37.3397757594581));
#25210=CARTESIAN_POINT('Ctrl Pts',(-40.0766823039535,36.3020646483887,37.382115445547));
#25211=CARTESIAN_POINT('Ctrl Pts',(-40.1113598957873,36.31985695315,37.4244551316359));
#25212=CARTESIAN_POINT('Ctrl Pts',(-40.1458153367065,36.3385932144465,37.4665799128291));
#25213=CARTESIAN_POINT('Ctrl Pts',(-40.180028115093,36.3582622688683,37.5084647102876));
#25214=CARTESIAN_POINT('Ctrl Pts',(-40.2142408934795,36.37793132329,37.5503495077461));
#25215=CARTESIAN_POINT('Ctrl Pts',(-40.2482110077184,36.3985331699072,37.5919943194928));
#25216=CARTESIAN_POINT('Ctrl Pts',(-40.2819182351279,36.4200555354481,37.6333743524638));
#25217=CARTESIAN_POINT('Ctrl Pts',(-40.3156254625376,36.4415779009889,37.6747543854349));
#25218=CARTESIAN_POINT('Ctrl Pts',(-40.3490698015163,36.4640207844321,37.7158696376735));
#25219=CARTESIAN_POINT('Ctrl Pts',(-40.3822313423855,36.4873708172573,37.7566956313795));
#25220=CARTESIAN_POINT('Ctrl Pts',(-40.4153928832547,36.5107208500824,37.7975216250854));
#25221=CARTESIAN_POINT('Ctrl Pts',(-40.4482716244472,36.5349780311859,37.8380583583306));
#25222=CARTESIAN_POINT('Ctrl Pts',(-40.4808479928981,36.5601279126792,37.8782816976643));
#25223=CARTESIAN_POINT('Ctrl Pts',(-40.513424361349,36.5852777941724,37.9185050369981));
#25224=CARTESIAN_POINT('Ctrl Pts',(-40.5456983555303,36.6113203748713,37.9584149805247));
#25225=CARTESIAN_POINT('Ctrl Pts',(-40.5776507623225,36.638240144732,37.9979877678588));
#25226=CARTESIAN_POINT('Ctrl Pts',(-40.6096031691147,36.6651599145927,38.0375605551929));
#25227=CARTESIAN_POINT('Ctrl Pts',(-40.6412339870097,36.6929568723436,38.0767961844664));
#25228=CARTESIAN_POINT('Ctrl Pts',(-40.6725243856593,36.7216144642273,38.115671296607));
#25229=CARTESIAN_POINT('Ctrl Pts',(-40.703814784309,36.750272056111,38.1545464087476));
#25230=CARTESIAN_POINT('Ctrl Pts',(-40.7347647622311,36.779790280771,38.1930610019186));
#25231=CARTESIAN_POINT('Ctrl Pts',(-40.7653558942499,36.8101515604333,38.23119214614));
#25232=CARTESIAN_POINT('Ctrl Pts',(-40.7959470262687,36.8405128400955,38.2693232903614));
#25233=CARTESIAN_POINT('Ctrl Pts',(-40.8261793109386,36.8717171733253,38.3070709838326));
#25234=CARTESIAN_POINT('Ctrl Pts',(-40.8560347501336,36.9037459792209,38.3444127529239));
#25235=CARTESIAN_POINT('Ctrl Pts',(-40.8858901893285,36.9357747851167,38.3817545220151));
#25236=CARTESIAN_POINT('Ctrl Pts',(-40.9153687816438,36.9686280621686,38.4186903649647));
#25237=CARTESIAN_POINT('Ctrl Pts',(-40.944452977432,37.0022862484628,38.4551982912251));
#25238=CARTESIAN_POINT('Ctrl Pts',(-40.9735371732202,37.035944434757,38.4917062174854));
#25239=CARTESIAN_POINT('Ctrl Pts',(-41.0022269711084,37.0704075287042,38.5277862253329));
#25240=CARTESIAN_POINT('Ctrl Pts',(-41.0305052907871,37.1056550106378,38.5634168334495));
#25241=CARTESIAN_POINT('Ctrl Pts',(-41.0587836104657,37.1409024925713,38.5990474415661));
#25242=CARTESIAN_POINT('Ctrl Pts',(-41.0866504505995,37.1769343608268,38.6342286482694));
#25243=CARTESIAN_POINT('Ctrl Pts',(-41.1140892205275,37.2137291623881,38.6689395070162));
#25244=CARTESIAN_POINT('Ctrl Pts',(-39.4885029329456,36.0995357124289,36.7142288179568));
#25245=CARTESIAN_POINT('Ctrl Pts',(-39.5256578065064,36.1072322970532,36.7589432482088));
#25246=CARTESIAN_POINT('Ctrl Pts',(-39.5626991277534,36.1159511992982,36.8035760623136));
#25247=CARTESIAN_POINT('Ctrl Pts',(-39.5996039709717,36.1256870222641,36.8480996360113));
#25248=CARTESIAN_POINT('Ctrl Pts',(-39.6364760444026,36.135414200271,36.8925836748425));
#25249=CARTESIAN_POINT('Ctrl Pts',(-39.6732118801939,36.1461564933479,36.9369586649175));
#25250=CARTESIAN_POINT('Ctrl Pts',(-39.7097887820638,36.1579072646444,36.9811971902702));
#25251=CARTESIAN_POINT('Ctrl Pts',(-39.7463656839339,36.1696580359408,37.0254357156229));
#25252=CARTESIAN_POINT('Ctrl Pts',(-39.7827836500186,36.182417284859,37.0695377740005));
#25253=CARTESIAN_POINT('Ctrl Pts',(-39.8190201803537,36.1961771284081,37.113476118036));
#25254=CARTESIAN_POINT('Ctrl Pts',(-39.8552567106888,36.2099369719573,37.1574144620715));
#25255=CARTESIAN_POINT('Ctrl Pts',(-39.8913118034313,36.2246974094365,37.2011890895288));
#25256=CARTESIAN_POINT('Ctrl Pts',(-39.927163182874,36.2404493214864,37.2447729553587));
#25257=CARTESIAN_POINT('Ctrl Pts',(-39.9630145623167,36.2562012335362,37.2883568211886));
#25258=CARTESIAN_POINT('Ctrl Pts',(-39.9986622266328,36.2729446193549,37.3317499231716));
#25259=CARTESIAN_POINT('Ctrl Pts',(-40.0340841517748,36.2906691344516,37.3749254519539));
#25260=CARTESIAN_POINT('Ctrl Pts',(-40.0695060769167,36.3083936495484,37.4181009807362));
#25261=CARTESIAN_POINT('Ctrl Pts',(-40.1047022610957,36.3270992930248,37.4610589341247));
#25262=CARTESIAN_POINT('Ctrl Pts',(-40.1396509592288,36.3467745080664,37.5037727716212));
#25263=CARTESIAN_POINT('Ctrl Pts',(-40.1745996573619,36.366449723108,37.5464866091177));
#25264=CARTESIAN_POINT('Ctrl Pts',(-40.2093008676697,36.3870945087132,37.5889563285476));
#25265=CARTESIAN_POINT('Ctrl Pts',(-40.2437331508764,36.4086961100169,37.6311556910557));
#25266=CARTESIAN_POINT('Ctrl Pts',(-40.2781654340831,36.4302977113206,37.6733550535639));
#25267=CARTESIAN_POINT('Ctrl Pts',(-40.3123287884256,36.4528561272191,37.7152840569987));
#25268=CARTESIAN_POINT('Ctrl Pts',(-40.3462021069497,36.4763574205668,37.7569167965795));
#25269=CARTESIAN_POINT('Ctrl Pts',(-40.3800754254738,36.4998587139144,37.7985495361603));
#25270=CARTESIAN_POINT('Ctrl Pts',(-40.4136587064533,36.5243028835146,37.8398860097669));
#25271=CARTESIAN_POINT('Ctrl Pts',(-40.4469312012788,36.54967482714,37.8809006786862));
#25272=CARTESIAN_POINT('Ctrl Pts',(-40.4802036961043,36.5750467707654,37.9219153476056));
#25273=CARTESIAN_POINT('Ctrl Pts',(-40.5131654030913,36.6013464871283,37.9626082097524));
#25274=CARTESIAN_POINT('Ctrl Pts',(-40.5457959576725,36.6285577276059,38.0029541240585));
#25275=CARTESIAN_POINT('Ctrl Pts',(-40.5784265122537,36.6557689680836,38.0433000383647));
#25276=CARTESIAN_POINT('Ctrl Pts',(-40.6107259127679,36.6838917312907,38.083299002776));
#25277=CARTESIAN_POINT('Ctrl Pts',(-40.6426742038376,36.7129086422805,38.1229263049318));
#25278=CARTESIAN_POINT('Ctrl Pts',(-40.6746224949072,36.7419255532703,38.1625536070876));
#25279=CARTESIAN_POINT('Ctrl Pts',(-40.7062196749005,36.7718366105629,38.2018092449689));
#25280=CARTESIAN_POINT('Ctrl Pts',(-40.7374462223,36.8026233343645,38.2406689654636));
#25281=CARTESIAN_POINT('Ctrl Pts',(-40.7686727696995,36.833410058166,38.2795286859583));
#25282=CARTESIAN_POINT('Ctrl Pts',(-40.7995286829138,36.8650724469085,38.3179924870875));
#25283=CARTESIAN_POINT('Ctrl Pts',(-40.8299948983795,36.8975909387715,38.3560366049504));
#25284=CARTESIAN_POINT('Ctrl Pts',(-40.8604611138452,36.9301094306343,38.3940807228133));
#25285=CARTESIAN_POINT('Ctrl Pts',(-40.8905376300156,36.9634840239645,38.4317051554743));
#25286=CARTESIAN_POINT('Ctrl Pts',(-40.9202058648666,36.9976940991033,38.4688866576175));
#25287=CARTESIAN_POINT('Ctrl Pts',(-40.9498740997176,37.0319041742421,38.5060681597608));
#25288=CARTESIAN_POINT('Ctrl Pts',(-40.9791340517388,37.0669497294479,38.5428067294934));
#25289=CARTESIAN_POINT('Ctrl Pts',(-41.0079676433999,37.1028091126999,38.579079668808));
#25290=CARTESIAN_POINT('Ctrl Pts',(-41.0368012350609,37.1386684959519,38.6153526081226));
#25291=CARTESIAN_POINT('Ctrl Pts',(-41.0652084648935,37.1753417054242,38.6511599151723));
#25292=CARTESIAN_POINT('Ctrl Pts',(-41.0931717822014,37.2128060834914,38.6864794673074));
#25293=CARTESIAN_POINT('Ctrl Pts',(-39.4346256110129,36.0919751221218,36.6944838970834));
#25294=CARTESIAN_POINT('Ctrl Pts',(-39.4725298722153,36.0992268422418,36.7400244943522));
#25295=CARTESIAN_POINT('Ctrl Pts',(-39.5103233304392,36.1075387342617,36.7854882570788));
#25296=CARTESIAN_POINT('Ctrl Pts',(-39.5479817765187,36.1169054606204,36.8308460611382));
#25297=CARTESIAN_POINT('Ctrl Pts',(-39.5856067836463,36.126263869761,36.8761635895733));
#25298=CARTESIAN_POINT('Ctrl Pts',(-39.6230970162442,36.1366752402719,36.9213753449624));
#25299=CARTESIAN_POINT('Ctrl Pts',(-39.660428502191,36.1481329029665,36.9664524162245));
#25300=CARTESIAN_POINT('Ctrl Pts',(-39.6977599881378,36.159590565661,37.0115294874866));
#25301=CARTESIAN_POINT('Ctrl Pts',(-39.7349327253984,36.1720945199135,37.0564718721653));
#25302=CARTESIAN_POINT('Ctrl Pts',(-39.7719229449465,36.1856367592142,37.101250831596));
#25303=CARTESIAN_POINT('Ctrl Pts',(-39.8089131644947,36.199178998515,37.1460297910268));
#25304=CARTESIAN_POINT('Ctrl Pts',(-39.8457208643172,36.2137595221243,37.1906453227709));
#25305=CARTESIAN_POINT('Ctrl Pts',(-39.8823225089789,36.2293689964792,37.2350688973405));
#25306=CARTESIAN_POINT('Ctrl Pts',(-39.9189241536405,36.244978470834,37.2794924719103));
#25307=CARTESIAN_POINT('Ctrl Pts',(-39.955319741146,36.2616168950825,37.323724086885));
#25308=CARTESIAN_POINT('Ctrl Pts',(-39.991485999596,36.2792736205146,37.3677354583607));
#25309=CARTESIAN_POINT('Ctrl Pts',(-40.0276522580461,36.2969303459467,37.4117468298364));
#25310=CARTESIAN_POINT('Ctrl Pts',(-40.0635891854849,36.315605371603,37.4555379554203));
#25311=CARTESIAN_POINT('Ctrl Pts',(-40.0992738033646,36.3352867472645,37.4990808329548));
#25312=CARTESIAN_POINT('Ctrl Pts',(-40.1349584212442,36.354968122926,37.5426237104893));
#25313=CARTESIAN_POINT('Ctrl Pts',(-40.170390727621,36.3756558475192,37.5859183376024));
#25314=CARTESIAN_POINT('Ctrl Pts',(-40.2055480666248,36.3973366845857,37.6289370296476));
#25315=CARTESIAN_POINT('Ctrl Pts',(-40.2407054056287,36.4190175216522,37.6719557216929));
#25316=CARTESIAN_POINT('Ctrl Pts',(-40.2755877753349,36.441691470006,37.7146984763238));
#25317=CARTESIAN_POINT('Ctrl Pts',(-40.310172871514,36.4653440238763,37.7571379617795));
#25318=CARTESIAN_POINT('Ctrl Pts',(-40.344757967693,36.4889965777465,37.7995774472352));
#25319=CARTESIAN_POINT('Ctrl Pts',(-40.3790457884594,36.5136277358433,37.8417136612032));
#25320=CARTESIAN_POINT('Ctrl Pts',(-40.4130144096595,36.5392217416009,37.8835196597081));
#25321=CARTESIAN_POINT('Ctrl Pts',(-40.4469830308596,36.5648157473584,37.925325658213));
#25322=CARTESIAN_POINT('Ctrl Pts',(-40.4806324506522,36.5913725993853,37.9668014389802));
#25323=CARTESIAN_POINT('Ctrl Pts',(-40.5139411530224,36.6188753104799,38.0079204802583));
#25324=CARTESIAN_POINT('Ctrl Pts',(-40.5472498553926,36.6463780215745,38.0490395215364));
#25325=CARTESIAN_POINT('Ctrl Pts',(-40.5802178385262,36.6748265902378,38.0898018210857));
#25326=CARTESIAN_POINT('Ctrl Pts',(-40.6128240220158,36.7042028203337,38.1301813132566));
#25327=CARTESIAN_POINT('Ctrl Pts',(-40.6454302055053,36.7335790504297,38.1705608054276));
#25328=CARTESIAN_POINT('Ctrl Pts',(-40.6776745875699,36.7638829403548,38.2105574880192));
#25329=CARTESIAN_POINT('Ctrl Pts',(-40.7095365503501,36.7950951082957,38.2501457847872));
#25330=CARTESIAN_POINT('Ctrl Pts',(-40.7413985131303,36.8263072762366,38.2897340815552));
#25331=CARTESIAN_POINT('Ctrl Pts',(-40.7728780548889,36.8584277204919,38.3289139903424));
#25332=CARTESIAN_POINT('Ctrl Pts',(-40.8039550466254,36.8914358983219,38.367660456977));
#25333=CARTESIAN_POINT('Ctrl Pts',(-40.8350320383618,36.9244440761519,38.4064069236116));
#25334=CARTESIAN_POINT('Ctrl Pts',(-40.8657064783874,36.9583399857604,38.4447199459838));
#25335=CARTESIAN_POINT('Ctrl Pts',(-40.8959587523012,36.9931019497439,38.48257502401));
#25336=CARTESIAN_POINT('Ctrl Pts',(-40.9262110262151,37.0278639137272,38.5204301020362));
#25337=CARTESIAN_POINT('Ctrl Pts',(-40.9560411323692,37.0634919301915,38.5578272336539));
#25338=CARTESIAN_POINT('Ctrl Pts',(-40.9854299960126,37.0999632147619,38.5947425041665));
#25339=CARTESIAN_POINT('Ctrl Pts',(-41.0148188596561,37.1364344993323,38.631657774679));
#25340=CARTESIAN_POINT('Ctrl Pts',(-41.0437664791875,37.1737490500216,38.6680911820752));
#25341=CARTESIAN_POINT('Ctrl Pts',(-41.0722543438753,37.2118830045948,38.7040194275986));
#25342=CARTESIAN_POINT('Ctrl Pts',(-39.3814629558515,36.0853326504592,36.6755521234339));
#25343=CARTESIAN_POINT('Ctrl Pts',(-39.4200963515739,36.0921175602388,36.7218957884221));
#25344=CARTESIAN_POINT('Ctrl Pts',(-39.4586222625692,36.1000005779042,36.7681680489437));
#25345=CARTESIAN_POINT('Ctrl Pts',(-39.497015155909,36.1089764651429,36.814338236632));
#25346=CARTESIAN_POINT('Ctrl Pts',(-39.5353739581419,36.1179443822105,36.8604674273371));
#25347=CARTESIAN_POINT('Ctrl Pts',(-39.5735999766239,36.1280032283558,36.9064947237168));
#25348=CARTESIAN_POINT('Ctrl Pts',(-39.6116679223089,36.139146336545,36.9523896741349));
#25349=CARTESIAN_POINT('Ctrl Pts',(-39.6497358679937,36.1502894447343,36.9982846245528));
#25350=CARTESIAN_POINT('Ctrl Pts',(-39.6876457386624,36.1625168143152,37.0440472263331));
#25351=CARTESIAN_POINT('Ctrl Pts',(-39.7253724546258,36.1758203444221,37.0896472031976));
#25352=CARTESIAN_POINT('Ctrl Pts',(-39.7630991705892,36.189123874529,37.1352471800621));
#25353=CARTESIAN_POINT('Ctrl Pts',(-39.8006427296317,36.2035035643805,37.1806845293466));
#25354=CARTESIAN_POINT('Ctrl Pts',(-39.8379782945584,36.2189498900012,37.2259291901463));
#25355=CARTESIAN_POINT('Ctrl Pts',(-39.8753138594851,36.234396215622,37.2711738509459));
#25356=CARTESIAN_POINT('Ctrl Pts',(-39.9124414281179,36.2509091761096,37.3162258206219));
#25357=CARTESIAN_POINT('Ctrl Pts',(-39.9493364385308,36.2684778369691,37.3610552933582));
#25358=CARTESIAN_POINT('Ctrl Pts',(-39.9862314489437,36.2860464978287,37.4058847660944));
#25359=CARTESIAN_POINT('Ctrl Pts',(-40.0228938989954,36.3046708580366,37.4504917392803));
#25360=CARTESIAN_POINT('Ctrl Pts',(-40.0592995345528,36.3243385870607,37.4948467016043));
#25361=CARTESIAN_POINT('Ctrl Pts',(-40.0957051701101,36.3440063160846,37.5392016639285));
#25362=CARTESIAN_POINT('Ctrl Pts',(-40.1318539890504,36.3647174127763,37.5833046128045));
#25363=CARTESIAN_POINT('Ctrl Pts',(-40.1677220770696,36.3864581668707,37.6271263704259));
#25364=CARTESIAN_POINT('Ctrl Pts',(-40.2035901650887,36.4081989209652,37.6709481280473));
#25365=CARTESIAN_POINT('Ctrl Pts',(-40.2391775200882,36.4309693311908,37.7144886918567));
#25366=CARTESIAN_POINT('Ctrl Pts',(-40.2744605992144,36.4547543256888,37.7577192561222));
#25367=CARTESIAN_POINT('Ctrl Pts',(-40.3097436783406,36.4785393201868,37.8009498203877));
#25368=CARTESIAN_POINT('Ctrl Pts',(-40.344722479535,36.5033388975689,37.843870382588));
#25369=CARTESIAN_POINT('Ctrl Pts',(-40.3793738624689,36.5291366442977,37.8864525471272));
#25370=CARTESIAN_POINT('Ctrl Pts',(-40.4140252454028,36.5549343910266,37.9290347116664));
#25371=CARTESIAN_POINT('Ctrl Pts',(-40.4483492080622,36.5817303055995,37.9712784760635));
#25372=CARTESIAN_POINT('Ctrl Pts',(-40.4823230432667,36.6095066545203,38.0131558924017));
#25373=CARTESIAN_POINT('Ctrl Pts',(-40.5162968784713,36.6372830034411,38.0550333087399));
#25374=CARTESIAN_POINT('Ctrl Pts',(-40.5499205842402,36.6660397850891,38.0965443745774));
#25375=CARTESIAN_POINT('Ctrl Pts',(-40.5831719165406,36.6957579694511,38.1376616266135));
#25376=CARTESIAN_POINT('Ctrl Pts',(-40.616423248841,36.7254761538132,38.1787788786495));
#25377=CARTESIAN_POINT('Ctrl Pts',(-40.6493022057342,36.7561557391554,38.2195023144866));
#25378=CARTESIAN_POINT('Ctrl Pts',(-40.6817870357346,36.7877764241078,38.2598049917394));
#25379=CARTESIAN_POINT('Ctrl Pts',(-40.714271865735,36.8193971090602,38.3001076689922));
#25380=CARTESIAN_POINT('Ctrl Pts',(-40.7463625669486,36.851958891778,38.3399895853106));
#25381=CARTESIAN_POINT('Ctrl Pts',(-40.7780379091856,36.8854402263731,38.3794243548364));
#25382=CARTESIAN_POINT('Ctrl Pts',(-40.8097132514226,36.9189215609682,38.4188591243623));
#25383=CARTESIAN_POINT('Ctrl Pts',(-40.8409732328363,36.9533224454876,38.457846744796));
#25384=CARTESIAN_POINT('Ctrl Pts',(-40.8717971725931,36.9886201180083,38.4963614216827));
#25385=CARTESIAN_POINT('Ctrl Pts',(-40.9026211123499,37.023917790529,38.5348760985694));
#25386=CARTESIAN_POINT('Ctrl Pts',(-40.9330090086526,37.0601122489923,38.572917829663));
#25387=CARTESIAN_POINT('Ctrl Pts',(-40.9629407573583,37.0971795455297,38.6104614460067));
#25388=CARTESIAN_POINT('Ctrl Pts',(-40.992872506064,37.134246842067,38.6480050623504));
#25389=CARTESIAN_POINT('Ctrl Pts',(-41.0223481054269,37.1721869745165,38.6850505617546));
#25390=CARTESIAN_POINT('Ctrl Pts',(-41.0513480545682,37.2109748407208,38.7215734340293));
#25391=CARTESIAN_POINT('Ctrl Pts',(-39.328929483429,36.0794935374574,36.6573329044902));
#25392=CARTESIAN_POINT('Ctrl Pts',(-39.368273666578,36.0857923759536,36.7044587632537));
#25393=CARTESIAN_POINT('Ctrl Pts',(-39.4075142338028,36.0932273061387,36.7515192758672));
#25394=CARTESIAN_POINT('Ctrl Pts',(-39.446624290186,36.1017932315173,36.7984821877224));
#25395=CARTESIAN_POINT('Ctrl Pts',(-39.4856996186549,36.1103515507519,36.8454033986921));
#25396=CARTESIAN_POINT('Ctrl Pts',(-39.5246446655334,36.1200388569976,36.8922271792333));
#25397=CARTESIAN_POINT('Ctrl Pts',(-39.5634327857681,36.1308485224857,36.9389214939046));
#25398=CARTESIAN_POINT('Ctrl Pts',(-39.6022209060027,36.1416581879739,36.9856158085758));
#25399=CARTESIAN_POINT('Ctrl Pts',(-39.6408520971723,36.1535902120295,37.0321806544619));
#25400=CARTESIAN_POINT('Ctrl Pts',(-39.6792999289752,36.1666364311187,37.078584173284));
#25401=CARTESIAN_POINT('Ctrl Pts',(-39.7177477607781,36.1796826502079,37.124987692106));
#25402=CARTESIAN_POINT('Ctrl Pts',(-39.7560122307984,36.1938430635127,37.1712298809617));
#25403=CARTESIAN_POINT('Ctrl Pts',(-39.7940671596448,36.2091079829044,37.2172791023278));
#25404=CARTESIAN_POINT('Ctrl Pts',(-39.8321220884911,36.2243729022961,37.2633283236939));
#25405=CARTESIAN_POINT('Ctrl Pts',(-39.8699674737866,36.2407423268217,37.3091845746951));
#25406=CARTESIAN_POINT('Ctrl Pts',(-39.9075774228251,36.258205057003,37.354816481842));
#25407=CARTESIAN_POINT('Ctrl Pts',(-39.9451873718635,36.2756677871843,37.400448388989));
#25408=CARTESIAN_POINT('Ctrl Pts',(-39.9825618823067,36.2942238219334,37.4458559494362));
#25409=CARTESIAN_POINT('Ctrl Pts',(-40.0196753836261,36.3138604657633,37.4910080966812));
#25410=CARTESIAN_POINT('Ctrl Pts',(-40.0567888849456,36.3334971095933,37.5361602439262));
#25411=CARTESIAN_POINT('Ctrl Pts',(-40.0936413748243,36.3542143612781,37.5810569751502));
#25412=CARTESIAN_POINT('Ctrl Pts',(-40.1302076398849,36.3759980466904,37.6256675733451));
#25413=CARTESIAN_POINT('Ctrl Pts',(-40.1667739049455,36.3977817321028,37.6702781715401));
#25414=CARTESIAN_POINT('Ctrl Pts',(-40.2030539428982,36.42063184988,37.7146026339187));
#25415=CARTESIAN_POINT('Ctrl Pts',(-40.2390229320341,36.4445327666565,37.7586106350066));
#25416=CARTESIAN_POINT('Ctrl Pts',(-40.27499192117,36.468433683433,37.8026186360944));
#25417=CARTESIAN_POINT('Ctrl Pts',(-40.3106498592423,36.4933853977163,37.8463101731435));
#25418=CARTESIAN_POINT('Ctrl Pts',(-40.3459723501384,36.5193708382809,37.8896553537003));
#25419=CARTESIAN_POINT('Ctrl Pts',(-40.3812948410344,36.5453562788454,37.933000534257));
#25420=CARTESIAN_POINT('Ctrl Pts',(-40.4162818825551,36.5723754440713,37.9759993556171));
#25421=CARTESIAN_POINT('Ctrl Pts',(-40.4509095376073,36.6004098482494,38.0186223992661));
#25422=CARTESIAN_POINT('Ctrl Pts',(-40.4855371926595,36.6284442524275,38.0612454429149));
#25423=CARTESIAN_POINT('Ctrl Pts',(-40.5198054590814,36.6574938938075,38.1034927061915));
#25424=CARTESIAN_POINT('Ctrl Pts',(-40.5536908915443,36.687538897489,38.145335284775));
#25425=CARTESIAN_POINT('Ctrl Pts',(-40.5875763240073,36.7175839011704,38.1871778633585));
#25426=CARTESIAN_POINT('Ctrl Pts',(-40.6210789203957,36.7486242652774,38.2286157546364));
#25427=CARTESIAN_POINT('Ctrl Pts',(-40.6541757592299,36.7806387529162,38.2696206080363));
#25428=CARTESIAN_POINT('Ctrl Pts',(-40.687272598064,36.8126532405551,38.3106254614361));
#25429=CARTESIAN_POINT('Ctrl Pts',(-40.7199636772774,36.845641849727,38.3511972743978));
#25430=CARTESIAN_POINT('Ctrl Pts',(-40.7522266306062,36.8795820106068,38.3913082888937));
#25431=CARTESIAN_POINT('Ctrl Pts',(-40.7844895839349,36.9135221714866,38.4314193033897));
#25432=CARTESIAN_POINT('Ctrl Pts',(-40.8163244093647,36.9484138819554,38.4710695169156));
#25433=CARTESIAN_POINT('Ctrl Pts',(-40.8477093264549,36.9842332701427,38.5102318019748));
#25434=CARTESIAN_POINT('Ctrl Pts',(-40.8790942435451,37.0200526583299,38.5493940870341));
#25435=CARTESIAN_POINT('Ctrl Pts',(-40.9100292503363,37.0567997219994,38.5880684411817));
#25436=CARTESIAN_POINT('Ctrl Pts',(-40.9404931820171,37.0944493199032,38.6262284045748));
#25437=CARTESIAN_POINT('Ctrl Pts',(-40.9709571136978,37.132098917807,38.664388367968));
#25438=CARTESIAN_POINT('Ctrl Pts',(-41.0009499683659,37.1706510475943,38.7020339382242));
#25439=CARTESIAN_POINT('Ctrl Pts',(-41.030451225803,37.2100793330453,38.7391393593644));
#25440=CARTESIAN_POINT('Ctrl Pts',(-39.2238625385841,36.0678153114539,36.6208944666028));
#25441=CARTESIAN_POINT('Ctrl Pts',(-39.2646282965863,36.073142007383,36.6695847129169));
#25442=CARTESIAN_POINT('Ctrl Pts',(-39.3052981762699,36.0796807626077,36.7182217297142));
#25443=CARTESIAN_POINT('Ctrl Pts',(-39.34584255874,36.0874267642663,36.7667700899032));
#25444=CARTESIAN_POINT('Ctrl Pts',(-39.3863509396808,36.0951658878348,36.8152753414023));
#25445=CARTESIAN_POINT('Ctrl Pts',(-39.4267340433523,36.104110114281,36.8636920902664));
#25446=CARTESIAN_POINT('Ctrl Pts',(-39.4669625126864,36.1142528943672,36.911985133444));
#25447=CARTESIAN_POINT('Ctrl Pts',(-39.5071909820206,36.1243956744533,36.9602781766217));
#25448=CARTESIAN_POINT('Ctrl Pts',(-39.5472648141921,36.1357370074583,37.0084475107197));
#25449=CARTESIAN_POINT('Ctrl Pts',(-39.5871548776739,36.148268604512,37.0564581134567));
#25450=CARTESIAN_POINT('Ctrl Pts',(-39.6270449411558,36.1608002015658,37.1044687161937));
#25451=CARTESIAN_POINT('Ctrl Pts',(-39.6667512331317,36.1745220617773,37.1523205841918));
#25452=CARTESIAN_POINT('Ctrl Pts',(-39.7062448898175,36.1894241687108,37.1999789266909));
#25453=CARTESIAN_POINT('Ctrl Pts',(-39.7457385465032,36.2043262756443,37.24763726919));
#25454=CARTESIAN_POINT('Ctrl Pts',(-39.7850195651239,36.220408628246,37.2951020828413));
#25455=CARTESIAN_POINT('Ctrl Pts',(-39.8240593914136,36.2376594970707,37.3423388588098));
#25456=CARTESIAN_POINT('Ctrl Pts',(-39.8630992177033,36.2549103658954,37.3895756347783));
#25457=CARTESIAN_POINT('Ctrl Pts',(-39.9018978489292,36.2733297497268,37.4365843697479));
#25458=CARTESIAN_POINT('Ctrl Pts',(-39.9404270817729,36.2929042231687,37.4833308868348));
#25459=CARTESIAN_POINT('Ctrl Pts',(-39.9789563146166,36.3124786966106,37.5300774039217));
#25460=CARTESIAN_POINT('Ctrl Pts',(-40.017216146372,36.3332082582817,37.5765616998417));
#25461=CARTESIAN_POINT('Ctrl Pts',(-40.0551787655156,36.3550778063297,37.6227499791836));
#25462=CARTESIAN_POINT('Ctrl Pts',(-40.0931413846591,36.3769473543777,37.6689382585255));
#25463=CARTESIAN_POINT('Ctrl Pts',(-40.130806788518,36.3999568872584,37.7148305180427));
#25464=CARTESIAN_POINT('Ctrl Pts',(-40.1681475976734,36.4240896485919,37.7603933927753));
#25465=CARTESIAN_POINT('Ctrl Pts',(-40.2054884068288,36.4482224099254,37.8059562675079));
#25466=CARTESIAN_POINT('Ctrl Pts',(-40.2425046186569,36.4734783980113,37.8511897542544));
#25467=CARTESIAN_POINT('Ctrl Pts',(-40.2791693254774,36.4998392262471,37.8960609668463));
#25468=CARTESIAN_POINT('Ctrl Pts',(-40.3158340322977,36.526200054483,37.9409321794382));
#25469=CARTESIAN_POINT('Ctrl Pts',(-40.352147231541,36.5536657210148,37.9854411147245));
#25470=CARTESIAN_POINT('Ctrl Pts',(-40.3880825262885,36.5822162357075,38.0295554129948));
#25471=CARTESIAN_POINT('Ctrl Pts',(-40.4240178210361,36.6107667504003,38.073669711265));
#25472=CARTESIAN_POINT('Ctrl Pts',(-40.4595752087639,36.6404021112443,38.1173893694198));
#25473=CARTESIAN_POINT('Ctrl Pts',(-40.4947288415519,36.6711007535647,38.160682601098));
#25474=CARTESIAN_POINT('Ctrl Pts',(-40.5298824743399,36.7017993958849,38.2039758327763));
#25475=CARTESIAN_POINT('Ctrl Pts',(-40.5646323497188,36.7335613175213,38.2468426349361));
#25476=CARTESIAN_POINT('Ctrl Pts',(-40.5989532062203,36.7663634105331,38.2892518406301));
#25477=CARTESIAN_POINT('Ctrl Pts',(-40.6332740627219,36.799165503545,38.331661046324));
#25478=CARTESIAN_POINT('Ctrl Pts',(-40.6671658979351,36.833007765625,38.3736126525723));
#25479=CARTESIAN_POINT('Ctrl Pts',(-40.7006040734473,36.8678655790743,38.4150761570084));
#25480=CARTESIAN_POINT('Ctrl Pts',(-40.7340422489594,36.9027233925236,38.4565396614444));
#25481=CARTESIAN_POINT('Ctrl Pts',(-40.7670267624215,36.938596754891,38.4975150611547));
#25482=CARTESIAN_POINT('Ctrl Pts',(-40.7995336341785,36.9754595744115,38.5379725625591));
#25483=CARTESIAN_POINT('Ctrl Pts',(-40.8320405059355,37.0123223939319,38.5784300639635));
#25484=CARTESIAN_POINT('Ctrl Pts',(-40.8640697337037,37.0501746680138,38.618369664219));
#25485=CARTESIAN_POINT('Ctrl Pts',(-40.8955980313347,37.0889888686504,38.6577623217111));
#25486=CARTESIAN_POINT('Ctrl Pts',(-40.9271263289655,37.1278030692871,38.6971549792031));
#25487=CARTESIAN_POINT('Ctrl Pts',(-40.9581536942437,37.1675791937501,38.7360006911634));
#25488=CARTESIAN_POINT('Ctrl Pts',(-40.9886575682726,37.2082883176943,38.7742712100345));
#25489=CARTESIAN_POINT('Ctrl Pts',(-39.1213009037391,36.0593349777119,36.5872926664368));
#25490=CARTESIAN_POINT('Ctrl Pts',(-39.1634150972342,36.0636128402979,36.6374640999373));
#25491=CARTESIAN_POINT('Ctrl Pts',(-39.2054433505444,36.0691789179925,36.6875969316031));
#25492=CARTESIAN_POINT('Ctrl Pts',(-39.2473531680651,36.0760288520249,36.7376523940249));
#25493=CARTESIAN_POINT('Ctrl Pts',(-39.2892257716136,36.0828727036338,36.7876634095199));
#25494=CARTESIAN_POINT('Ctrl Pts',(-39.3309801462962,36.0909981320292,36.8375971891504));
#25495=CARTESIAN_POINT('Ctrl Pts',(-39.3725840666773,36.100398815097,36.8874151893489));
#25496=CARTESIAN_POINT('Ctrl Pts',(-39.4141879870585,36.1097994981648,36.9372331895473));
#25497=CARTESIAN_POINT('Ctrl Pts',(-39.4556414498437,36.1204754351501,36.9869354063684));
#25498=CARTESIAN_POINT('Ctrl Pts',(-39.4969124627552,36.1324183387962,37.0364834761731));
#25499=CARTESIAN_POINT('Ctrl Pts',(-39.5381834756667,36.1443612424423,37.0860315459778));
#25500=CARTESIAN_POINT('Ctrl Pts',(-39.5792720354387,36.1575711117933,37.1354254648433));
#25501=CARTESIAN_POINT('Ctrl Pts',(-39.6201464322449,36.1720377072933,37.1846271081025));
#25502=CARTESIAN_POINT('Ctrl Pts',(-39.6610208290511,36.1865043027934,37.2338287513618));
#25503=CARTESIAN_POINT('Ctrl Pts',(-39.7016810596549,36.2022276232881,37.2828381151187));
#25504=CARTESIAN_POINT('Ctrl Pts',(-39.7420957453741,36.219195492734,37.3316173723016));
#25505=CARTESIAN_POINT('Ctrl Pts',(-39.7825104310933,36.2361633621799,37.3803966294844));
#25506=CARTESIAN_POINT('Ctrl Pts',(-39.822679568738,36.2543757792275,37.4289457762338));
#25507=CARTESIAN_POINT('Ctrl Pts',(-39.8625721590876,36.2738186501582,37.4772273412781));
#25508=CARTESIAN_POINT('Ctrl Pts',(-39.9024647494372,36.2932615210888,37.5255089063225));
#25509=CARTESIAN_POINT('Ctrl Pts',(-39.942080789334,36.3139348443555,37.5735228858394));
#25510=CARTESIAN_POINT('Ctrl Pts',(-39.9813897066777,36.335822630304,37.6212322219917));
#25511=CARTESIAN_POINT('Ctrl Pts',(-40.0206986240214,36.3577104162525,37.668941558144));
#25512=CARTESIAN_POINT('Ctrl Pts',(-40.0597004156941,36.3808126631406,37.7163462471529));
#25513=CARTESIAN_POINT('Ctrl Pts',(-40.0983649837487,36.4051115100372,37.763409701623));
#25514=CARTESIAN_POINT('Ctrl Pts',(-40.1370295518033,36.4294103569339,37.8104731560931));
#25515=CARTESIAN_POINT('Ctrl Pts',(-40.1753568931785,36.4549058019088,37.8571953722981));
#25516=CARTESIAN_POINT('Ctrl Pts',(-40.2133174303323,36.481578140267,37.9035402895529));
#25517=CARTESIAN_POINT('Ctrl Pts',(-40.2512779674861,36.5082504786252,37.9498852068076));
#25518=CARTESIAN_POINT('Ctrl Pts',(-40.2888716974199,36.5360997082516,37.9958528214448));
#25519=CARTESIAN_POINT('Ctrl Pts',(-40.3260696085235,36.5651043110576,38.0414076549687));
#25520=CARTESIAN_POINT('Ctrl Pts',(-40.3632675196271,36.5941089138638,38.0869624884926));
#25521=CARTESIAN_POINT('Ctrl Pts',(-40.4000696089563,36.6242688875483,38.1321045372966));
#25522=CARTESIAN_POINT('Ctrl Pts',(-40.4364474754407,36.6555609337657,38.1767989596455));
#25523=CARTESIAN_POINT('Ctrl Pts',(-40.4728253419251,36.686852979983,38.2214933819945));
#25524=CARTESIAN_POINT('Ctrl Pts',(-40.5087789826821,36.7192770962499,38.2657401743488));
#25525=CARTESIAN_POINT('Ctrl Pts',(-40.5442806508694,36.7528082398403,38.3095051853305));
#25526=CARTESIAN_POINT('Ctrl Pts',(-40.5797823190567,36.7863393834308,38.3532701963122));
#25527=CARTESIAN_POINT('Ctrl Pts',(-40.6148320118633,36.8209775516863,38.3965534224558));
#25528=CARTESIAN_POINT('Ctrl Pts',(-40.6494026793325,36.8566959960423,38.4393214552702));
#25529=CARTESIAN_POINT('Ctrl Pts',(-40.6839733468017,36.8924144403984,38.4820894880846));
#25530=CARTESIAN_POINT('Ctrl Pts',(-40.7180649861996,36.9292131580259,38.5243423241839));
#25531=CARTESIAN_POINT('Ctrl Pts',(-40.7516512860782,36.9670637357012,38.5660473493613));
#25532=CARTESIAN_POINT('Ctrl Pts',(-40.7852375859569,37.0049143133765,38.6077523745386));
#25533=CARTESIAN_POINT('Ctrl Pts',(-40.8183185436573,37.0438167481007,38.6489095854915));
#25534=CARTESIAN_POINT('Ctrl Pts',(-40.850868626706,37.0837410057141,38.6894872124688));
#25535=CARTESIAN_POINT('Ctrl Pts',(-40.8834187097547,37.1236652633276,38.7300648394461));
#25536=CARTESIAN_POINT('Ctrl Pts',(-40.9154379155743,37.1646113406675,38.7700628792342));
#25537=CARTESIAN_POINT('Ctrl Pts',(-40.9469015299415,37.2065476288528,38.8094504554143));
#25538=CARTESIAN_POINT('Ctrl Pts',(-39.0207460949714,36.0533905312094,36.5559457683958));
#25539=CARTESIAN_POINT('Ctrl Pts',(-39.0641468291962,36.0565585379072,36.6075281860324));
#25540=CARTESIAN_POINT('Ctrl Pts',(-39.1074736387074,36.0610908816947,36.6590890062573));
#25541=CARTESIAN_POINT('Ctrl Pts',(-39.1506910132618,36.0669838469081,36.7105859702823));
#25542=CARTESIAN_POINT('Ctrl Pts',(-39.1938700127939,36.0728715794419,36.762037207394));
#25543=CARTESIAN_POINT('Ctrl Pts',(-39.2369397677751,36.0801175176109,36.8134246970649));
#25544=CARTESIAN_POINT('Ctrl Pts',(-39.2798650412689,36.0887157332477,36.864706397297));
#25545=CARTESIAN_POINT('Ctrl Pts',(-39.3227903147626,36.0973139488844,36.9159880975291));
#25546=CARTESIAN_POINT('Ctrl Pts',(-39.3655711029354,36.1072644412216,36.9671640037434));
#25547=CARTESIAN_POINT('Ctrl Pts',(-39.4081724052227,36.1185590693907,37.0181922470333));
#25548=CARTESIAN_POINT('Ctrl Pts',(-39.45077370751,36.1298536975599,37.0692204903233));
#25549=CARTESIAN_POINT('Ctrl Pts',(-39.4931955201093,36.1424924605521,37.1201010661334));
#25550=CARTESIAN_POINT('Ctrl Pts',(-39.5354031361866,36.1564650181319,37.1707923471893));
#25551=CARTESIAN_POINT('Ctrl Pts',(-39.5776107522639,36.1704375757116,37.2214836282453));
#25552=CARTESIAN_POINT('Ctrl Pts',(-39.6196041680497,36.1857439266316,37.2719856100209));
#25553=CARTESIAN_POINT('Ctrl Pts',(-39.6613490271611,36.2023715481965,37.3222569749733));
#25554=CARTESIAN_POINT('Ctrl Pts',(-39.7030938862725,36.2189991697614,37.3725283399257));
#25555=CARTESIAN_POINT('Ctrl Pts',(-39.7445901849912,36.2369480604885,37.422569083569));
#25556=CARTESIAN_POINT('Ctrl Pts',(-39.7858039736614,36.256203535727,37.4723382657212));
#25557=CARTESIAN_POINT('Ctrl Pts',(-39.8270177623316,36.2754590109655,37.5221074478735));
#25558=CARTESIAN_POINT('Ctrl Pts',(-39.8679490372736,36.296021068996,37.5716050640911));
#25559=CARTESIAN_POINT('Ctrl Pts',(-39.9085643110985,36.3178728872391,37.6207906185448));
#25560=CARTESIAN_POINT('Ctrl Pts',(-39.9491795849234,36.3397247054822,37.6699761729984));
#25561=CARTESIAN_POINT('Ctrl Pts',(-39.9894788539988,36.3628662819846,37.718849661295));
#25562=CARTESIAN_POINT('Ctrl Pts',(-40.0294291480157,36.3872786837715,37.7673710982308));
#25563=CARTESIAN_POINT('Ctrl Pts',(-40.0693794420325,36.4116910855584,37.8158925351664));
#25564=CARTESIAN_POINT('Ctrl Pts',(-40.108980757423,36.4373743104501,37.8640619164087));
#25565=CARTESIAN_POINT('Ctrl Pts',(-40.1482006948761,36.4643073460468,37.9118398328035));
#25566=CARTESIAN_POINT('Ctrl Pts',(-40.1874206323292,36.4912403816436,37.9596177491984));
#25567=CARTESIAN_POINT('Ctrl Pts',(-40.226259188349,36.5194232255428,38.0070041964814));
#25568=CARTESIAN_POINT('Ctrl Pts',(-40.2646845876771,36.5488328203184,38.0539604060487));
#25569=CARTESIAN_POINT('Ctrl Pts',(-40.3031099870053,36.5782424150938,38.100916615616));
#25570=CARTESIAN_POINT('Ctrl Pts',(-40.3411222262111,36.6088787581198,38.147442583275));
#25571=CARTESIAN_POINT('Ctrl Pts',(-40.3786902060768,36.6407167846715,38.1935002444121));
#25572=CARTESIAN_POINT('Ctrl Pts',(-40.4162581859424,36.6725548112233,38.2395579055492));
#25573=CARTESIAN_POINT('Ctrl Pts',(-40.4533819031105,36.7055945184568,38.2851472560515));
#25574=CARTESIAN_POINT('Ctrl Pts',(-40.4900309853024,36.7398088753693,38.3302309975876));
#25575=CARTESIAN_POINT('Ctrl Pts',(-40.5266800674943,36.7740232322819,38.3753147391237));
#25576=CARTESIAN_POINT('Ctrl Pts',(-40.5628545114368,36.8094122358185,38.4198928676681));
#25577=CARTESIAN_POINT('Ctrl Pts',(-40.5985247214753,36.8459469329247,38.4639289122053));
#25578=CARTESIAN_POINT('Ctrl Pts',(-40.6341949315138,36.8824816300309,38.5079649567424));
#25579=CARTESIAN_POINT('Ctrl Pts',(-40.6693609044662,36.9201620174461,38.5514589133412));
#25580=CARTESIAN_POINT('Ctrl Pts',(-40.7039938697502,36.9589572674526,38.594375197988));
#25581=CARTESIAN_POINT('Ctrl Pts',(-40.7386268350342,36.9977525174592,38.6372914826347));
#25582=CARTESIAN_POINT('Ctrl Pts',(-40.7727267895576,37.0376626265932,38.6796300914979));
#25583=CARTESIAN_POINT('Ctrl Pts',(-40.8062658348873,37.0786549429194,38.7213563857966));
#25584=CARTESIAN_POINT('Ctrl Pts',(-40.839804880217,37.1196472592456,38.7630826800952));
#25585=CARTESIAN_POINT('Ctrl Pts',(-40.8727830133582,37.1617217791039,38.8041966561039));
#25586=CARTESIAN_POINT('Ctrl Pts',(-40.9051732536821,37.2048440797748,38.8446646769594));
#25587=CARTESIAN_POINT('Ctrl Pts',(-38.9201912862036,36.0474460847069,36.5245988703548));
#25588=CARTESIAN_POINT('Ctrl Pts',(-38.9648785611582,36.0495042355166,36.5775922721275));
#25589=CARTESIAN_POINT('Ctrl Pts',(-39.0095039268703,36.053002845397,36.6305810809114));
#25590=CARTESIAN_POINT('Ctrl Pts',(-39.0540288584583,36.0579388417914,36.6835195465397));
#25591=CARTESIAN_POINT('Ctrl Pts',(-39.0985142539742,36.0628704552501,36.7364110052682));
#25592=CARTESIAN_POINT('Ctrl Pts',(-39.142899389254,36.0692369031925,36.7892522049794));
#25593=CARTESIAN_POINT('Ctrl Pts',(-39.1871460158604,36.0770326513983,36.8419976052451));
#25594=CARTESIAN_POINT('Ctrl Pts',(-39.2313926424668,36.084828399604,36.8947430055108));
#25595=CARTESIAN_POINT('Ctrl Pts',(-39.2755007560271,36.0940534472931,36.9473926011183));
#25596=CARTESIAN_POINT('Ctrl Pts',(-39.3194323476903,36.1046997999852,36.9999010178936));
#25597=CARTESIAN_POINT('Ctrl Pts',(-39.3633639393533,36.1153461526773,37.0524094346688));
#25598=CARTESIAN_POINT('Ctrl Pts',(-39.4071190047799,36.1274138093109,37.1047766674234));
#25599=CARTESIAN_POINT('Ctrl Pts',(-39.4506598401283,36.1408923289704,37.1569575862761));
#25600=CARTESIAN_POINT('Ctrl Pts',(-39.4942006754768,36.1543708486299,37.2091385051288));
#25601=CARTESIAN_POINT('Ctrl Pts',(-39.5375272764445,36.1692602299752,37.2611331049231));
#25602=CARTESIAN_POINT('Ctrl Pts',(-39.5806023089482,36.185547603659,37.3128965776451));
#25603=CARTESIAN_POINT('Ctrl Pts',(-39.6236773414518,36.2018349773427,37.3646600503671));
#25604=CARTESIAN_POINT('Ctrl Pts',(-39.6665008012444,36.2195203417495,37.4161923909043));
#25605=CARTESIAN_POINT('Ctrl Pts',(-39.7090357882352,36.2385884212958,37.4674491901644));
#25606=CARTESIAN_POINT('Ctrl Pts',(-39.7515707752261,36.2576565008421,37.5187059894245));
#25607=CARTESIAN_POINT('Ctrl Pts',(-39.7938172852132,36.2781072936366,37.5696872423429));
#25608=CARTESIAN_POINT('Ctrl Pts',(-39.8357389155194,36.2999231441743,37.6203490150978));
#25609=CARTESIAN_POINT('Ctrl Pts',(-39.8776605458256,36.3217389947119,37.6710107878528));
#25610=CARTESIAN_POINT('Ctrl Pts',(-39.9192572923035,36.3449199008286,37.7213530754372));
#25611=CARTESIAN_POINT('Ctrl Pts',(-39.9604933122826,36.3694458575057,37.7713324948385));
#25612=CARTESIAN_POINT('Ctrl Pts',(-40.0017293322618,36.3939718141829,37.8213119142398));
#25613=CARTESIAN_POINT('Ctrl Pts',(-40.0426046216675,36.4198428189912,37.8709284605194));
#25614=CARTESIAN_POINT('Ctrl Pts',(-40.0830839594199,36.4470365518267,37.9201393760542));
#25615=CARTESIAN_POINT('Ctrl Pts',(-40.1235632971723,36.474230284662,37.969350291589));
#25616=CARTESIAN_POINT('Ctrl Pts',(-40.163646679278,36.5027467428342,38.018155571518));
#25617=CARTESIAN_POINT('Ctrl Pts',(-40.2032995668307,36.5325613295791,38.0665131571287));
#25618=CARTESIAN_POINT('Ctrl Pts',(-40.2429524543834,36.562375916324,38.1148707427393));
#25619=CARTESIAN_POINT('Ctrl Pts',(-40.2821748434659,36.5934886286912,38.1627806292535));
#25620=CARTESIAN_POINT('Ctrl Pts',(-40.3209329367128,36.6258726355774,38.2102015291787));
#25621=CARTESIAN_POINT('Ctrl Pts',(-40.3596910299596,36.6582566424635,38.257622429104));
#25622=CARTESIAN_POINT('Ctrl Pts',(-40.3979848235389,36.6919119406636,38.3045543377541));
#25623=CARTESIAN_POINT('Ctrl Pts',(-40.4357813197353,36.7268095108983,38.3509568098446));
#25624=CARTESIAN_POINT('Ctrl Pts',(-40.4735778159318,36.7617070811331,38.397359281935));
#25625=CARTESIAN_POINT('Ctrl Pts',(-40.5108770110103,36.7978469199508,38.4432323128804));
#25626=CARTESIAN_POINT('Ctrl Pts',(-40.5476467636181,36.8351978698072,38.4885363691403));
#25627=CARTESIAN_POINT('Ctrl Pts',(-40.584416516226,36.8725488196634,38.5338404254003));
#25628=CARTESIAN_POINT('Ctrl Pts',(-40.6206568227329,36.9111108768664,38.5785755024985));
#25629=CARTESIAN_POINT('Ctrl Pts',(-40.6563364534222,36.9508507992041,38.6227030466147));
#25630=CARTESIAN_POINT('Ctrl Pts',(-40.6920160841115,36.9905907215418,38.6668305907309));
#25631=CARTESIAN_POINT('Ctrl Pts',(-40.727135035458,37.0315085050857,38.7103505975043));
#25632=CARTESIAN_POINT('Ctrl Pts',(-40.7616630430686,37.0735688801247,38.7532255591243));
#25633=CARTESIAN_POINT('Ctrl Pts',(-40.7961910506793,37.1156292551636,38.7961005207444));
#25634=CARTESIAN_POINT('Ctrl Pts',(-40.8301281111422,37.1588322175403,38.8383304329737));
#25635=CARTESIAN_POINT('Ctrl Pts',(-40.8634449774227,37.2031405306967,38.8798788985044));
#25636=CARTESIAN_POINT('Ctrl Pts',(-38.8216486787866,36.0440450754439,36.4955134247666));
#25637=CARTESIAN_POINT('Ctrl Pts',(-38.8675604854068,36.0449321771633,36.5498474686122));
#25638=CARTESIAN_POINT('Ctrl Pts',(-38.9134244761254,36.047335827461,36.6041963012607));
#25639=CARTESIAN_POINT('Ctrl Pts',(-38.9591989734608,36.0512537858363,36.6585105300504));
#25640=CARTESIAN_POINT('Ctrl Pts',(-39.0049328251677,36.0551682652464,36.7127765303266));
#25641=CARTESIAN_POINT('Ctrl Pts',(-39.0505773373462,36.0605943642153,36.7670079822283));
#25642=CARTESIAN_POINT('Ctrl Pts',(-39.0960911068884,36.0675271092293,36.8211556889297));
#25643=CARTESIAN_POINT('Ctrl Pts',(-39.1416048764306,36.0744598542433,36.8753033956312));
#25644=CARTESIAN_POINT('Ctrl Pts',(-39.1869878983544,36.0828992445309,36.929367351204));
#25645=CARTESIAN_POINT('Ctrl Pts',(-39.2321990079216,36.0928375767059,36.9832985122337));
#25646=CARTESIAN_POINT('Ctrl Pts',(-39.2774101174888,36.1027759088809,37.0372296732634));
#25647=CARTESIAN_POINT('Ctrl Pts',(-39.3224493097507,36.1142131818435,37.0910280338458));
#25648=CARTESIAN_POINT('Ctrl Pts',(-39.3672757328278,36.127138976372,37.1446447927315));
#25649=CARTESIAN_POINT('Ctrl Pts',(-39.412102155905,36.1400647709004,37.1982615516173));
#25650=CARTESIAN_POINT('Ctrl Pts',(-39.456715804891,36.1544790855687,37.2516967029369));
#25651=CARTESIAN_POINT('Ctrl Pts',(-39.5010762146839,36.170368804263,37.3049017759191));
#25652=CARTESIAN_POINT('Ctrl Pts',(-39.5454366244767,36.1862585229573,37.3581068489013));
#25653=CARTESIAN_POINT('Ctrl Pts',(-39.5895437902214,36.2036236439281,37.411081837722));
#25654=CARTESIAN_POINT('Ctrl Pts',(-39.6333577068124,36.2224483779869,37.463778689801));
#25655=CARTESIAN_POINT('Ctrl Pts',(-39.6771716234035,36.2412731120458,37.51647554188));
#25656=CARTESIAN_POINT('Ctrl Pts',(-39.7206922860459,36.2615574571228,37.568894251449));
#25657=CARTESIAN_POINT('Ctrl Pts',(-39.763880222015,36.2832829796017,37.6209872710733));
#25658=CARTESIAN_POINT('Ctrl Pts',(-39.8070681579841,36.3050085020806,37.6730802906977));
#25659=CARTESIAN_POINT('Ctrl Pts',(-39.8499233625534,36.3281751995749,37.7248476146753));
#25660=CARTESIAN_POINT('Ctrl Pts',(-39.8924069668004,36.3527620274664,37.7762422867567));
#25661=CARTESIAN_POINT('Ctrl Pts',(-39.9348905710474,36.3773488553579,37.8276369588381));
#25662=CARTESIAN_POINT('Ctrl Pts',(-39.9770025703228,36.4033558109476,37.8786589733977));
#25663=CARTESIAN_POINT('Ctrl Pts',(-40.0187047698331,36.4307592767579,37.9292620503397));
#25664=CARTESIAN_POINT('Ctrl Pts',(-40.0604069693434,36.4581627425682,37.9798651272818));
#25665=CARTESIAN_POINT('Ctrl Pts',(-40.1016993645249,36.4869627155928,38.0300492610674));
#25666=CARTESIAN_POINT('Ctrl Pts',(-40.1425445038216,36.5171330482867,38.0797689315001));
#25667=CARTESIAN_POINT('Ctrl Pts',(-40.1833896431183,36.5473033809806,38.1294886019328));
#25668=CARTESIAN_POINT('Ctrl Pts',(-40.2237875220601,36.5788440700355,38.1787438035703));
#25669=CARTESIAN_POINT('Ctrl Pts',(-40.2637015000916,36.6117264852023,38.2274898584855));
#25670=CARTESIAN_POINT('Ctrl Pts',(-40.3036154781231,36.6446089003691,38.2762359134006));
#25671=CARTESIAN_POINT('Ctrl Pts',(-40.3430455508759,36.6788330380435,38.3244728162577));
#25672=CARTESIAN_POINT('Ctrl Pts',(-40.381955955092,36.7143678371214,38.372156812246));
#25673=CARTESIAN_POINT('Ctrl Pts',(-40.420866359308,36.7499026361994,38.4198408082342));
#25674=CARTESIAN_POINT('Ctrl Pts',(-40.4592570907285,36.7867480927872,38.4669718921339));
#25675=CARTESIAN_POINT('Ctrl Pts',(-40.4970933281026,36.8248707711673,38.5135073114282));
#25676=CARTESIAN_POINT('Ctrl Pts',(-40.5349295654766,36.8629934495474,38.5600427307225));
#25677=CARTESIAN_POINT('Ctrl Pts',(-40.5722113046629,36.9023933455436,38.6059824803173));
#25678=CARTESIAN_POINT('Ctrl Pts',(-40.6089047294248,36.9430347093574,38.6512848873549));
#25679=CARTESIAN_POINT('Ctrl Pts',(-40.6455981541867,36.9836760731712,38.6965872943927));
#25680=CARTESIAN_POINT('Ctrl Pts',(-40.6817032605078,37.0255589003514,38.7412523539138));
#25681=CARTESIAN_POINT('Ctrl Pts',(-40.7171872983561,37.068645191732,38.7852395481339));
#25682=CARTESIAN_POINT('Ctrl Pts',(-40.7526713362044,37.1117314831127,38.8292267423539));
#25683=CARTESIAN_POINT('Ctrl Pts',(-40.7875343016955,37.1560212339757,38.872536066457));
#25684=CARTESIAN_POINT('Ctrl Pts',(-40.8217445702653,37.201474264566,38.9151282310574));
#25685=CARTESIAN_POINT('Ctrl Pts',(-38.7247757052312,36.0427370989735,36.4682927109237));
#25686=CARTESIAN_POINT('Ctrl Pts',(-38.7718578692351,36.0424028155446,36.5239060150788));
#25687=CARTESIAN_POINT('Ctrl Pts',(-38.8189082888934,36.043660957969,36.5795557599548));
#25688=CARTESIAN_POINT('Ctrl Pts',(-38.8658820090438,36.0465103227804,36.6351887739484));
#25689=CARTESIAN_POINT('Ctrl Pts',(-38.9128140187114,36.0493571574882,36.6907723884083));
#25690=CARTESIAN_POINT('Ctrl Pts',(-38.9596694593267,36.0537923896288,36.74633929494));
#25691=CARTESIAN_POINT('Ctrl Pts',(-39.0064036414297,36.0598117889971,36.8018364953211));
#25692=CARTESIAN_POINT('Ctrl Pts',(-39.0531378235326,36.0658311883654,36.8573336957021));
#25693=CARTESIAN_POINT('Ctrl Pts',(-39.099750741452,36.0734347542309,36.912761183198));
#25694=CARTESIAN_POINT('Ctrl Pts',(-39.1461979370387,36.0826152345168,36.9680660925603));
#25695=CARTESIAN_POINT('Ctrl Pts',(-39.1926451326255,36.0917957148027,37.0233710019225));
#25696=CARTESIAN_POINT('Ctrl Pts',(-39.2389266002433,36.102553108395,37.0785533264399));
#25697=CARTESIAN_POINT('Ctrl Pts',(-39.2849981978721,36.1148771551806,37.133560434694));
#25698=CARTESIAN_POINT('Ctrl Pts',(-39.3310697955009,36.1272012019662,37.1885675429481));
#25699=CARTESIAN_POINT('Ctrl Pts',(-39.3769315175499,36.1410919004496,37.2433994282638));
#25700=CARTESIAN_POINT('Ctrl Pts',(-39.4225396223406,36.156536002056,37.298003793462));
#25701=CARTESIAN_POINT('Ctrl Pts',(-39.4681477271312,36.1719801036622,37.3526081586602));
#25702=CARTESIAN_POINT('Ctrl Pts',(-39.513502209129,36.1889776065172,37.4069849971147));
#25703=CARTESIAN_POINT('Ctrl Pts',(-39.5585598104479,36.2075122988592,37.4610824456581));
#25704=CARTESIAN_POINT('Ctrl Pts',(-39.6036174117667,36.2260469912013,37.5151798942014));
#25705=CARTESIAN_POINT('Ctrl Pts',(-39.6483781269388,36.2461188707815,37.5689979462689));
#25706=CARTESIAN_POINT('Ctrl Pts',(-39.6927992643964,36.2677087935801,37.6224852716482));
#25707=CARTESIAN_POINT('Ctrl Pts',(-39.737220401854,36.2892987163787,37.6759725970276));
#25708=CARTESIAN_POINT('Ctrl Pts',(-39.7813019562067,36.3124066797758,37.7291291892284));
#25709=CARTESIAN_POINT('Ctrl Pts',(-39.8250018836525,36.3370106440169,37.7819043489209));
#25710=CARTESIAN_POINT('Ctrl Pts',(-39.8687018110983,36.3616146082581,37.8346795086135));
#25711=CARTESIAN_POINT('Ctrl Pts',(-39.9120201063341,36.3877145703575,37.8870732293937));
#25712=CARTESIAN_POINT('Ctrl Pts',(-39.9549154535338,36.4152856368725,37.9390355395383));
#25713=CARTESIAN_POINT('Ctrl Pts',(-39.9978108007334,36.4428567033876,37.9909978496829));
#25714=CARTESIAN_POINT('Ctrl Pts',(-40.0402831946916,36.4718988709725,38.0425287428864));
#25715=CARTESIAN_POINT('Ctrl Pts',(-40.0822921263801,36.5023844399883,38.0935790703672));
#25716=CARTESIAN_POINT('Ctrl Pts',(-40.1243010580686,36.532870009004,38.144629397848));
#25717=CARTESIAN_POINT('Ctrl Pts',(-40.1658465223896,36.5647989757511,38.1951991534113));
#25718=CARTESIAN_POINT('Ctrl Pts',(-40.2068888943955,36.598140887239,38.2452401049829));
#25719=CARTESIAN_POINT('Ctrl Pts',(-40.2479312664015,36.6314827987268,38.2952810565544));
#25720=CARTESIAN_POINT('Ctrl Pts',(-40.2884705411118,36.6662376509092,38.3447931980618));
#25721=CARTESIAN_POINT('Ctrl Pts',(-40.3284680532555,36.7023722955423,38.3937293061547));
#25722=CARTESIAN_POINT('Ctrl Pts',(-40.3684655653993,36.7385069401753,38.4426654142476));
#25723=CARTESIAN_POINT('Ctrl Pts',(-40.4079213101227,36.7760213728738,38.4910254829877));
#25724=CARTESIAN_POINT('Ctrl Pts',(-40.4467976555966,36.8148798133799,38.5387633878407));
#25725=CARTESIAN_POINT('Ctrl Pts',(-40.4856740010705,36.8537382538859,38.5865012926936));
#25726=CARTESIAN_POINT('Ctrl Pts',(-40.5239709425773,36.8939406974841,38.6336170278665));
#25727=CARTESIAN_POINT('Ctrl Pts',(-40.561651953523,36.9354488001637,38.680065655637));
#25728=CARTESIAN_POINT('Ctrl Pts',(-40.5993329644687,36.9769569028435,38.7265142834075));
#25729=CARTESIAN_POINT('Ctrl Pts',(-40.6363980402809,37.0197706595677,38.7722957981391));
#25730=CARTESIAN_POINT('Ctrl Pts',(-40.6728118292859,37.0638492357256,38.817366534653));
#25731=CARTESIAN_POINT('Ctrl Pts',(-40.709225618291,37.1079278118835,38.862437271167));
#25732=CARTESIAN_POINT('Ctrl Pts',(-40.7449881160701,37.1532712021262,38.9067972239939));
#25733=CARTESIAN_POINT('Ctrl Pts',(-40.7800652133139,37.1998361591463,38.9504040838028));
#25734=CARTESIAN_POINT('Ctrl Pts',(-38.6279027316758,36.0414291225031,36.4410719970808));
#25735=CARTESIAN_POINT('Ctrl Pts',(-38.6761552530635,36.0398734539259,36.4979645615455));
#25736=CARTESIAN_POINT('Ctrl Pts',(-38.7243921016613,36.039986088477,36.5549152186491));
#25737=CARTESIAN_POINT('Ctrl Pts',(-38.7725650446267,36.0417668597245,36.6118670178464));
#25738=CARTESIAN_POINT('Ctrl Pts',(-38.8206952122552,36.0435460497299,36.66876824649));
#25739=CARTESIAN_POINT('Ctrl Pts',(-38.8687615813073,36.0469904150423,36.7256706076517));
#25740=CARTESIAN_POINT('Ctrl Pts',(-38.916716175971,36.0520964687649,36.7825173017124));
#25741=CARTESIAN_POINT('Ctrl Pts',(-38.9646707706347,36.0572025224874,36.8393639957731));
#25742=CARTESIAN_POINT('Ctrl Pts',(-39.0125135845495,36.063970263931,36.896155015192));
#25743=CARTESIAN_POINT('Ctrl Pts',(-39.0601968661558,36.0723928923278,36.9528336728868));
#25744=CARTESIAN_POINT('Ctrl Pts',(-39.1078801477621,36.0808155207247,37.0095123305816));
#25745=CARTESIAN_POINT('Ctrl Pts',(-39.1554038907358,36.0908930349464,37.066078619034));
#25746=CARTESIAN_POINT('Ctrl Pts',(-39.2027206629163,36.1026153339892,37.1224760766564));
#25747=CARTESIAN_POINT('Ctrl Pts',(-39.2500374350968,36.114337633032,37.1788735342789));
#25748=CARTESIAN_POINT('Ctrl Pts',(-39.2971472302088,36.1277047153306,37.2351021535907));
#25749=CARTESIAN_POINT('Ctrl Pts',(-39.3440030299973,36.1427031998488,37.2911058110049));
#25750=CARTESIAN_POINT('Ctrl Pts',(-39.3908588297857,36.1577016843671,37.347109468419));
#25751=CARTESIAN_POINT('Ctrl Pts',(-39.4374606280368,36.1743315691062,37.4028881565074));
#25752=CARTESIAN_POINT('Ctrl Pts',(-39.4837619140834,36.1925762197316,37.4583862015151));
#25753=CARTESIAN_POINT('Ctrl Pts',(-39.5300632001299,36.210820870357,37.5138842465228));
#25754=CARTESIAN_POINT('Ctrl Pts',(-39.5760639678317,36.2306802844402,37.5691016410887));
#25755=CARTESIAN_POINT('Ctrl Pts',(-39.6217183067778,36.2521346075585,37.6239832722232));
#25756=CARTESIAN_POINT('Ctrl Pts',(-39.667372645724,36.2735889306768,37.6788649033576));
#25757=CARTESIAN_POINT('Ctrl Pts',(-39.7126805498601,36.2966381599766,37.7334107637814));
#25758=CARTESIAN_POINT('Ctrl Pts',(-39.7575968005046,36.3212592605674,37.7875664110852));
#25759=CARTESIAN_POINT('Ctrl Pts',(-39.8025130511491,36.3458803611583,37.8417220583889));
#25760=CARTESIAN_POINT('Ctrl Pts',(-39.8470376423455,36.3720733297673,37.8954874853898));
#25761=CARTESIAN_POINT('Ctrl Pts',(-39.8911261372345,36.3998119969872,37.948809028737));
#25762=CARTESIAN_POINT('Ctrl Pts',(-39.9352146321234,36.427550664207,38.0021305720841));
#25763=CARTESIAN_POINT('Ctrl Pts',(-39.9788670248583,36.4568350263522,38.0550082247054));
#25764=CARTESIAN_POINT('Ctrl Pts',(-40.0220397489386,36.4876358316899,38.1073892092343));
#25765=CARTESIAN_POINT('Ctrl Pts',(-40.0652124730189,36.5184366370274,38.1597701937633));
#25766=CARTESIAN_POINT('Ctrl Pts',(-40.1079055227192,36.5507538814668,38.2116545032524));
#25767=CARTESIAN_POINT('Ctrl Pts',(-40.1500762886995,36.5845552892756,38.2629903514803));
#25768=CARTESIAN_POINT('Ctrl Pts',(-40.1922470546799,36.6183566970844,38.3143261997082));
#25769=CARTESIAN_POINT('Ctrl Pts',(-40.2338955313476,36.6536422637751,38.3651135798659));
#25770=CARTESIAN_POINT('Ctrl Pts',(-40.2749801514191,36.6903767539631,38.4153018000635));
#25771=CARTESIAN_POINT('Ctrl Pts',(-40.3160647714905,36.7271112441511,38.4654900202611));
#25772=CARTESIAN_POINT('Ctrl Pts',(-40.3565855295169,36.7652946529604,38.5150790738416));
#25773=CARTESIAN_POINT('Ctrl Pts',(-40.3965019830907,36.8048888555924,38.5640194642532));
#25774=CARTESIAN_POINT('Ctrl Pts',(-40.4364184366645,36.8444830582244,38.6129598546648));
#25775=CARTESIAN_POINT('Ctrl Pts',(-40.4757305804917,36.8854880494245,38.6612515754158));
#25776=CARTESIAN_POINT('Ctrl Pts',(-40.5143991776212,36.9278628909701,38.7088464239191));
#25777=CARTESIAN_POINT('Ctrl Pts',(-40.5530677747507,36.9702377325157,38.7564412724223));
#25778=CARTESIAN_POINT('Ctrl Pts',(-40.5910928200539,37.013982418784,38.8033392423644));
#25779=CARTESIAN_POINT('Ctrl Pts',(-40.6284363602157,37.0590532797192,38.8494935211722));
#25780=CARTESIAN_POINT('Ctrl Pts',(-40.6657799003775,37.1041241406544,38.89564779998));
#25781=CARTESIAN_POINT('Ctrl Pts',(-40.7024419304448,37.1505211702767,38.9410583815309));
#25782=CARTESIAN_POINT('Ctrl Pts',(-40.7383858563626,37.1981980537265,38.9856799365482));
#25783=CARTESIAN_POINT('Ctrl Pts',(-38.5327022782564,36.042218146015,36.4157194736928));
#25784=CARTESIAN_POINT('Ctrl Pts',(-38.582070920586,36.0393906665048,36.4738298424583));
#25785=CARTESIAN_POINT('Ctrl Pts',(-38.6314419402381,36.0383071559065,36.5320222263094));
#25786=CARTESIAN_POINT('Ctrl Pts',(-38.6807637016069,36.0389686897623,36.5902357592848));
#25787=CARTESIAN_POINT('Ctrl Pts',(-38.7300416675413,36.0396296362069,36.6483976013454));
#25788=CARTESIAN_POINT('Ctrl Pts',(-38.7792704554811,36.0420325293332,36.7065805465471));
#25789=CARTESIAN_POINT('Ctrl Pts',(-38.8283986715219,36.0461748081124,36.7647238488323));
#25790=CARTESIAN_POINT('Ctrl Pts',(-38.8775268875627,36.0503170868915,36.8228671511175));
#25791=CARTESIAN_POINT('Ctrl Pts',(-38.9265545245766,36.0561987507077,36.8809708020488));
#25792=CARTESIAN_POINT('Ctrl Pts',(-38.9754304000649,36.0638136102815,36.9389741400892));
#25793=CARTESIAN_POINT('Ctrl Pts',(-39.0243062755532,36.0714284698554,36.9969774781296));
#25794=CARTESIAN_POINT('Ctrl Pts',(-39.0730303824243,36.0807765240684,37.0548804948621));
#25795=CARTESIAN_POINT('Ctrl Pts',(-39.1215518562211,36.0918479683989,37.1126227396887));
#25796=CARTESIAN_POINT('Ctrl Pts',(-39.1700733300179,36.1029194127294,37.1703649845152));
#25797=CARTESIAN_POINT('Ctrl Pts',(-39.2183921637013,36.1157142455581,37.2279464490573));
#25798=CARTESIAN_POINT('Ctrl Pts',(-39.2664579168746,36.1302190676599,37.2853070196423));
#25799=CARTESIAN_POINT('Ctrl Pts',(-39.3145236700479,36.1447238897616,37.3426675902273));
#25800=CARTESIAN_POINT('Ctrl Pts',(-39.3623363357353,36.1609386990197,37.3998072585318));
#25801=CARTESIAN_POINT('Ctrl Pts',(-39.4098460026943,36.1788465295219,37.4566663730815));
#25802=CARTESIAN_POINT('Ctrl Pts',(-39.4573556696534,36.1967543600241,37.5135254876311));
#25803=CARTESIAN_POINT('Ctrl Pts',(-39.5045623309918,36.2163552091614,37.5701040401762));
#25804=CARTESIAN_POINT('Ctrl Pts',(-39.5514167086316,36.2376285797793,37.6263429657525));
#25805=CARTESIAN_POINT('Ctrl Pts',(-39.5982710862714,36.2589019503972,37.6825818913288));
#25806=CARTESIAN_POINT('Ctrl Pts',(-39.6447731734175,36.2818478393999,37.7384811817772));
#25807=CARTESIAN_POINT('Ctrl Pts',(-39.6908744278377,36.3064422611834,37.7939824817302));
#25808=CARTESIAN_POINT('Ctrl Pts',(-39.7369756822578,36.3310366829669,37.8494837816833));
#25809=CARTESIAN_POINT('Ctrl Pts',(-39.7826760972645,36.3572796339542,37.9045870830887));
#25810=CARTESIAN_POINT('Ctrl Pts',(-39.8279279676327,36.3851436901509,37.959234861785));
#25811=CARTESIAN_POINT('Ctrl Pts',(-39.873179838001,36.4130077463476,38.0138826404814));
#25812=CARTESIAN_POINT('Ctrl Pts',(-39.917983157166,36.4424929037033,38.0680748885401));
#25813=CARTESIAN_POINT('Ctrl Pts',(-39.9622911563025,36.4735683570419,38.1217550328776));
#25814=CARTESIAN_POINT('Ctrl Pts',(-40.0065991554391,36.5046438103804,38.1754351772151));
#25815=CARTESIAN_POINT('Ctrl Pts',(-40.0504118281197,36.5373095551866,38.2286032100432));
#25816=CARTESIAN_POINT('Ctrl Pts',(-40.0936834393859,36.5715314693577,38.2812036272513));
#25817=CARTESIAN_POINT('Ctrl Pts',(-40.136955050652,36.6057533835288,38.3338040444593));
#25818=CARTESIAN_POINT('Ctrl Pts',(-40.1796855942259,36.641531462094,38.3858368384154));
#25819=CARTESIAN_POINT('Ctrl Pts',(-40.2218304643064,36.6788283371755,38.4372476896451));
#25820=CARTESIAN_POINT('Ctrl Pts',(-40.263975334387,36.7161252122571,38.4886585408747));
#25821=CARTESIAN_POINT('Ctrl Pts',(-40.3055345248605,36.754940878439,38.5394474419187));
#25822=CARTESIAN_POINT('Ctrl Pts',(-40.346464652041,36.7952347999842,38.589561371138));
#25823=CARTESIAN_POINT('Ctrl Pts',(-40.3873947792216,36.8355287215294,38.6396753003573));
#25824=CARTESIAN_POINT('Ctrl Pts',(-40.4276958371702,36.8773008925874,38.6891142504804));
#25825=CARTESIAN_POINT('Ctrl Pts',(-40.4673257547153,36.9205076940649,38.737826608198));
#25826=CARTESIAN_POINT('Ctrl Pts',(-40.5069556722604,36.9637144955425,38.7865389659155));
#25827=CARTESIAN_POINT('Ctrl Pts',(-40.5459144436521,37.0083559211679,38.8345247241592));
#25828=CARTESIAN_POINT('Ctrl Pts',(-40.5841613979055,37.0543853594171,38.8817337855118));
#25829=CARTESIAN_POINT('Ctrl Pts',(-40.6224083521588,37.1004147976663,38.9289428468643));
#25830=CARTESIAN_POINT('Ctrl Pts',(-40.6599434837245,37.147832241859,38.9753752044751));
#25831=CARTESIAN_POINT('Ctrl Pts',(-40.6967276065595,37.1965881851941,39.0209823812249));
#25832=CARTESIAN_POINT('Ctrl Pts',(-38.4389275238392,36.0447816639384,36.3919506587633));
#25833=CARTESIAN_POINT('Ctrl Pts',(-38.4893637622182,36.0406398859262,36.4512238512357));
#25834=CARTESIAN_POINT('Ctrl Pts',(-38.539822323781,36.0383173783364,36.5106051639133));
#25835=CARTESIAN_POINT('Ctrl Pts',(-38.5902480567288,36.0378166779306,36.5700296922399));
#25836=CARTESIAN_POINT('Ctrl Pts',(-38.6406290139668,36.0373164221236,36.6294014543442));
#25837=CARTESIAN_POINT('Ctrl Pts',(-38.6909771928631,36.0386347396562,36.6888163459556));
#25838=CARTESIAN_POINT('Ctrl Pts',(-38.74123765991,36.0417701921486,36.7482095411327));
#25839=CARTESIAN_POINT('Ctrl Pts',(-38.7914981269569,36.044905644641,36.8076027363098));
#25840=CARTESIAN_POINT('Ctrl Pts',(-38.8416708741728,36.0498582315951,36.8669742256202));
#25841=CARTESIAN_POINT('Ctrl Pts',(-38.8917011594712,36.0566225493811,36.9262592304807));
#25842=CARTESIAN_POINT('Ctrl Pts',(-38.9417314447696,36.063386867167,36.9855442353412));
#25843=CARTESIAN_POINT('Ctrl Pts',(-38.9916192602048,36.0719629147108,37.0447427463364));
#25844=CARTESIAN_POINT('Ctrl Pts',(-39.0413101745598,36.0823413349242,37.1037901736122));
#25845=CARTESIAN_POINT('Ctrl Pts',(-39.0910010889149,36.0927197551375,37.1628376008879));
#25846=CARTESIAN_POINT('Ctrl Pts',(-39.1404950942985,36.1049005463721,37.2217339350668));
#25847=CARTESIAN_POINT('Ctrl Pts',(-39.1897381891798,36.1188704185053,37.2804149159938));
#25848=CARTESIAN_POINT('Ctrl Pts',(-39.2389812840611,36.1328402906386,37.3390958969207));
#25849=CARTESIAN_POINT('Ctrl Pts',(-39.287973460617,36.1485992414516,37.3975615152759));
#25850=CARTESIAN_POINT('Ctrl Pts',(-39.3366612648428,36.1661300767903,37.4557479808452));
#25851=CARTESIAN_POINT('Ctrl Pts',(-39.3853490690688,36.1836609121289,37.5139344464145));
#25852=CARTESIAN_POINT('Ctrl Pts',(-39.4337324932325,36.2029636292092,37.5718417499571));
#25853=CARTESIAN_POINT('Ctrl Pts',(-39.4817587475222,36.224017167372,37.6294067104208));
#25854=CARTESIAN_POINT('Ctrl Pts',(-39.5297850018119,36.2450707055347,37.6869716708845));
#25855=CARTESIAN_POINT('Ctrl Pts',(-39.5774540786024,36.2678750614369,37.7441942791276));
#25856=CARTESIAN_POINT('Ctrl Pts',(-39.6247139674825,36.2924053538775,37.8010121011491));
#25857=CARTESIAN_POINT('Ctrl Pts',(-39.6719738563627,36.3169356463181,37.8578299231705));
#25858=CARTESIAN_POINT('Ctrl Pts',(-39.7188245498275,36.3431918714014,37.914242949947));
#25859=CARTESIAN_POINT('Ctrl Pts',(-39.7652149303884,36.3711453816896,37.9701896307907));
#25860=CARTESIAN_POINT('Ctrl Pts',(-39.8116053109493,36.3990988919778,38.0261363116345));
#25861=CARTESIAN_POINT('Ctrl Pts',(-39.8575353712387,36.4287496830316,38.0816166376605));
#25862=CARTESIAN_POINT('Ctrl Pts',(-39.9029549982392,36.4600654036945,38.1365700758237));
#25863=CARTESIAN_POINT('Ctrl Pts',(-39.9483746252396,36.4913811243574,38.1915235139868));
#25864=CARTESIAN_POINT('Ctrl Pts',(-39.9932838117383,36.5243617696561,38.2459500555599));
#25865=CARTESIAN_POINT('Ctrl Pts',(-40.0376335585701,36.5589713553244,38.299790317254));
#25866=CARTESIAN_POINT('Ctrl Pts',(-40.0819833054019,36.5935809409928,38.353630578948));
#25867=CARTESIAN_POINT('Ctrl Pts',(-40.1257736055232,36.6298194615343,38.4068845522123));
#25868=CARTESIAN_POINT('Ctrl Pts',(-40.1689566805506,36.6676473781038,38.4594941331138));
#25869=CARTESIAN_POINT('Ctrl Pts',(-40.2121397555781,36.7054752946732,38.5121037140154));
#25870=CARTESIAN_POINT('Ctrl Pts',(-40.2547155986539,36.7448926012632,38.5640688941992));
#25871=CARTESIAN_POINT('Ctrl Pts',(-40.2966377564584,36.7858562907448,38.615332975899));
#25872=CARTESIAN_POINT('Ctrl Pts',(-40.3385599142629,36.8268199802263,38.6665970575989));
#25873=CARTESIAN_POINT('Ctrl Pts',(-40.3798283801375,36.8693300460936,38.7171600326734));
#25874=CARTESIAN_POINT('Ctrl Pts',(-40.4203981272041,36.913340106793,38.7669667332631));
#25875=CARTESIAN_POINT('Ctrl Pts',(-40.4609678742707,36.9573501674925,38.8167734338529));
#25876=CARTESIAN_POINT('Ctrl Pts',(-40.5008388960863,37.0028602160348,38.8658238520481));
#25877=CARTESIAN_POINT('Ctrl Pts',(-40.5399676904852,37.0498205976687,38.9140644702981));
#25878=CARTESIAN_POINT('Ctrl Pts',(-40.5790964848841,37.0967809793025,38.9623050885482));
#25879=CARTESIAN_POINT('Ctrl Pts',(-40.6174830456522,37.14519168657,39.0097358991921));
#25880=CARTESIAN_POINT('Ctrl Pts',(-40.6550854902779,37.1949998998915,39.056305151788));
#25881=CARTESIAN_POINT('Ctrl Pts',(-38.3451527694219,36.0473451818618,36.3681818438339));
#25882=CARTESIAN_POINT('Ctrl Pts',(-38.3966566038503,36.0418891053477,36.428617860013));
#25883=CARTESIAN_POINT('Ctrl Pts',(-38.4482027073239,36.0383276007663,36.4891881015171));
#25884=CARTESIAN_POINT('Ctrl Pts',(-38.4997324118508,36.0366646660989,36.5498236251951));
#25885=CARTESIAN_POINT('Ctrl Pts',(-38.5512163603923,36.0350032080402,36.6104053073431));
#25886=CARTESIAN_POINT('Ctrl Pts',(-38.6026839302451,36.0352369499792,36.6710521453642));
#25887=CARTESIAN_POINT('Ctrl Pts',(-38.6540766482982,36.0373655761849,36.7316952334331));
#25888=CARTESIAN_POINT('Ctrl Pts',(-38.7054693663512,36.0394942023905,36.792338321502));
#25889=CARTESIAN_POINT('Ctrl Pts',(-38.7567872237691,36.0435177124826,36.8529776491916));
#25890=CARTESIAN_POINT('Ctrl Pts',(-38.8079719188776,36.0494314884807,36.9135443208722));
#25891=CARTESIAN_POINT('Ctrl Pts',(-38.8591566139861,36.0553452644788,36.9741109925528));
#25892=CARTESIAN_POINT('Ctrl Pts',(-38.9102081379853,36.0631493053533,37.0346049978107));
#25893=CARTESIAN_POINT('Ctrl Pts',(-38.9610684928986,36.0728347014494,37.0949576075357));
#25894=CARTESIAN_POINT('Ctrl Pts',(-39.0119288478118,36.0825200975455,37.1553102172607));
#25895=CARTESIAN_POINT('Ctrl Pts',(-39.0625980248957,36.0940868471861,37.2155214210763));
#25896=CARTESIAN_POINT('Ctrl Pts',(-39.113018461485,36.1075217693508,37.2755228123452));
#25897=CARTESIAN_POINT('Ctrl Pts',(-39.1634388980743,36.1209566915156,37.3355242036141));
#25898=CARTESIAN_POINT('Ctrl Pts',(-39.2136105854986,36.1362597838835,37.3953157720199));
#25899=CARTESIAN_POINT('Ctrl Pts',(-39.2634765269914,36.1534136240587,37.4548295886088));
#25900=CARTESIAN_POINT('Ctrl Pts',(-39.3133424684842,36.1705674642338,37.5143434051978));
#25901=CARTESIAN_POINT('Ctrl Pts',(-39.3629026554732,36.1895720492569,37.5735794597381));
#25902=CARTESIAN_POINT('Ctrl Pts',(-39.4121007864128,36.2104057549646,37.6324704550892));
#25903=CARTESIAN_POINT('Ctrl Pts',(-39.4612989173524,36.2312394606722,37.6913614504403));
#25904=CARTESIAN_POINT('Ctrl Pts',(-39.5101349837871,36.253902283474,37.749907376478));
#25905=CARTESIAN_POINT('Ctrl Pts',(-39.5585535071273,36.2783684465717,37.8080417205678));
#25906=CARTESIAN_POINT('Ctrl Pts',(-39.6069720304676,36.3028346096693,37.8661760646576));
#25907=CARTESIAN_POINT('Ctrl Pts',(-39.6549730023906,36.3291041088485,37.9238988168053));
#25908=CARTESIAN_POINT('Ctrl Pts',(-39.7025018931441,36.3571470732283,37.9811443997964));
#25909=CARTESIAN_POINT('Ctrl Pts',(-39.7500307838977,36.3851900376081,38.0383899827877));
#25910=CARTESIAN_POINT('Ctrl Pts',(-39.7970875853114,36.4150064623599,38.095158386781));
#25911=CARTESIAN_POINT('Ctrl Pts',(-39.8436188401758,36.4465624503471,38.1513851187698));
#25912=CARTESIAN_POINT('Ctrl Pts',(-39.8901500950402,36.4781184383343,38.2076118507586));
#25913=CARTESIAN_POINT('Ctrl Pts',(-39.9361557953568,36.5114139841255,38.2632969010767));
#25914=CARTESIAN_POINT('Ctrl Pts',(-39.9815836777543,36.5464112412911,38.3183770072567));
#25915=CARTESIAN_POINT('Ctrl Pts',(-40.0270115601517,36.5814084984567,38.3734571134366));
#25916=CARTESIAN_POINT('Ctrl Pts',(-40.0718616168206,36.6181074609745,38.4279322660091));
#25917=CARTESIAN_POINT('Ctrl Pts',(-40.1160828967949,36.656466419032,38.4817405765826));
#25918=CARTESIAN_POINT('Ctrl Pts',(-40.1603041767692,36.6948253770893,38.535548887156));
#25919=CARTESIAN_POINT('Ctrl Pts',(-40.2038966724473,36.7348443240874,38.5886903464796));
#25920=CARTESIAN_POINT('Ctrl Pts',(-40.2468108608757,36.7764777815053,38.6411045806601));
#25921=CARTESIAN_POINT('Ctrl Pts',(-40.2897250493041,36.8181112389233,38.6935188148405));
#25922=CARTESIAN_POINT('Ctrl Pts',(-40.3319609231047,36.8613591995997,38.7452058148664));
#25923=CARTESIAN_POINT('Ctrl Pts',(-40.3734704996928,36.9061725195211,38.7961068583283));
#25924=CARTESIAN_POINT('Ctrl Pts',(-40.414980076281,36.9509858394425,38.8470079017903));
#25925=CARTESIAN_POINT('Ctrl Pts',(-40.4557633485205,36.9973645109018,38.8971229799369));
#25926=CARTESIAN_POINT('Ctrl Pts',(-40.495773983065,37.0452558359202,38.9463951550846));
#25927=CARTESIAN_POINT('Ctrl Pts',(-40.5357846176094,37.0931471609388,38.9956673302322));
#25928=CARTESIAN_POINT('Ctrl Pts',(-40.57502260758,37.1425511312811,39.044096593909));
#25929=CARTESIAN_POINT('Ctrl Pts',(-40.6134433739962,37.1934116145889,39.0916279223511));
#25930=CARTESIAN_POINT('Ctrl Pts',(-38.2528053810356,36.051685450517,36.345998711413));
#25931=CARTESIAN_POINT('Ctrl Pts',(-38.3053282503167,36.0448725367672,36.4075425279015));
#25932=CARTESIAN_POINT('Ctrl Pts',(-38.357915230494,36.0400291326329,36.4692488577792));
#25933=CARTESIAN_POINT('Ctrl Pts',(-38.4105040239329,36.0371609165339,36.5310445960988));
#25934=CARTESIAN_POINT('Ctrl Pts',(-38.4630461209646,36.0342952472778,36.5927854626717));
#25935=CARTESIAN_POINT('Ctrl Pts',(-38.5155900182526,36.0334012603794,36.6546155674746));
#25936=CARTESIAN_POINT('Ctrl Pts',(-38.5680735815496,36.0344799595119,36.7164617913297));
#25937=CARTESIAN_POINT('Ctrl Pts',(-38.6205571448467,36.0355586586442,36.7783080151848));
#25938=CARTESIAN_POINT('Ctrl Pts',(-38.6729803643777,36.0386100435895,36.840170346572));
#25939=CARTESIAN_POINT('Ctrl Pts',(-38.7252812502133,36.0436304561532,36.9019756302016));
#25940=CARTESIAN_POINT('Ctrl Pts',(-38.7775821360489,36.0486508687169,36.9637809138313));
#25941=CARTESIAN_POINT('Ctrl Pts',(-38.8297606784486,36.055640307948,37.0255291381914));
#25942=CARTESIAN_POINT('Ctrl Pts',(-38.881755178192,36.0645904625521,37.0871472846484));
#25943=CARTESIAN_POINT('Ctrl Pts',(-38.9337496779355,36.073540617156,37.1487654311053));
#25944=CARTESIAN_POINT('Ctrl Pts',(-38.9855601253396,36.0844514854511,37.2102534881825));
#25945=CARTESIAN_POINT('Ctrl Pts',(-39.0371252575936,36.097310122788,37.2715387463425));
#25946=CARTESIAN_POINT('Ctrl Pts',(-39.0886903898476,36.1101687601249,37.3328240045024));
#25947=CARTESIAN_POINT('Ctrl Pts',(-39.1400101973423,36.1249751640943,37.3939064523297));
#25948=CARTESIAN_POINT('Ctrl Pts',(-39.1910239983568,36.1417117873728,37.4547138610926));
#25949=CARTESIAN_POINT('Ctrl Pts',(-39.2420377993713,36.1584484106512,37.5155212698555));
#25950=CARTESIAN_POINT('Ctrl Pts',(-39.2927455844049,36.1771152501096,37.576053628229));
#25951=CARTESIAN_POINT('Ctrl Pts',(-39.3430873960814,36.197690197282,37.6362393588477));
#25952=CARTESIAN_POINT('Ctrl Pts',(-39.3934292077581,36.2182651444544,37.6964250894664));
#25953=CARTESIAN_POINT('Ctrl Pts',(-39.443405036709,36.240748195499,37.7562641811227));
#25954=CARTESIAN_POINT('Ctrl Pts',(-39.49295579152,36.2651127331137,37.8156858768529));
#25955=CARTESIAN_POINT('Ctrl Pts',(-39.542506546331,36.2894772707283,37.8751075725831));
#25956=CARTESIAN_POINT('Ctrl Pts',(-39.5916322177749,36.3157232903655,37.9341118613208));
#25957=CARTESIAN_POINT('Ctrl Pts',(-39.6402747199215,36.3438197288223,37.9926289735902));
#25958=CARTESIAN_POINT('Ctrl Pts',(-39.688917222068,36.371916167279,38.0511460858596));
#25959=CARTESIAN_POINT('Ctrl Pts',(-39.7370765458555,36.4018630193127,38.1091760107623));
#25960=CARTESIAN_POINT('Ctrl Pts',(-39.7846957480054,36.4336248492489,38.1666501310679));
#25961=CARTESIAN_POINT('Ctrl Pts',(-39.8323149501553,36.4653866791851,38.2241242513735));
#25962=CARTESIAN_POINT('Ctrl Pts',(-39.8793940217993,36.4989634811011,38.2810425563783));
#25963=CARTESIAN_POINT('Ctrl Pts',(-39.9258772967491,36.5343155305869,38.3373377431282));
#25964=CARTESIAN_POINT('Ctrl Pts',(-39.972360571699,36.5696675800726,38.3936329298781));
#25965=CARTESIAN_POINT('Ctrl Pts',(-40.0182480412996,36.606794870538,38.4493049878891));
#25966=CARTESIAN_POINT('Ctrl Pts',(-40.0634854479255,36.6456534827089,38.5042880874195));
#25967=CARTESIAN_POINT('Ctrl Pts',(-40.1087228545514,36.6845120948799,38.5592711869499));
#25968=CARTESIAN_POINT('Ctrl Pts',(-40.1533101897776,36.725102021514,38.6135653177595));
#25969=CARTESIAN_POINT('Ctrl Pts',(-40.1971947326411,36.7673752522233,38.6671062787693));
#25970=CARTESIAN_POINT('Ctrl Pts',(-40.2410792755046,36.8096484829327,38.7206472397791));
#25971=CARTESIAN_POINT('Ctrl Pts',(-40.2842610178336,36.8536050098406,38.7734350210174));
#25972=CARTESIAN_POINT('Ctrl Pts',(-40.3266888998378,36.8991928448641,38.8254072016798));
#25973=CARTESIAN_POINT('Ctrl Pts',(-40.369116781842,36.9447806798878,38.8773793823421));
#25974=CARTESIAN_POINT('Ctrl Pts',(-40.410790795619,36.9919998145336,38.9285359527485));
#25975=CARTESIAN_POINT('Ctrl Pts',(-40.451661663113,37.0407944058147,38.9788164197751));
#25976=CARTESIAN_POINT('Ctrl Pts',(-40.4925325306069,37.0895889970958,39.0290968868015));
#25977=CARTESIAN_POINT('Ctrl Pts',(-40.5326002442068,37.1399590359233,39.078501241083));
#25978=CARTESIAN_POINT('Ctrl Pts',(-40.5718174239661,37.1918449563019,39.1269710600356));
#25979=CARTESIAN_POINT('Ctrl Pts',(-38.1617009122515,36.0575623125548,36.3251892428041));
#25980=CARTESIAN_POINT('Ctrl Pts',(-38.2151985657498,36.0493560734031,36.387790684347));
#25981=CARTESIAN_POINT('Ctrl Pts',(-38.2687839975976,36.0431937832001,36.4505850367912));
#25982=CARTESIAN_POINT('Ctrl Pts',(-38.3223911778814,36.039083033096,36.5134949225584));
#25983=CARTESIAN_POINT('Ctrl Pts',(-38.3759507574777,36.0349759331473,36.5763489472675));
#25984=CARTESIAN_POINT('Ctrl Pts',(-38.4295320360924,36.0329167323991,36.6393182875267));
#25985=CARTESIAN_POINT('Ctrl Pts',(-38.4830691061556,36.0329079637685,36.702325487995));
#25986=CARTESIAN_POINT('Ctrl Pts',(-38.5366061762187,36.0328991951379,36.7653326884632));
#25987=CARTESIAN_POINT('Ctrl Pts',(-38.5900990269231,36.0349408586266,36.8283777364218));
#25988=CARTESIAN_POINT('Ctrl Pts',(-38.6434818594694,36.0390304428894,36.8913830834058));
#25989=CARTESIAN_POINT('Ctrl Pts',(-38.6968646920157,36.0431200271523,36.9543884303896));
#25990=CARTESIAN_POINT('Ctrl Pts',(-38.750137495628,36.0492575313638,37.0173540636806));
#25991=CARTESIAN_POINT('Ctrl Pts',(-38.8032347421755,36.0574354060963,37.0802025324973));
#25992=CARTESIAN_POINT('Ctrl Pts',(-38.856331988723,36.0656132808288,37.143051001314));
#25993=CARTESIAN_POINT('Ctrl Pts',(-38.9092536674875,36.0758315244315,37.2057822929699));
#25994=CARTESIAN_POINT('Ctrl Pts',(-38.9619346822386,36.0880775679694,37.2683192449354));
#25995=CARTESIAN_POINT('Ctrl Pts',(-39.0146156969898,36.1003236115073,37.3308561969009));
#25996=CARTESIAN_POINT('Ctrl Pts',(-39.0670560370872,36.1145974525074,37.3931987965509));
#25997=CARTESIAN_POINT('Ctrl Pts',(-39.1191911983832,36.1308815334554,37.4552703594684));
#25998=CARTESIAN_POINT('Ctrl Pts',(-39.1713263596792,36.1471656144034,37.517341922386));
#25999=CARTESIAN_POINT('Ctrl Pts',(-39.2231563316488,36.1654599320122,37.579142436041));
#26000=CARTESIAN_POINT('Ctrl Pts',(-39.2746173609027,36.1857419833824,37.6405958828037));
#26001=CARTESIAN_POINT('Ctrl Pts',(-39.3260783901567,36.2060240347524,37.7020493295664));
#26002=CARTESIAN_POINT('Ctrl Pts',(-39.3771704663128,36.2282938157907,37.7631556970329));
#26003=CARTESIAN_POINT('Ctrl Pts',(-39.4278307436407,36.2525239335868,37.8238398214092));
#26004=CARTESIAN_POINT('Ctrl Pts',(-39.4784910209687,36.276754051383,37.8845239457855));
#26005=CARTESIAN_POINT('Ctrl Pts',(-39.5287194892421,36.302944501046,37.9447858148217));
#26006=CARTESIAN_POINT('Ctrl Pts',(-39.5784543650103,36.3310630670532,38.0045513034978));
#26007=CARTESIAN_POINT('Ctrl Pts',(-39.6281892407785,36.3591816330604,38.0643167921739));
#26008=CARTESIAN_POINT('Ctrl Pts',(-39.6774305139982,36.3892283097345,38.1235858884251));
#26009=CARTESIAN_POINT('Ctrl Pts',(-39.726117615524,36.4211661382093,38.182285688391));
#26010=CARTESIAN_POINT('Ctrl Pts',(-39.7748047170498,36.453103966684,38.2409854883569));
#26011=CARTESIAN_POINT('Ctrl Pts',(-39.8229376370528,36.4869329405122,38.2991159801882));
#26012=CARTESIAN_POINT('Ctrl Pts',(-39.870457169702,36.5226114484139,38.3566056605612));
#26013=CARTESIAN_POINT('Ctrl Pts',(-39.9179767023511,36.5582899563156,38.4140953409343));
#26014=CARTESIAN_POINT('Ctrl Pts',(-39.9648828380547,36.595817991089,38.4709441982441));
#26015=CARTESIAN_POINT('Ctrl Pts',(-40.0111178799974,36.6351493914341,38.5270823056415));
#26016=CARTESIAN_POINT('Ctrl Pts',(-40.0573529219401,36.6744807917791,38.5832204130388));
#26017=CARTESIAN_POINT('Ctrl Pts',(-40.102916860788,36.7156155497563,38.6386477591913));
#26018=CARTESIAN_POINT('Ctrl Pts',(-40.1477536506837,36.7585030676174,38.6932961657759));
#26019=CARTESIAN_POINT('Ctrl Pts',(-40.1925904405793,36.8013905854786,38.7479445723606));
#26020=CARTESIAN_POINT('Ctrl Pts',(-40.2367000724727,36.8460308545666,38.8018140283461));
#26021=CARTESIAN_POINT('Ctrl Pts',(-40.2800282893812,36.8923689651881,38.8548382716906));
#26022=CARTESIAN_POINT('Ctrl Pts',(-40.3233565062898,36.9387070758096,38.9078625150351));
#26023=CARTESIAN_POINT('Ctrl Pts',(-40.3659032994663,36.9867430186105,38.960041535035));
#26024=CARTESIAN_POINT('Ctrl Pts',(-40.4076163342913,37.0364177070515,39.0113111489662));
#26025=CARTESIAN_POINT('Ctrl Pts',(-40.4493293691164,37.0860923954925,39.0625807628974));
#26026=CARTESIAN_POINT('Ctrl Pts',(-40.4902086371704,37.1374058195468,39.1129409604106));
#26027=CARTESIAN_POINT('Ctrl Pts',(-40.5302038549723,37.1902948612154,39.1623297960218));
#26028=CARTESIAN_POINT('Ctrl Pts',(-38.0705964434674,36.0634391745925,36.3043797741951));
#26029=CARTESIAN_POINT('Ctrl Pts',(-38.125068881183,36.053839610039,36.3680388407926));
#26030=CARTESIAN_POINT('Ctrl Pts',(-38.1796527647013,36.0463584337675,36.4319212158031));
#26031=CARTESIAN_POINT('Ctrl Pts',(-38.2342783318298,36.0410051496582,36.4959452490178));
#26032=CARTESIAN_POINT('Ctrl Pts',(-38.2888553939909,36.0356566190167,36.5599124318634));
#26033=CARTESIAN_POINT('Ctrl Pts',(-38.3434740539323,36.0324322044189,36.6240210075788));
#26034=CARTESIAN_POINT('Ctrl Pts',(-38.3980646307614,36.0313359680253,36.6881891846602));
#26035=CARTESIAN_POINT('Ctrl Pts',(-38.4526552075906,36.0302397316317,36.7523573617416));
#26036=CARTESIAN_POINT('Ctrl Pts',(-38.5072176894685,36.0312716736637,36.8165851262716));
#26037=CARTESIAN_POINT('Ctrl Pts',(-38.5616824687255,36.0344304296258,36.8807905366098));
#26038=CARTESIAN_POINT('Ctrl Pts',(-38.6161472479825,36.0375891855878,36.944995946948));
#26039=CARTESIAN_POINT('Ctrl Pts',(-38.6705143128074,36.0428747547796,37.0091789891697));
#26040=CARTESIAN_POINT('Ctrl Pts',(-38.724714306159,36.0502803496406,37.0732577803462));
#26041=CARTESIAN_POINT('Ctrl Pts',(-38.7789142995106,36.0576859445016,37.1373365715227));
#26042=CARTESIAN_POINT('Ctrl Pts',(-38.8329472096354,36.0672115634119,37.2013110977573));
#26043=CARTESIAN_POINT('Ctrl Pts',(-38.8867441068837,36.0788450131507,37.2650997435283));
#26044=CARTESIAN_POINT('Ctrl Pts',(-38.940541004132,36.0904784628896,37.3288883892993));
#26045=CARTESIAN_POINT('Ctrl Pts',(-38.9941018768322,36.1042197409205,37.3924911407721));
#26046=CARTESIAN_POINT('Ctrl Pts',(-39.0473583984096,36.120051279538,37.4558268578443));
#26047=CARTESIAN_POINT('Ctrl Pts',(-39.100614919987,36.1358828181555,37.5191625749165));
#26048=CARTESIAN_POINT('Ctrl Pts',(-39.1535670788927,36.1538046139148,37.582231243853));
#26049=CARTESIAN_POINT('Ctrl Pts',(-39.206147325724,36.1737937694826,37.6449524067597));
#26050=CARTESIAN_POINT('Ctrl Pts',(-39.2587275725553,36.1937829250503,37.7076735696665));
#26051=CARTESIAN_POINT('Ctrl Pts',(-39.3109358959166,36.2158394360822,37.7700472129432));
#26052=CARTESIAN_POINT('Ctrl Pts',(-39.3627056957615,36.2399351340599,37.8319937659655));
#26053=CARTESIAN_POINT('Ctrl Pts',(-39.4144754956064,36.2640308320376,37.8939403189879));
#26054=CARTESIAN_POINT('Ctrl Pts',(-39.4658067607094,36.2901657117264,37.9554597683227));
#26055=CARTESIAN_POINT('Ctrl Pts',(-39.5166340100992,36.3183064052841,38.0164736334055));
#26056=CARTESIAN_POINT('Ctrl Pts',(-39.567461259489,36.3464470988418,38.0774874984883));
#26057=CARTESIAN_POINT('Ctrl Pts',(-39.6177844821409,36.3765936001565,38.1379957660878));
#26058=CARTESIAN_POINT('Ctrl Pts',(-39.6675394830426,36.4087074271696,38.1979212457141));
#26059=CARTESIAN_POINT('Ctrl Pts',(-39.7172944839443,36.4408212541828,38.2578467253403));
#26060=CARTESIAN_POINT('Ctrl Pts',(-39.7664812523064,36.4749023999232,38.3171894039982));
#26061=CARTESIAN_POINT('Ctrl Pts',(-39.8150370426548,36.510907366241,38.3758735779943));
#26062=CARTESIAN_POINT('Ctrl Pts',(-39.8635928330032,36.5469123325587,38.4345577519904));
#26063=CARTESIAN_POINT('Ctrl Pts',(-39.9115176348099,36.58484111164,38.4925834085993));
#26064=CARTESIAN_POINT('Ctrl Pts',(-39.9587503120694,36.6246453001592,38.5498765238635));
#26065=CARTESIAN_POINT('Ctrl Pts',(-40.0059829893289,36.6644494886784,38.6071696391278));
#26066=CARTESIAN_POINT('Ctrl Pts',(-40.0525235317984,36.7061290779986,38.6637302006231));
#26067=CARTESIAN_POINT('Ctrl Pts',(-40.0983125687262,36.7496308830115,38.7194860527826));
#26068=CARTESIAN_POINT('Ctrl Pts',(-40.1441016056541,36.7931326880244,38.7752419049421));
#26069=CARTESIAN_POINT('Ctrl Pts',(-40.1891391271119,36.8384566992927,38.8301930356747));
#26070=CARTESIAN_POINT('Ctrl Pts',(-40.2333676789247,36.8855450855121,38.8842693417014));
#26071=CARTESIAN_POINT('Ctrl Pts',(-40.2775962307375,36.9326334717315,38.938345647728));
#26072=CARTESIAN_POINT('Ctrl Pts',(-40.3210158033137,36.9814862226874,38.9915471173214));
#26073=CARTESIAN_POINT('Ctrl Pts',(-40.3635710054698,37.0320410082882,39.0438058781573));
#26074=CARTESIAN_POINT('Ctrl Pts',(-40.4061262076258,37.0825957938891,39.0960646389932));
#26075=CARTESIAN_POINT('Ctrl Pts',(-40.4478170301341,37.1348526031702,39.1473806797382));
#26076=CARTESIAN_POINT('Ctrl Pts',(-40.4885902859785,37.1887447661289,39.197688532008));
#26077=CARTESIAN_POINT('Ctrl Pts',(-37.9807359148445,36.0708539957089,36.2849451673821));
#26078=CARTESIAN_POINT('Ctrl Pts',(-38.0361388636876,36.0598245864939,36.349611657568));
#26079=CARTESIAN_POINT('Ctrl Pts',(-38.0916787515611,36.0509875068319,36.4145339633157));
#26080=CARTESIAN_POINT('Ctrl Pts',(-38.1472819813364,36.044354405607,36.4796260509332));
#26081=CARTESIAN_POINT('Ctrl Pts',(-38.202835838025,36.0377271942682,36.5446603397988));
#26082=CARTESIAN_POINT('Ctrl Pts',(-38.2584529112245,36.0333000505676,36.609864093988));
#26083=CARTESIAN_POINT('Ctrl Pts',(-38.314059634525,36.0310787757327,36.675151063009));
#26084=CARTESIAN_POINT('Ctrl Pts',(-38.3696663578256,36.0288575008977,36.74043803203));
#26085=CARTESIAN_POINT('Ctrl Pts',(-38.4252627182639,36.0288420954269,36.8058082006614));
#26086=CARTESIAN_POINT('Ctrl Pts',(-38.4807751786657,36.0310325287199,36.8711751005551));
#26087=CARTESIAN_POINT('Ctrl Pts',(-38.5362876390675,36.033222962013,36.9365420004487));
#26088=CARTESIAN_POINT('Ctrl Pts',(-38.5917161864921,36.0376192335413,37.0019056163654));
#26089=CARTESIAN_POINT('Ctrl Pts',(-38.646987507313,36.0442154811027,37.0671794905916));
#26090=CARTESIAN_POINT('Ctrl Pts',(-38.7022588281338,36.0508117286641,37.1324533648177));
#26091=CARTESIAN_POINT('Ctrl Pts',(-38.7573729094671,36.0596079507043,37.1976374821365));
#26092=CARTESIAN_POINT('Ctrl Pts',(-38.8122568549514,36.0705924690439,37.2626456239265));
#26093=CARTESIAN_POINT('Ctrl Pts',(-38.8671408004357,36.0815769873834,37.3276537657165));
#26094=CARTESIAN_POINT('Ctrl Pts',(-38.9217945972781,36.0947497994464,37.3924859168235));
#26095=CARTESIAN_POINT('Ctrl Pts',(-38.9761459589933,36.1100934420574,37.4570563255389));
#26096=CARTESIAN_POINT('Ctrl Pts',(-39.0304973207086,36.1254370846684,37.5216267342543));
#26097=CARTESIAN_POINT('Ctrl Pts',(-39.0845462346282,36.1429515542368,37.5859353855265));
#26098=CARTESIAN_POINT('Ctrl Pts',(-39.1382212151398,36.1626136488479,37.6498972211433));
#26099=CARTESIAN_POINT('Ctrl Pts',(-39.1918961956515,36.182275743459,37.7138590567601));
#26100=CARTESIAN_POINT('Ctrl Pts',(-39.2451972302446,36.2040854585169,37.777474061812));
#26101=CARTESIAN_POINT('Ctrl Pts',(-39.2980538230577,36.2280139147768,37.840658096331));
#26102=CARTESIAN_POINT('Ctrl Pts',(-39.3509104158708,36.2519423710367,37.9038421308499));
#26103=CARTESIAN_POINT('Ctrl Pts',(-39.403322554584,36.2779895629094,37.966595180108));
#26104=CARTESIAN_POINT('Ctrl Pts',(-39.4552209193481,36.3061210102197,38.0288342447005));
#26105=CARTESIAN_POINT('Ctrl Pts',(-39.5071192841123,36.3342524575298,38.091073309293));
#26106=CARTESIAN_POINT('Ctrl Pts',(-39.558503862831,36.3644681537101,38.1527983747124));
#26107=CARTESIAN_POINT('Ctrl Pts',(-39.6093066948198,36.3967281088421,38.2139278014215));
#26108=CARTESIAN_POINT('Ctrl Pts',(-39.6601095268087,36.4289880639741,38.2750572281306));
#26109=CARTESIAN_POINT('Ctrl Pts',(-39.7103306002267,36.4632922705294,38.3355910018807));
#26110=CARTESIAN_POINT('Ctrl Pts',(-39.7599034931162,36.4995953345826,38.3954490587125));
#26111=CARTESIAN_POINT('Ctrl Pts',(-39.8094763860058,36.5358983986359,38.4553071155443));
#26112=CARTESIAN_POINT('Ctrl Pts',(-39.8584010868125,36.5742003117175,38.5144894415054));
#26113=CARTESIAN_POINT('Ctrl Pts',(-39.9066128878016,36.6144503958987,38.5729177597622));
#26114=CARTESIAN_POINT('Ctrl Pts',(-39.9548246887907,36.65470048008,38.631346078019));
#26115=CARTESIAN_POINT('Ctrl Pts',(-40.0023235787247,36.6968987259727,38.689020374952));
#26116=CARTESIAN_POINT('Ctrl Pts',(-40.0490467350601,36.7409893056005,38.7458643676801));
#26117=CARTESIAN_POINT('Ctrl Pts',(-40.0957698913955,36.7850798852282,38.8027083604082));
#26118=CARTESIAN_POINT('Ctrl Pts',(-40.1417173032415,36.8310627883089,38.8587220356807));
#26119=CARTESIAN_POINT('Ctrl Pts',(-40.1868281992345,36.878877184372,38.9138313061286));
#26120=CARTESIAN_POINT('Ctrl Pts',(-40.2319390952273,36.9266915804353,38.9689405765764));
#26121=CARTESIAN_POINT('Ctrl Pts',(-40.2762134648518,36.976337458332,39.0231454293531));
#26122=CARTESIAN_POINT('Ctrl Pts',(-40.3195927484955,37.0277491458603,39.0763741683628));
#26123=CARTESIAN_POINT('Ctrl Pts',(-40.3629720321391,37.0791608333887,39.1296029073724));
#26124=CARTESIAN_POINT('Ctrl Pts',(-40.4054562196899,37.1323383185621,39.1818555202063));
#26125=CARTESIAN_POINT('Ctrl Pts',(-40.4469891180173,37.1872112609937,39.2330628914883));
#26126=CARTESIAN_POINT('Ctrl Pts',(-37.8919774678215,36.0796223244832,36.2667225297271));
#26127=CARTESIAN_POINT('Ctrl Pts',(-37.9482699971579,36.067131319434,36.3323499709714));
#26128=CARTESIAN_POINT('Ctrl Pts',(-38.0047267235371,36.0569059654783,36.3982677820133));
#26129=CARTESIAN_POINT('Ctrl Pts',(-38.0612701224292,36.0489603009388,36.4643854465506));
#26130=CARTESIAN_POINT('Ctrl Pts',(-38.1177633134081,36.0410216917806,36.5304444016712));
#26131=CARTESIAN_POINT('Ctrl Pts',(-38.1743430088834,36.0353587273096,36.596702838963));
#26132=CARTESIAN_POINT('Ctrl Pts',(-38.2309316534887,36.0319791699089,36.6630699361382));
#26133=CARTESIAN_POINT('Ctrl Pts',(-38.2875202980941,36.0285996125084,36.7294370333135));
#26134=CARTESIAN_POINT('Ctrl Pts',(-38.3441178776431,36.0275034630254,36.7959127737345));
#26135=CARTESIAN_POINT('Ctrl Pts',(-38.4006468122553,36.0286922239828,36.8624060372502));
#26136=CARTESIAN_POINT('Ctrl Pts',(-38.4571757468675,36.0298809849402,36.9288993007659));
#26137=CARTESIAN_POINT('Ctrl Pts',(-38.5136360223715,36.03335465604,36.9954100707068));
#26138=CARTESIAN_POINT('Ctrl Pts',(-38.5699502470932,36.0391084758241,37.0618471789059));
#26139=CARTESIAN_POINT('Ctrl Pts',(-38.6262644718148,36.0448622956084,37.128284287105));
#26140=CARTESIAN_POINT('Ctrl Pts',(-38.6824326316366,36.0528962626346,37.194647716907));
#26141=CARTESIAN_POINT('Ctrl Pts',(-38.7383777352955,36.0631993645204,37.260846502108));
#26142=CARTESIAN_POINT('Ctrl Pts',(-38.7943228389544,36.073502466406,37.3270452873091));
#26143=CARTESIAN_POINT('Ctrl Pts',(-38.8500448724255,36.0860747005682,37.3930794113136));
#26144=CARTESIAN_POINT('Ctrl Pts',(-38.9054674559635,36.1008988338949,37.4588583593065));
#26145=CARTESIAN_POINT('Ctrl Pts',(-38.9608900395015,36.1157229672217,37.5246373072994));
#26146=CARTESIAN_POINT('Ctrl Pts',(-39.0160131592125,36.1327989959966,37.5901610627903));
#26147=CARTESIAN_POINT('Ctrl Pts',(-39.0707612562991,36.152103513631,37.6553398105404));
#26148=CARTESIAN_POINT('Ctrl Pts',(-39.1255093533857,36.1714080312654,37.7205185582905));
#26149=CARTESIAN_POINT('Ctrl Pts',(-39.179882414123,36.1929410329197,37.7853522819599));
#26150=CARTESIAN_POINT('Ctrl Pts',(-39.2338059078403,36.2166730027081,37.8497521121557));
#26151=CARTESIAN_POINT('Ctrl Pts',(-39.2877294015577,36.2404049724964,37.9141519423515));
#26152=CARTESIAN_POINT('Ctrl Pts',(-39.3412033147369,36.2663359044695,37.9781178629291));
#26153=CARTESIAN_POINT('Ctrl Pts',(-39.394154349194,36.2944302543756,38.0415621940174));
#26154=CARTESIAN_POINT('Ctrl Pts',(-39.447105383651,36.3225246042818,38.1050065251057));
#26155=CARTESIAN_POINT('Ctrl Pts',(-39.4995335261116,36.352782365078,38.1679292507998));
#26156=CARTESIAN_POINT('Ctrl Pts',(-39.5513669118587,36.3851620616078,38.2302441211647));
#26157=CARTESIAN_POINT('Ctrl Pts',(-39.6032002976058,36.4175417581375,38.2925589915297));
#26158=CARTESIAN_POINT('Ctrl Pts',(-39.6544389136452,36.4520433822834,38.3542659909437));
#26159=CARTESIAN_POINT('Ctrl Pts',(-39.7050125257772,36.4886196417072,38.4152805359019));
#26160=CARTESIAN_POINT('Ctrl Pts',(-39.7555861379091,36.5251959011311,38.4762950808601));
#26161=CARTESIAN_POINT('Ctrl Pts',(-39.8054947334551,36.5638467866634,38.5366171560666));
#26162=CARTESIAN_POINT('Ctrl Pts',(-39.8546699013115,36.6045193184576,38.5961640763708));
#26163=CARTESIAN_POINT('Ctrl Pts',(-39.9038450691679,36.6451918502518,38.655710996675));
#26164=CARTESIAN_POINT('Ctrl Pts',(-39.9522867970068,36.6878860181116,38.7144827471489));
#26165=CARTESIAN_POINT('Ctrl Pts',(-39.9999286844011,36.7325432999504,38.7723987677153));
#26166=CARTESIAN_POINT('Ctrl Pts',(-40.0475705717954,36.7772005817894,38.8303147882816));
#26167=CARTESIAN_POINT('Ctrl Pts',(-40.0944126068016,36.8238209664121,38.8873750644213));
#26168=CARTESIAN_POINT('Ctrl Pts',(-40.140390581736,36.8723405499575,38.9435013820225));
#26169=CARTESIAN_POINT('Ctrl Pts',(-40.1863685566705,36.9208601335028,38.9996276996238));
#26170=CARTESIAN_POINT('Ctrl Pts',(-40.2314824600069,36.9712789038072,39.0548200446163));
#26171=CARTESIAN_POINT('Ctrl Pts',(-40.2756704528598,37.0235277504564,39.1090027633136));
#26172=CARTESIAN_POINT('Ctrl Pts',(-40.3198584457128,37.0757765971056,39.1631854820109));
#26173=CARTESIAN_POINT('Ctrl Pts',(-40.3631205170047,37.129855507001,39.2163585608298));
#26174=CARTESIAN_POINT('Ctrl Pts',(-40.4053973662082,37.1856903526729,39.2684491139483));
#26175=CARTESIAN_POINT('Ctrl Pts',(-37.8032190207985,36.0883906532575,36.248499892072));
#26176=CARTESIAN_POINT('Ctrl Pts',(-37.8604011306282,36.0744380523741,36.3150882843748));
#26177=CARTESIAN_POINT('Ctrl Pts',(-37.9177746955132,36.0628244241247,36.382001600711));
#26178=CARTESIAN_POINT('Ctrl Pts',(-37.975258263522,36.0535661962707,36.4491448421679));
#26179=CARTESIAN_POINT('Ctrl Pts',(-38.0326907887911,36.0443161892931,36.5162284635436));
#26180=CARTESIAN_POINT('Ctrl Pts',(-38.0902331065422,36.0374174040515,36.5835415839379));
#26181=CARTESIAN_POINT('Ctrl Pts',(-38.1478036724524,36.0328795640852,36.6509888092675));
#26182=CARTESIAN_POINT('Ctrl Pts',(-38.2053742383626,36.028341724119,36.7184360345971));
#26183=CARTESIAN_POINT('Ctrl Pts',(-38.2629730370223,36.0261648306239,36.7860173468077));
#26184=CARTESIAN_POINT('Ctrl Pts',(-38.3205184458449,36.0263519192456,36.8536369739454));
#26185=CARTESIAN_POINT('Ctrl Pts',(-38.3780638546675,36.0265390078675,36.921256601083));
#26186=CARTESIAN_POINT('Ctrl Pts',(-38.4355558582509,36.0290900785386,36.9889145250481));
#26187=CARTESIAN_POINT('Ctrl Pts',(-38.4929129868733,36.0340014705456,37.0565148672202));
#26188=CARTESIAN_POINT('Ctrl Pts',(-38.5502701154958,36.0389128625527,37.1241152093923));
#26189=CARTESIAN_POINT('Ctrl Pts',(-38.6074923538061,36.046184574565,37.1916579516774));
#26190=CARTESIAN_POINT('Ctrl Pts',(-38.6644986156396,36.0558062599968,37.2590473802896));
#26191=CARTESIAN_POINT('Ctrl Pts',(-38.7215048774731,36.0654279454286,37.3264368089017));
#26192=CARTESIAN_POINT('Ctrl Pts',(-38.7782951475729,36.07739960169,37.3936729058038));
#26193=CARTESIAN_POINT('Ctrl Pts',(-38.8347889529337,36.0917042257324,37.4606603930742));
#26194=CARTESIAN_POINT('Ctrl Pts',(-38.8912827582945,36.1060088497749,37.5276478803445));
#26195=CARTESIAN_POINT('Ctrl Pts',(-38.9474800837969,36.1226464377564,37.5943867400541));
#26196=CARTESIAN_POINT('Ctrl Pts',(-39.0033012974584,36.141593378414,37.6607823999375));
#26197=CARTESIAN_POINT('Ctrl Pts',(-39.0591225111199,36.1605403190717,37.7271780598209));
#26198=CARTESIAN_POINT('Ctrl Pts',(-39.1145675980014,36.1817966073224,37.7932305021078));
#26199=CARTESIAN_POINT('Ctrl Pts',(-39.1695579926229,36.2053320906394,37.8588461279804));
#26200=CARTESIAN_POINT('Ctrl Pts',(-39.2245483872446,36.2288675739563,37.924461753853));
#26201=CARTESIAN_POINT('Ctrl Pts',(-39.2790840748897,36.2546822460295,37.9896405457502));
#26202=CARTESIAN_POINT('Ctrl Pts',(-39.3330877790397,36.2827394985316,38.0542901433343));
#26203=CARTESIAN_POINT('Ctrl Pts',(-39.3870914831897,36.3107967510337,38.1189397409185));
#26204=CARTESIAN_POINT('Ctrl Pts',(-39.4405631893923,36.3410965764458,38.1830601268872));
#26205=CARTESIAN_POINT('Ctrl Pts',(-39.4934271288977,36.3735960143734,38.246560440908));
#26206=CARTESIAN_POINT('Ctrl Pts',(-39.546291068403,36.4060954523009,38.3100607549287));
#26207=CARTESIAN_POINT('Ctrl Pts',(-39.5985472270638,36.4407944940374,38.3729409800067));
#26208=CARTESIAN_POINT('Ctrl Pts',(-39.6501215584381,36.4776439488319,38.4351120130913));
#26209=CARTESIAN_POINT('Ctrl Pts',(-39.7016958898123,36.5144934036264,38.4972830461759));
#26210=CARTESIAN_POINT('Ctrl Pts',(-39.7525883800977,36.5534932616094,38.5587448706279));
#26211=CARTESIAN_POINT('Ctrl Pts',(-39.8027269148214,36.5945882410166,38.6194103929794));
#26212=CARTESIAN_POINT('Ctrl Pts',(-39.8528654495451,36.6356832204237,38.680075915331));
#26213=CARTESIAN_POINT('Ctrl Pts',(-39.9022500152889,36.6788733102505,38.7399451193458));
#26214=CARTESIAN_POINT('Ctrl Pts',(-39.9508106337421,36.7240972943005,38.7989331677504));
#26215=CARTESIAN_POINT('Ctrl Pts',(-39.9993712521953,36.7693212783505,38.8579212161551));
#26216=CARTESIAN_POINT('Ctrl Pts',(-40.0471079103616,36.8165791445153,38.9160280931619));
#26217=CARTESIAN_POINT('Ctrl Pts',(-40.0939529642376,36.8658039155428,38.9731714579166));
#26218=CARTESIAN_POINT('Ctrl Pts',(-40.1407980181136,36.9150286865703,39.0303148226713));
#26219=CARTESIAN_POINT('Ctrl Pts',(-40.1867514551618,36.9662203492825,39.0864946598795));
#26220=CARTESIAN_POINT('Ctrl Pts',(-40.2317481572241,37.0193063550525,39.1416313582644));
#26221=CARTESIAN_POINT('Ctrl Pts',(-40.2767448592865,37.0723923608224,39.1967680566494));
#26222=CARTESIAN_POINT('Ctrl Pts',(-40.3207848143196,37.1273726954398,39.2508616014532));
#26223=CARTESIAN_POINT('Ctrl Pts',(-40.363805614399,37.184169444352,39.3038353364083));
#26224=CARTESIAN_POINT('Ctrl Pts',(-37.7155633104343,36.0985133588211,36.2314899874893));
#26225=CARTESIAN_POINT('Ctrl Pts',(-37.7735940555694,36.0830673910403,36.2989928414705));
#26226=CARTESIAN_POINT('Ctrl Pts',(-37.8318452786789,36.0700330978996,36.3668572209427));
#26227=CARTESIAN_POINT('Ctrl Pts',(-37.8902315079545,36.0594295410209,36.4349835452439));
#26228=CARTESIAN_POINT('Ctrl Pts',(-37.948565892969,36.0488353996083,36.5030493765319));
#26229=CARTESIAN_POINT('Ctrl Pts',(-38.0070350278182,36.0406676826179,36.5713766682024));
#26230=CARTESIAN_POINT('Ctrl Pts',(-38.0655532757724,36.0349382968221,36.6398653415568));
#26231=CARTESIAN_POINT('Ctrl Pts',(-38.1240715237266,36.0292089110264,36.7083540149113));
#26232=CARTESIAN_POINT('Ctrl Pts',(-38.1826388680546,36.0259178580415,36.7770040503664));
#26233=CARTESIAN_POINT('Ctrl Pts',(-38.2411695302526,36.0250699058513,36.8457148990595));
#26234=CARTESIAN_POINT('Ctrl Pts',(-38.2997001924505,36.0242219536612,36.9144257477526));
#26235=CARTESIAN_POINT('Ctrl Pts',(-38.3581941557842,36.025817102488,36.9831973900379));
#26236=CARTESIAN_POINT('Ctrl Pts',(-38.4165657510128,36.0298529677364,37.0519291011623));
#26237=CARTESIAN_POINT('Ctrl Pts',(-38.4749373462413,36.0338888329847,37.1206608122868));
#26238=CARTESIAN_POINT('Ctrl Pts',(-38.5331865566767,36.0403654134821,37.1893525725995));
#26239=CARTESIAN_POINT('Ctrl Pts',(-38.5912280730533,36.0492731791837,37.2579037762394));
#26240=CARTESIAN_POINT('Ctrl Pts',(-38.6492695894299,36.0581809448852,37.3264549798792));
#26241=CARTESIAN_POINT('Ctrl Pts',(-38.7071033951548,36.069519893227,37.3948656072474));
#26242=CARTESIAN_POINT('Ctrl Pts',(-38.7646447905916,36.0832733767442,37.4630354658025));
#26243=CARTESIAN_POINT('Ctrl Pts',(-38.8221861860284,36.0970268602613,37.5312053243577));
#26244=CARTESIAN_POINT('Ctrl Pts',(-38.8794351547276,36.1131948750061,37.5991343946107));
#26245=CARTESIAN_POINT('Ctrl Pts',(-38.9363078545486,36.1317537049394,37.6667231905533));
#26246=CARTESIAN_POINT('Ctrl Pts',(-38.9931805543695,36.1503125348727,37.7343119864959));
#26247=CARTESIAN_POINT('Ctrl Pts',(-39.0496769690542,36.1712621746747,37.8015604888055));
#26248=CARTESIAN_POINT('Ctrl Pts',(-39.1057143593112,36.194571909252,37.8683702091491));
#26249=CARTESIAN_POINT('Ctrl Pts',(-39.1617517495681,36.2178816438295,37.9351799294927));
#26250=CARTESIAN_POINT('Ctrl Pts',(-39.2173300993782,36.2435514665059,38.0015508487707));
#26251=CARTESIAN_POINT('Ctrl Pts',(-39.2723680144236,36.2715437531241,38.0673857645443));
#26252=CARTESIAN_POINT('Ctrl Pts',(-39.3274059294689,36.2995360397424,38.1332206803179));
#26253=CARTESIAN_POINT('Ctrl Pts',(-39.3819033940163,36.3298507822888,38.1985195737665));
#26254=CARTESIAN_POINT('Ctrl Pts',(-39.4357805969077,36.3624435577397,38.2631868128));
#26255=CARTESIAN_POINT('Ctrl Pts',(-39.4896577997992,36.3950363331905,38.3278540518334));
#26256=CARTESIAN_POINT('Ctrl Pts',(-39.5429147256334,36.4299071322184,38.3918896179649));
#26257=CARTESIAN_POINT('Ctrl Pts',(-39.5954733799659,36.4670048630141,38.4551997293104));
#26258=CARTESIAN_POINT('Ctrl Pts',(-39.6480320342983,36.5041025938097,38.5185098406561));
#26259=CARTESIAN_POINT('Ctrl Pts',(-39.6998924021046,36.5434272457595,38.5810944791169));
#26260=CARTESIAN_POINT('Ctrl Pts',(-39.7509785338906,36.5849212078543,38.6428619874586));
#26261=CARTESIAN_POINT('Ctrl Pts',(-39.8020646656766,36.6264151699492,38.7046294958002));
#26262=CARTESIAN_POINT('Ctrl Pts',(-39.8523765468386,36.67007843032,38.7655798563646));
#26263=CARTESIAN_POINT('Ctrl Pts',(-39.9018404950872,36.7158470274101,38.8256238047931));
#26264=CARTESIAN_POINT('Ctrl Pts',(-39.9513044433358,36.7616156245003,38.8856677532216));
#26265=CARTESIAN_POINT('Ctrl Pts',(-39.9999204445307,36.80948954522,38.9448052723487));
#26266=CARTESIAN_POINT('Ctrl Pts',(-40.0476172992077,36.8593986646901,39.0029497519172));
#26267=CARTESIAN_POINT('Ctrl Pts',(-40.0953141538847,36.9093077841602,39.0610942314857));
#26268=CARTESIAN_POINT('Ctrl Pts',(-40.1420918484084,36.9612520881088,39.1182456548728));
#26269=CARTESIAN_POINT('Ctrl Pts',(-40.1878818744981,37.0151554935858,39.1743203193843));
#26270=CARTESIAN_POINT('Ctrl Pts',(-40.2336719005877,37.0690588990627,39.2303949838959));
#26271=CARTESIAN_POINT('Ctrl Pts',(-40.2784742451523,37.1249213906555,39.2853928735001));
#26272=CARTESIAN_POINT('Ctrl Pts',(-40.3222232915804,37.1826611500204,39.3392334380224));
#26273=CARTESIAN_POINT('Ctrl Pts',(-37.6288986882551,36.1098451974354,36.2155645638857));
#26274=CARTESIAN_POINT('Ctrl Pts',(-37.6877397713873,36.092877953765,36.2839383179962));
#26275=CARTESIAN_POINT('Ctrl Pts',(-37.7468320665581,36.078394354814,36.3527121922699));
#26276=CARTESIAN_POINT('Ctrl Pts',(-37.8060859993744,36.0664163519574,36.4217819364555));
#26277=CARTESIAN_POINT('Ctrl Pts',(-37.8652873174493,36.0544489850114,36.4907903499148));
#26278=CARTESIAN_POINT('Ctrl Pts',(-37.9246499681569,36.0449827700856,36.5600940869988));
#26279=CARTESIAN_POINT('Ctrl Pts',(-37.9840841272394,36.0380320309295,36.6295882811515));
#26280=CARTESIAN_POINT('Ctrl Pts',(-38.043518286322,36.0310812917733,36.6990824753041));
#26281=CARTESIAN_POINT('Ctrl Pts',(-38.1030239356216,36.0266460305104,36.7687671052939));
#26282=CARTESIAN_POINT('Ctrl Pts',(-38.1625110345032,36.0247329583309,36.8385367282189));
#26283=CARTESIAN_POINT('Ctrl Pts',(-38.2219981333846,36.0228198861515,36.9083063511438));
#26284=CARTESIAN_POINT('Ctrl Pts',(-38.2814666636739,36.02342900364,36.9781609456884));
#26285=CARTESIAN_POINT('Ctrl Pts',(-38.340826640902,36.026559389114,37.0479948117696));
#26286=CARTESIAN_POINT('Ctrl Pts',(-38.4001866181302,36.0296897745879,37.1178286778509));
#26287=CARTESIAN_POINT('Ctrl Pts',(-38.459438024162,36.0353414270909,37.1876417941335));
#26288=CARTESIAN_POINT('Ctrl Pts',(-38.518491203069,36.0435057948568,37.2573285232974));
#26289=CARTESIAN_POINT('Ctrl Pts',(-38.577544381976,36.0516701626229,37.3270152524612));
#26290=CARTESIAN_POINT('Ctrl Pts',(-38.6363993157166,36.0623472431577,37.3965755732159));
#26291=CARTESIAN_POINT('Ctrl Pts',(-38.6949669482823,36.0755208804975,37.4659042307574));
#26292=CARTESIAN_POINT('Ctrl Pts',(-38.7535345808479,36.0886945178373,37.5352328882988));
#26293=CARTESIAN_POINT('Ctrl Pts',(-38.8118148943452,36.1043647079574,37.604329861446));
#26294=CARTESIAN_POINT('Ctrl Pts',(-38.869719702249,36.1225077395987,37.6730905965066));
#26295=CARTESIAN_POINT('Ctrl Pts',(-38.9276245101529,36.1406507712399,37.7418513315672));
#26296=CARTESIAN_POINT('Ctrl Pts',(-38.9851537947725,36.1612666388593,37.810275807534));
#26297=CARTESIAN_POINT('Ctrl Pts',(-39.0422205059976,36.1843241476738,37.8782604882997));
#26298=CARTESIAN_POINT('Ctrl Pts',(-39.0992872172227,36.2073816564885,37.9462451690653));
#26299=CARTESIAN_POINT('Ctrl Pts',(-39.1558913376187,36.2328807994539,38.0137900338597));
#26300=CARTESIAN_POINT('Ctrl Pts',(-39.2119472169822,36.2607829926868,38.0807928775543));
#26301=CARTESIAN_POINT('Ctrl Pts',(-39.2680030963459,36.2886851859197,38.1477957212488));
#26302=CARTESIAN_POINT('Ctrl Pts',(-39.3235107175512,36.3189904208956,38.2142565233733));
#26303=CARTESIAN_POINT('Ctrl Pts',(-39.3783860895567,36.3516528414203,38.2800747191427));
#26304=CARTESIAN_POINT('Ctrl Pts',(-39.4332614615622,36.384315261945,38.3458929149119));
#26305=CARTESIAN_POINT('Ctrl Pts',(-39.4875045676025,36.4193348580397,38.4110684842176));
#26306=CARTESIAN_POINT('Ctrl Pts',(-39.54103333003,36.4566586400015,38.4755028070172));
#26307=CARTESIAN_POINT('Ctrl Pts',(-39.5945620924575,36.4939824219634,38.5399371298167));
#26308=CARTESIAN_POINT('Ctrl Pts',(-39.6473764949183,36.5336103783894,38.6036301864247));
#26309=CARTESIAN_POINT('Ctrl Pts',(-39.6993966215995,36.5754825464625,38.6664856000542));
#26310=CARTESIAN_POINT('Ctrl Pts',(-39.7514167482806,36.6173547145356,38.7293410136837));
#26311=CARTESIAN_POINT('Ctrl Pts',(-39.8026425832891,36.6614710814631,38.7913587651315));
#26312=CARTESIAN_POINT('Ctrl Pts',(-39.8529966145439,36.7077648928152,38.8524450125895));
#26313=CARTESIAN_POINT('Ctrl Pts',(-39.9033506457986,36.7540587041673,38.9135312600474));
#26314=CARTESIAN_POINT('Ctrl Pts',(-39.9528328579157,36.8025299458004,38.9736859848527));
#26315=CARTESIAN_POINT('Ctrl Pts',(-40.0013683771669,36.8531052737307,39.0328181642253));
#26316=CARTESIAN_POINT('Ctrl Pts',(-40.0499038964181,36.9036806016611,39.0919503435978));
#26317=CARTESIAN_POINT('Ctrl Pts',(-40.0974927079752,36.9563600004371,39.1500599594719));
#26318=CARTESIAN_POINT('Ctrl Pts',(-40.1440628030983,37.0110637585259,39.2070590836124));
#26319=CARTESIAN_POINT('Ctrl Pts',(-40.1906328982213,37.0657675166147,39.2640582077529));
#26320=CARTESIAN_POINT('Ctrl Pts',(-40.2361842626827,37.1224956173034,39.3199468227458));
#26321=CARTESIAN_POINT('Ctrl Pts',(-40.2806479706938,37.1811622227888,39.3746403610508));
#26322=CARTESIAN_POINT('Ctrl Pts',(-37.4555694438967,36.1325088746638,36.1837137166787));
#26323=CARTESIAN_POINT('Ctrl Pts',(-37.516031203023,36.1124990792145,36.2538292710476));
#26324=CARTESIAN_POINT('Ctrl Pts',(-37.5768056423164,36.0951168686426,36.3244221349243));
#26325=CARTESIAN_POINT('Ctrl Pts',(-37.6377949822143,36.0803899738306,36.3953787188787));
#26326=CARTESIAN_POINT('Ctrl Pts',(-37.6987301664097,36.0656761558176,36.4662722966806));
#26327=CARTESIAN_POINT('Ctrl Pts',(-37.7598798488343,36.053612945021,36.5375289245917));
#26328=CARTESIAN_POINT('Ctrl Pts',(-37.8211458301736,36.0442194991441,36.6090341603408));
#26329=CARTESIAN_POINT('Ctrl Pts',(-37.882411811513,36.0348260532672,36.6805393960898));
#26330=CARTESIAN_POINT('Ctrl Pts',(-37.9437940707557,36.028102375448,36.7522932151489));
#26331=CARTESIAN_POINT('Ctrl Pts',(-38.0051940430043,36.02405906329,36.8241803865376));
#26332=CARTESIAN_POINT('Ctrl Pts',(-38.066594015253,36.020015751132,36.8960675579264));
#26333=CARTESIAN_POINT('Ctrl Pts',(-38.1280116794532,36.0186528059442,36.9680880569896));
#26334=CARTESIAN_POINT('Ctrl Pts',(-38.1893484206806,36.0199722318693,37.0401262329843));
#26335=CARTESIAN_POINT('Ctrl Pts',(-38.2506851619081,36.0212916577943,37.112164408979));
#26336=CARTESIAN_POINT('Ctrl Pts',(-38.3119409591326,36.0252934543084,37.1842202372016));
#26337=CARTESIAN_POINT('Ctrl Pts',(-38.3730174631004,36.0319710262034,37.2561780174135));
#26338=CARTESIAN_POINT('Ctrl Pts',(-38.4340939670681,36.0386485980984,37.3281357976253));
#26339=CARTESIAN_POINT('Ctrl Pts',(-38.4949911568403,36.0480019430191,37.399995505153));
#26340=CARTESIAN_POINT('Ctrl Pts',(-38.5556112636636,36.0600158880042,37.471641760667));
#26341=CARTESIAN_POINT('Ctrl Pts',(-38.6162313704868,36.0720298329893,37.5432880161809));
#26342=CARTESIAN_POINT('Ctrl Pts',(-38.6765743735804,36.0867043738602,37.6147207951165));
#26343=CARTESIAN_POINT('Ctrl Pts',(-38.73654339765,36.1040158089172,37.6858254084132));
#26344=CARTESIAN_POINT('Ctrl Pts',(-38.7965124217196,36.1213272439742,37.75693002171));
#26345=CARTESIAN_POINT('Ctrl Pts',(-38.856107446209,36.1412755672286,37.8277064449908));
#26346=CARTESIAN_POINT('Ctrl Pts',(-38.9152327993705,36.1638286245175,37.8980410466006));
#26347=CARTESIAN_POINT('Ctrl Pts',(-38.974358152532,36.1863816818065,37.9683756482105));
#26348=CARTESIAN_POINT('Ctrl Pts',(-39.0330138140995,36.2115394653499,38.0382684040376));
#26349=CARTESIAN_POINT('Ctrl Pts',(-39.0911056220996,36.2392614718121,38.1076071035742));
#26350=CARTESIAN_POINT('Ctrl Pts',(-39.1491974300997,36.2669834782743,38.1769458031107));
#26351=CARTESIAN_POINT('Ctrl Pts',(-39.2067253646211,36.297269698109,38.245730422587));
#26352=CARTESIAN_POINT('Ctrl Pts',(-39.2635970748546,36.3300714087814,38.3138505318281));
#26353=CARTESIAN_POINT('Ctrl Pts',(-39.320468785088,36.3628731194539,38.3819706410691));
#26354=CARTESIAN_POINT('Ctrl Pts',(-39.3766842515407,36.3981903096824,38.449426216723));
#26355=CARTESIAN_POINT('Ctrl Pts',(-39.4321532301582,36.4359661939766,38.5161089624306));
#26356=CARTESIAN_POINT('Ctrl Pts',(-39.4876222087758,36.4737420782708,38.5827917081382));
#26357=CARTESIAN_POINT('Ctrl Pts',(-39.5423446805459,36.5139766436494,38.6487016010402));
#26358=CARTESIAN_POINT('Ctrl Pts',(-39.5962327970173,36.5566052236789,38.7137328252454));
#26359=CARTESIAN_POINT('Ctrl Pts',(-39.6501209134886,36.5992338037085,38.7787640494506));
#26360=CARTESIAN_POINT('Ctrl Pts',(-39.7031746561902,36.6442563837493,38.8429165826654));
#26361=CARTESIAN_POINT('Ctrl Pts',(-39.7553088534572,36.6916006236253,38.9060874281821));
#26362=CARTESIAN_POINT('Ctrl Pts',(-39.8074430507241,36.7389448635013,38.9692582736989));
#26363=CARTESIAN_POINT('Ctrl Pts',(-39.8586576846856,36.7886107469615,39.0314474098607));
#26364=CARTESIAN_POINT('Ctrl Pts',(-39.9088705330851,36.8405184918122,39.0925549888413));
#26365=CARTESIAN_POINT('Ctrl Pts',(-39.9590833814847,36.8924262366629,39.153662567822));
#26366=CARTESIAN_POINT('Ctrl Pts',(-40.0082944271086,36.946575825094,39.2136885686702));
#26367=CARTESIAN_POINT('Ctrl Pts',(-40.0564246602987,37.0028802884064,39.2725366120686));
#26368=CARTESIAN_POINT('Ctrl Pts',(-40.1045548934888,37.0591847517187,39.3313846554671));
#26369=CARTESIAN_POINT('Ctrl Pts',(-40.1516042977434,37.1176440705994,39.3890547212372));
#26370=CARTESIAN_POINT('Ctrl Pts',(-40.1974973289207,37.1781643683257,39.4454542071075));
#26371=CARTESIAN_POINT('Ctrl Pts',(-37.2861893607158,36.1599896970836,36.1561835957183));
#26372=CARTESIAN_POINT('Ctrl Pts',(-37.3481189647613,36.1368261638688,36.2278671181891));
#26373=CARTESIAN_POINT('Ctrl Pts',(-37.4104295575346,36.116431223471,36.3001131071893));
#26374=CARTESIAN_POINT('Ctrl Pts',(-37.4730148236326,36.0988394102363,36.3727982828643));
#26375=CARTESIAN_POINT('Ctrl Pts',(-37.5355445169199,36.081263217715,36.4454189174777));
#26376=CARTESIAN_POINT('Ctrl Pts',(-37.598348371835,36.066485183133,36.5184779311402));
#26377=CARTESIAN_POINT('Ctrl Pts',(-37.6613194336917,36.0545302334178,36.5918508930387));
#26378=CARTESIAN_POINT('Ctrl Pts',(-37.7242904955485,36.0425752837025,36.6652238549373));
#26379=CARTESIAN_POINT('Ctrl Pts',(-37.7874287400627,36.0334434233531,36.7389107367709));
#26380=CARTESIAN_POINT('Ctrl Pts',(-37.8506266534105,36.0271499800832,36.8127860511375));
#26381=CARTESIAN_POINT('Ctrl Pts',(-37.9138245667584,36.0208565368133,36.886661365504));
#26382=CARTESIAN_POINT('Ctrl Pts',(-37.9770821245729,36.0174015129466,36.9607250839144));
#26383=CARTESIAN_POINT('Ctrl Pts',(-38.0402916188546,36.0167905858017,37.0348510883942));
#26384=CARTESIAN_POINT('Ctrl Pts',(-38.1035011131364,36.0161796586568,37.1089770928739));
#26385=CARTESIAN_POINT('Ctrl Pts',(-38.166662519518,36.0184128283742,37.1831653548423));
#26386=CARTESIAN_POINT('Ctrl Pts',(-38.2296683014119,36.0234861033926,37.2572895538674));
#26387=CARTESIAN_POINT('Ctrl Pts',(-38.2926740833058,36.028559378411,37.3314137528924));
#26388=CARTESIAN_POINT('Ctrl Pts',(-38.3555242164265,36.0364727566876,37.4054738603985));
#26389=CARTESIAN_POINT('Ctrl Pts',(-38.4181117005737,36.0472125920524,37.4793437822614));
#26390=CARTESIAN_POINT('Ctrl Pts',(-38.480699184721,36.0579524274172,37.5532137041244));
#26391=CARTESIAN_POINT('Ctrl Pts',(-38.5430239957735,36.0715187156511,37.62689341187));
#26392=CARTESIAN_POINT('Ctrl Pts',(-38.6049800330493,36.087888202952,37.7002574656486));
#26393=CARTESIAN_POINT('Ctrl Pts',(-38.6669360703251,36.1042576902527,37.7736215194272));
#26394=CARTESIAN_POINT('Ctrl Pts',(-38.7285233099485,36.1234303702393,37.8466698909623));
#26395=CARTESIAN_POINT('Ctrl Pts',(-38.7896369108142,36.1453734609973,37.9192782203987));
#26396=CARTESIAN_POINT('Ctrl Pts',(-38.8507505116798,36.1673165517552,37.9918865498351));
#26397=CARTESIAN_POINT('Ctrl Pts',(-38.9113904502382,36.1920300447632,38.06405480919));
#26398=CARTESIAN_POINT('Ctrl Pts',(-38.9714535007296,36.2194717417869,38.1356601406378));
#26399=CARTESIAN_POINT('Ctrl Pts',(-39.0315165512211,36.2469134388106,38.2072654720858));
#26400=CARTESIAN_POINT('Ctrl Pts',(-39.0910026905017,36.2770833292175,38.2783078480319));
#26401=CARTESIAN_POINT('Ctrl Pts',(-39.1498106584341,36.3099299421387,38.3486663296049));
#26402=CARTESIAN_POINT('Ctrl Pts',(-39.2086186263666,36.3427765550599,38.4190248111778));
#26403=CARTESIAN_POINT('Ctrl Pts',(-39.2667484002909,36.3782998777878,38.488699371264));
#26404=CARTESIAN_POINT('Ctrl Pts',(-39.3241010292931,36.4164393419089,38.5575714003491));
#26405=CARTESIAN_POINT('Ctrl Pts',(-39.3814536582952,36.45457880603,38.6264434294343));
#26406=CARTESIAN_POINT('Ctrl Pts',(-39.438029120276,36.4953343968044,38.6945129009776));
#26407=CARTESIAN_POINT('Ctrl Pts',(-39.4937311093081,36.5386366541766,38.7616639373173));
#26408=CARTESIAN_POINT('Ctrl Pts',(-39.5494330983402,36.5819389115487,38.8288149736569));
#26409=CARTESIAN_POINT('Ctrl Pts',(-39.6042615929597,36.6277878187964,38.8950475489147));
#26410=CARTESIAN_POINT('Ctrl Pts',(-39.6581232590185,36.6761052602375,38.9602489105081));
#26411=CARTESIAN_POINT('Ctrl Pts',(-39.7119849250771,36.7244227016787,39.0254502721014));
#26412=CARTESIAN_POINT('Ctrl Pts',(-39.7648797418191,36.7752086586655,39.0896203949022));
#26413=CARTESIAN_POINT('Ctrl Pts',(-39.8167176635902,36.8283766252215,39.1526500340368));
#26414=CARTESIAN_POINT('Ctrl Pts',(-39.8685555853612,36.8815445917776,39.2156796731713));
#26415=CARTESIAN_POINT('Ctrl Pts',(-39.9193365921837,36.9370945473924,39.2775688043466));
#26416=CARTESIAN_POINT('Ctrl Pts',(-39.9689742324666,36.9949318895442,39.3382120611364));
#26417=CARTESIAN_POINT('Ctrl Pts',(-40.0186118727495,37.0527692316959,39.3988553179263));
#26418=CARTESIAN_POINT('Ctrl Pts',(-40.0671061273606,37.1128939380812,39.4582526769549));
#26419=CARTESIAN_POINT('Ctrl Pts',(-40.1143744321613,37.1752036308061,39.5163030078388));
#26420=CARTESIAN_POINT('Ctrl Pts',(-37.1201105829165,36.1914413355051,36.1322276221139));
#26421=CARTESIAN_POINT('Ctrl Pts',(-37.1833706680423,36.1650364607197,36.2053221084819));
#26422=CARTESIAN_POINT('Ctrl Pts',(-37.2470865241116,36.1415374300666,36.2790718308968));
#26423=CARTESIAN_POINT('Ctrl Pts',(-37.3111430442604,36.1209866911517,36.3533435554538));
#26424=CARTESIAN_POINT('Ctrl Pts',(-37.3751426851931,36.1004542003389,36.4275493301675));
#26425=CARTESIAN_POINT('Ctrl Pts',(-37.4394823577102,36.0828647766077,36.5022761482019));
#26426=CARTESIAN_POINT('Ctrl Pts',(-37.5040460348623,36.0682501398455,36.5773892509488));
#26427=CARTESIAN_POINT('Ctrl Pts',(-37.5686097120143,36.0536355030834,36.6525023536957));
#26428=CARTESIAN_POINT('Ctrl Pts',(-37.6333973657805,36.0419956596332,36.7280017085557));
#26429=CARTESIAN_POINT('Ctrl Pts',(-37.6982921613446,36.0333516002066,36.8037511637661));
#26430=CARTESIAN_POINT('Ctrl Pts',(-37.7631869569087,36.0247075407801,36.8795006189766));
#26431=CARTESIAN_POINT('Ctrl Pts',(-37.828188866106,36.0190592691289,36.9555001416619));
#26432=CARTESIAN_POINT('Ctrl Pts',(-37.8931806677428,36.0164169710636,37.031612678082));
#26433=CARTESIAN_POINT('Ctrl Pts',(-37.9581724693795,36.0137746729984,37.1077252145021));
#26434=CARTESIAN_POINT('Ctrl Pts',(-38.023154135249,36.014138349666,37.1839507316237));
#26435=CARTESIAN_POINT('Ctrl Pts',(-38.0880084806633,36.0175073452301,37.2601517681595));
#26436=CARTESIAN_POINT('Ctrl Pts',(-38.1528628260775,36.0208763407942,37.3363528046953));
#26437=CARTESIAN_POINT('Ctrl Pts',(-38.2175898228894,36.0272506537927,37.4125293275738));
#26438=CARTESIAN_POINT('Ctrl Pts',(-38.2820727456685,36.036618789108,37.4885439638614));
#26439=CARTESIAN_POINT('Ctrl Pts',(-38.3465556684475,36.0459869244234,37.564558600149));
#26440=CARTESIAN_POINT('Ctrl Pts',(-38.4107944892078,36.0583488779898,37.6404113168551));
#26441=CARTESIAN_POINT('Ctrl Pts',(-38.4746733628712,36.0736823568782,37.7159653249819));
#26442=CARTESIAN_POINT('Ctrl Pts',(-38.5385522365345,36.0890158357666,37.7915193331088));
#26443=CARTESIAN_POINT('Ctrl Pts',(-38.6020711353772,36.1073208333222,37.8667745998657));
#26444=CARTESIAN_POINT('Ctrl Pts',(-38.6651155125921,36.1285643392274,37.9415954136664));
#26445=CARTESIAN_POINT('Ctrl Pts',(-38.728159889807,36.1498078451326,38.016416227467));
#26446=CARTESIAN_POINT('Ctrl Pts',(-38.7907297180327,36.1739898501675,38.0908025558389));
#26447=CARTESIAN_POINT('Ctrl Pts',(-38.8527121619685,36.2010667457132,38.1646202541957));
#26448=CARTESIAN_POINT('Ctrl Pts',(-38.9146946059044,36.228143641259,38.2384379525525));
#26449=CARTESIAN_POINT('Ctrl Pts',(-38.9760896386497,36.2581154155639,38.3116869888571));
#26450=CARTESIAN_POINT('Ctrl Pts',(-39.0367865434716,36.2909280190285,38.384235269459));
#26451=CARTESIAN_POINT('Ctrl Pts',(-39.0974834482934,36.3237406224932,38.4567835500607));
#26452=CARTESIAN_POINT('Ctrl Pts',(-39.157482198849,36.3593940408766,38.5286310434735));
#26453=CARTESIAN_POINT('Ctrl Pts',(-39.2166745963907,36.3978239785864,38.599648183519));
#26454=CARTESIAN_POINT('Ctrl Pts',(-39.2758669939324,36.4362539162962,38.6706653235644));
#26455=CARTESIAN_POINT('Ctrl Pts',(-39.3342530127704,36.4774603566536,38.7408520794209));
#26456=CARTESIAN_POINT('Ctrl Pts',(-39.3917273624771,36.5213689900238,38.8100818798013));
#26457=CARTESIAN_POINT('Ctrl Pts',(-39.4492017121837,36.5652776233941,38.8793116801817));
#26458=CARTESIAN_POINT('Ctrl Pts',(-39.5057643678147,36.6118884307206,38.9475844950401));
#26459=CARTESIAN_POINT('Ctrl Pts',(-39.5613133271045,36.6611173564033,39.0147772045947));
#26460=CARTESIAN_POINT('Ctrl Pts',(-39.6168622863942,36.7103462820862,39.0819699141494));
#26461=CARTESIAN_POINT('Ctrl Pts',(-39.6713975252342,36.7621933047597,39.1480824892385));
#26462=CARTESIAN_POINT('Ctrl Pts',(-39.7248206975006,36.816564926095,39.2129957057488));
#26463=CARTESIAN_POINT('Ctrl Pts',(-39.7782438697671,36.8709365474302,39.2779089222591));
#26464=CARTESIAN_POINT('Ctrl Pts',(-39.8305549522741,36.9278327438297,39.3416227520181));
#26465=CARTESIAN_POINT('Ctrl Pts',(-39.8816596098305,36.9871509115369,39.40402229669));
#26466=CARTESIAN_POINT('Ctrl Pts',(-39.9327642673869,37.0464690792441,39.466421841362));
#26467=CARTESIAN_POINT('Ctrl Pts',(-39.982662477813,37.1082091925145,39.5275070738652));
#26468=CARTESIAN_POINT('Ctrl Pts',(-40.0312642571703,37.1722599123143,39.5871678361448));
#26469=CARTESIAN_POINT('Ctrl Pts',(-36.9540318051171,36.2228929739267,36.1082716485095));
#26470=CARTESIAN_POINT('Ctrl Pts',(-37.0186223713234,36.1932467575705,36.1827770987747));
#26471=CARTESIAN_POINT('Ctrl Pts',(-37.0837434906885,36.1666436366623,36.2580305546043));
#26472=CARTESIAN_POINT('Ctrl Pts',(-37.1492712648881,36.1431339720672,36.3338888280434));
#26473=CARTESIAN_POINT('Ctrl Pts',(-37.2147408534664,36.1196451829629,36.4096797428573));
#26474=CARTESIAN_POINT('Ctrl Pts',(-37.2806163435853,36.0992443700824,36.4860743652637));
#26475=CARTESIAN_POINT('Ctrl Pts',(-37.3467726360328,36.0819700462733,36.5629276088589));
#26476=CARTESIAN_POINT('Ctrl Pts',(-37.4129289284802,36.0646957224643,36.6397808524541));
#26477=CARTESIAN_POINT('Ctrl Pts',(-37.4793659914983,36.0505478959133,36.7170926803403));
#26478=CARTESIAN_POINT('Ctrl Pts',(-37.5459576692786,36.0395532203301,36.7947162763948));
#26479=CARTESIAN_POINT('Ctrl Pts',(-37.612549347059,36.0285585447468,36.8723398724492));
#26480=CARTESIAN_POINT('Ctrl Pts',(-37.6792956076391,36.020717025311,36.9502751994095));
#26481=CARTESIAN_POINT('Ctrl Pts',(-37.7460697166309,36.0160433563256,37.0283742677699));
#26482=CARTESIAN_POINT('Ctrl Pts',(-37.8128438256227,36.01136968734,37.1064733361303));
#26483=CARTESIAN_POINT('Ctrl Pts',(-37.87964575098,36.0098638709579,37.184736108405));
#26484=CARTESIAN_POINT('Ctrl Pts',(-37.9463486599146,36.0115285870677,37.2630139824516));
#26485=CARTESIAN_POINT('Ctrl Pts',(-38.0130515688492,36.0131933031775,37.3412918564982));
#26486=CARTESIAN_POINT('Ctrl Pts',(-38.0796554293524,36.0180285508978,37.4195847947491));
#26487=CARTESIAN_POINT('Ctrl Pts',(-38.1460337907632,36.0260249861637,37.4977441454614));
#26488=CARTESIAN_POINT('Ctrl Pts',(-38.212412152174,36.0340214214295,37.5759034961736));
#26489=CARTESIAN_POINT('Ctrl Pts',(-38.2785649826422,36.0451790403285,37.6539292218401));
#26490=CARTESIAN_POINT('Ctrl Pts',(-38.3443666926931,36.0594765108045,37.7316731843153));
#26491=CARTESIAN_POINT('Ctrl Pts',(-38.4101684027439,36.0737739812805,37.8094171467904));
#26492=CARTESIAN_POINT('Ctrl Pts',(-38.4756189608059,36.091211296405,37.8868793087691));
#26493=CARTESIAN_POINT('Ctrl Pts',(-38.5405941143701,36.1117552174574,37.963912606934));
#26494=CARTESIAN_POINT('Ctrl Pts',(-38.6055692679342,36.1322991385099,38.0409459050989));
#26495=CARTESIAN_POINT('Ctrl Pts',(-38.6700689858271,36.1559496555719,38.1175503024878));
#26496=CARTESIAN_POINT('Ctrl Pts',(-38.7339708232074,36.1826617496396,38.1935803677536));
#26497=CARTESIAN_POINT('Ctrl Pts',(-38.7978726605876,36.2093738437074,38.2696104330193));
#26498=CARTESIAN_POINT('Ctrl Pts',(-38.8611765867978,36.2391475019103,38.3450661296824));
#26499=CARTESIAN_POINT('Ctrl Pts',(-38.923762428509,36.2719260959184,38.419804209313));
#26500=CARTESIAN_POINT('Ctrl Pts',(-38.9863482702203,36.3047046899263,38.4945422889437));
#26501=CARTESIAN_POINT('Ctrl Pts',(-39.048215997407,36.3404882039654,38.5685627156829));
#26502=CARTESIAN_POINT('Ctrl Pts',(-39.1092481634882,36.379208615264,38.6417249666887));
#26503=CARTESIAN_POINT('Ctrl Pts',(-39.1702803295695,36.4179290265625,38.7148872176946));
#26504=CARTESIAN_POINT('Ctrl Pts',(-39.2304769052649,36.4595863165027,38.7871912578642));
#26505=CARTESIAN_POINT('Ctrl Pts',(-39.289723615646,36.5041013258711,38.8584998222854));
#26506=CARTESIAN_POINT('Ctrl Pts',(-39.3489703260272,36.5486163352394,38.9298083867066));
#26507=CARTESIAN_POINT('Ctrl Pts',(-39.4072671426698,36.5959890426447,39.0001214411655));
#26508=CARTESIAN_POINT('Ctrl Pts',(-39.4645033951906,36.6461294525692,39.0693054986814));
#26509=CARTESIAN_POINT('Ctrl Pts',(-39.5217396477114,36.6962698624937,39.1384895561974));
#26510=CARTESIAN_POINT('Ctrl Pts',(-39.5779153086493,36.7491779508538,39.2065445835747));
#26511=CARTESIAN_POINT('Ctrl Pts',(-39.6329237314111,36.8047532269684,39.2733413774608));
#26512=CARTESIAN_POINT('Ctrl Pts',(-39.6879321541729,36.8603285030829,39.3401381713469));
#26513=CARTESIAN_POINT('Ctrl Pts',(-39.7417733123646,36.918570940267,39.4056766996897));
#26514=CARTESIAN_POINT('Ctrl Pts',(-39.7943449871944,36.9793699335296,39.4698325322437));
#26515=CARTESIAN_POINT('Ctrl Pts',(-39.8469166620243,37.0401689267921,39.5339883647977));
#26516=CARTESIAN_POINT('Ctrl Pts',(-39.8982188282653,37.1035244469479,39.5967614707754));
#26517=CARTESIAN_POINT('Ctrl Pts',(-39.9481540821793,37.1693161938226,39.6580326644507));
#26518=CARTESIAN_POINT('Ctrl Pts',(-36.7912613073679,36.2583245548778,36.0878978700413));
#26519=CARTESIAN_POINT('Ctrl Pts',(-36.8570448313337,36.2253491798246,36.1636570993428));
#26520=CARTESIAN_POINT('Ctrl Pts',(-36.9234401661104,36.1955503975034,36.2402647180933));
#26521=CARTESIAN_POINT('Ctrl Pts',(-36.9903143661334,36.1689875916672,36.3175673204643));
#26522=CARTESIAN_POINT('Ctrl Pts',(-37.0571291849714,36.1424483723694,36.394801281713));
#26523=CARTESIAN_POINT('Ctrl Pts',(-37.1244219834839,36.1191393992778,36.472728951828));
#26524=CARTESIAN_POINT('Ctrl Pts',(-37.1920582731525,36.0991070017637,36.5511945771713));
#26525=CARTESIAN_POINT('Ctrl Pts',(-37.259694562821,36.0790746042497,36.6296602025146));
#26526=CARTESIAN_POINT('Ctrl Pts',(-37.327674307687,36.062318792826,36.7086637413645));
#26527=CARTESIAN_POINT('Ctrl Pts',(-37.3958616587387,36.0488728169132,36.7880473051252));
#26528=CARTESIAN_POINT('Ctrl Pts',(-37.4640490097905,36.0354268410005,36.8674308688859));
#26529=CARTESIAN_POINT('Ctrl Pts',(-37.5324439307829,36.0252907076194,36.9471944153556));
#26530=CARTESIAN_POINT('Ctrl Pts',(-37.6009097538766,36.0184844547042,37.0271785505671));
#26531=CARTESIAN_POINT('Ctrl Pts',(-37.6693755769703,36.0116782017889,37.1071626857786));
#26532=CARTESIAN_POINT('Ctrl Pts',(-37.7379122657777,36.0082018328405,37.1873673672181));
#26533=CARTESIAN_POINT('Ctrl Pts',(-37.8063828785137,36.0080620953735,37.2676323310766));
#26534=CARTESIAN_POINT('Ctrl Pts',(-37.8748534912497,36.0079223579063,37.3478972949351));
#26535=CARTESIAN_POINT('Ctrl Pts',(-37.9432579915291,36.0111192518882,37.4282224985554));
#26536=CARTESIAN_POINT('Ctrl Pts',(-38.0114597095541,36.0176462083918,37.5084474472333));
#26537=CARTESIAN_POINT('Ctrl Pts',(-38.079661427579,36.0241731648953,37.5886723959111));
#26538=CARTESIAN_POINT('Ctrl Pts',(-38.1476603271114,36.0340301803553,37.6687970470156));
#26539=CARTESIAN_POINT('Ctrl Pts',(-38.2153205551546,36.0471973963919,37.7486613147697));
#26540=CARTESIAN_POINT('Ctrl Pts',(-38.2829807831979,36.0603646124286,37.8285255825238));
#26541=CARTESIAN_POINT('Ctrl Pts',(-38.3503023038048,36.0768420219581,37.9081294244924));
#26542=CARTESIAN_POINT('Ctrl Pts',(-38.4171506223099,36.0965965570376,37.9873138019821));
#26543=CARTESIAN_POINT('Ctrl Pts',(-38.483998940815,36.1163510921171,38.0664981794718));
#26544=CARTESIAN_POINT('Ctrl Pts',(-38.5503740217048,36.1393827421724,38.1452630504119));
#26545=CARTESIAN_POINT('Ctrl Pts',(-38.6161432647377,36.1656453621667,38.223451057146));
#26546=CARTESIAN_POINT('Ctrl Pts',(-38.6819125077707,36.1919079821609,38.3016390638801));
#26547=CARTESIAN_POINT('Ctrl Pts',(-38.7470758780082,36.2214015580719,38.3792501648692));
#26548=CARTESIAN_POINT('Ctrl Pts',(-38.8115031981583,36.2540670522875,38.4561293107248));
#26549=CARTESIAN_POINT('Ctrl Pts',(-38.8759305183084,36.286732546503,38.5330084565804));
#26550=CARTESIAN_POINT('Ctrl Pts',(-38.9396217541463,36.3225699416089,38.6091556064603));
#26551=CARTESIAN_POINT('Ctrl Pts',(-39.0024496701877,36.361507543251,38.6844186372596));
#26552=CARTESIAN_POINT('Ctrl Pts',(-39.0652775862291,36.400445144893,38.759681668059));
#26553=CARTESIAN_POINT('Ctrl Pts',(-39.1272421490989,36.4424829323341,38.8340605397946));
#26554=CARTESIAN_POINT('Ctrl Pts',(-39.1882195722495,36.4875368406862,38.9074066619901));
#26555=CARTESIAN_POINT('Ctrl Pts',(-39.2491969954,36.5325907490382,38.9807527841855));
#26556=CARTESIAN_POINT('Ctrl Pts',(-39.3091872464385,36.5806607543238,39.0530661178757));
#26557=CARTESIAN_POINT('Ctrl Pts',(-39.3680704811376,36.6316507565641,39.1242021974759));
#26558=CARTESIAN_POINT('Ctrl Pts',(-39.4269537158367,36.6826407588044,39.1953382770762));
#26559=CARTESIAN_POINT('Ctrl Pts',(-39.4847299029149,36.736550730877,39.2652970647943));
#26560=CARTESIAN_POINT('Ctrl Pts',(-39.5412836181438,36.7932729210564,39.3339387957669));
#26561=CARTESIAN_POINT('Ctrl Pts',(-39.5978373333727,36.8499951112357,39.4025805267396));
#26562=CARTESIAN_POINT('Ctrl Pts',(-39.6531685467061,36.9095294893625,39.4699051644974));
#26563=CARTESIAN_POINT('Ctrl Pts',(-39.7071667139898,36.9717570816839,39.5357782020048));
#26564=CARTESIAN_POINT('Ctrl Pts',(-39.7611648812735,37.0339846740053,39.6016512395122));
#26565=CARTESIAN_POINT('Ctrl Pts',(-39.8138299738162,37.098905447445,39.6660726417677));
#26566=CARTESIAN_POINT('Ctrl Pts',(-39.8650567681803,37.1663896806103,39.7289136957327));
#26567=CARTESIAN_POINT('Ctrl Pts',(-36.6313596335673,36.2971547767807,36.0705950037057));
#26568=CARTESIAN_POINT('Ctrl Pts',(-36.6982091283211,36.260779871097,36.1474619304646));
#26569=CARTESIAN_POINT('Ctrl Pts',(-36.7657578569626,36.2277105354781,36.2252849626787));
#26570=CARTESIAN_POINT('Ctrl Pts',(-36.8338636442589,36.1980163667922,36.3039002996823));
#26571=CARTESIAN_POINT('Ctrl Pts',(-36.9019089567779,36.1683485651496,36.3824458299163));
#26572=CARTESIAN_POINT('Ctrl Pts',(-36.9705102990142,36.1420499565984,36.4617822122257));
#26573=CARTESIAN_POINT('Ctrl Pts',(-37.0395235375808,36.1191757952692,36.5417427585964));
#26574=CARTESIAN_POINT('Ctrl Pts',(-37.1085367761474,36.09630163394,36.6217033049671));
#26575=CARTESIAN_POINT('Ctrl Pts',(-37.1779618703816,36.0768519333104,36.7022879682863));
#26576=CARTESIAN_POINT('Ctrl Pts',(-37.2476529561698,36.0608675577589,36.7833274378659));
#26577=CARTESIAN_POINT('Ctrl Pts',(-37.3173440419582,36.0448831822074,36.8643669074455));
#26578=CARTESIAN_POINT('Ctrl Pts',(-37.3873010782385,36.0323641411522,36.9458611355369));
#26579=CARTESIAN_POINT('Ctrl Pts',(-37.4573770832718,36.0233367374574,37.0276389004303));
#26580=CARTESIAN_POINT('Ctrl Pts',(-37.5274530883051,36.0143093337625,37.1094166653237));
#26581=CARTESIAN_POINT('Ctrl Pts',(-37.5976480208025,36.008773572747,37.1914779188356));
#26582=CARTESIAN_POINT('Ctrl Pts',(-37.6678143991983,36.0067410852035,37.2736502479195));
#26583=CARTESIAN_POINT('Ctrl Pts',(-37.7379807775941,36.00470859766,37.3558225770034));
#26584=CARTESIAN_POINT('Ctrl Pts',(-37.8081185605461,36.0061793847861,37.4381059332432));
#26585=CARTESIAN_POINT('Ctrl Pts',(-37.8780803865613,36.0111503564157,37.5203274369483));
#26586=CARTESIAN_POINT('Ctrl Pts',(-37.9480422125766,36.0161213280453,37.6025489406534));
#26587=CARTESIAN_POINT('Ctrl Pts',(-38.0178280404336,36.0245924812496,37.6847085433788));
#26588=CARTESIAN_POINT('Ctrl Pts',(-38.087291248107,36.0365460178929,37.7666336254434));
#26589=CARTESIAN_POINT('Ctrl Pts',(-38.1567544557805,36.0484995545361,37.8485587075081));
#26590=CARTESIAN_POINT('Ctrl Pts',(-38.2258950023425,36.0639354675753,37.9302492206416));
#26591=CARTESIAN_POINT('Ctrl Pts',(-38.2945676215226,36.0828213257145,38.0115335307338));
#26592=CARTESIAN_POINT('Ctrl Pts',(-38.3632402407026,36.1017071838536,38.092817840826));
#26593=CARTESIAN_POINT('Ctrl Pts',(-38.4314448920386,36.1240429759653,38.173695899984));
#26594=CARTESIAN_POINT('Ctrl Pts',(-38.4990382756025,36.1497817739097,38.2539977810866));
#26595=CARTESIAN_POINT('Ctrl Pts',(-38.5666316591664,36.1755205718542,38.3342996621892));
#26596=CARTESIAN_POINT('Ctrl Pts',(-38.6336137351323,36.2046623604661,38.4140253179224));
#26597=CARTESIAN_POINT('Ctrl Pts',(-38.6998437722378,36.2371459120121,38.4930072423977));
#26598=CARTESIAN_POINT('Ctrl Pts',(-38.7660738093433,36.2696294635582,38.571989166873));
#26599=CARTESIAN_POINT('Ctrl Pts',(-38.8315517685658,36.3054547588989,38.6502273135541));
#26600=CARTESIAN_POINT('Ctrl Pts',(-38.8961400788355,36.3445465280617,38.7275573018515));
#26601=CARTESIAN_POINT('Ctrl Pts',(-38.9607283891053,36.3836382972244,38.8048872901491));
#26602=CARTESIAN_POINT('Ctrl Pts',(-39.0244270123667,36.4259965171763,38.8813090745));
#26603=CARTESIAN_POINT('Ctrl Pts',(-39.087102115986,36.4715321920828,38.9566620905444));
#26604=CARTESIAN_POINT('Ctrl Pts',(-39.1497772196053,36.5170678669892,39.0320151065888));
#26605=CARTESIAN_POINT('Ctrl Pts',(-39.2114287666543,36.5657809700204,39.1062993099285));
#26606=CARTESIAN_POINT('Ctrl Pts',(-39.2719272254649,36.6175691535503,39.1793586273225));
#26607=CARTESIAN_POINT('Ctrl Pts',(-39.3324256842755,36.6693573370803,39.2524179447164));
#26608=CARTESIAN_POINT('Ctrl Pts',(-39.3917710192021,36.7242205705952,39.324252333118));
#26609=CARTESIAN_POINT('Ctrl Pts',(-39.4498385439942,36.7820435848685,39.3947108664176));
#26610=CARTESIAN_POINT('Ctrl Pts',(-39.5079060687864,36.8398665991418,39.4651693997171));
#26611=CARTESIAN_POINT('Ctrl Pts',(-39.5646957492308,36.9006493601041,39.5342520364003));
#26612=CARTESIAN_POINT('Ctrl Pts',(-39.6200882685805,36.9642641614319,39.6018136318669));
#26613=CARTESIAN_POINT('Ctrl Pts',(-39.6754807879302,37.0278789627596,39.6693752273335));
#26614=CARTESIAN_POINT('Ctrl Pts',(-39.7294761135479,37.0943257669709,39.7354157417759));
#26615=CARTESIAN_POINT('Ctrl Pts',(-39.7819607997063,37.1634649674249,39.79979642218));
#26616=CARTESIAN_POINT('Ctrl Pts',(-36.4714579597666,36.3359849986837,36.0532921373701));
#26617=CARTESIAN_POINT('Ctrl Pts',(-36.5393734253084,36.2962105623695,36.1312667615863));
#26618=CARTESIAN_POINT('Ctrl Pts',(-36.6080755478147,36.2598706734529,36.2103052072641));
#26619=CARTESIAN_POINT('Ctrl Pts',(-36.6774129223844,36.2270451419173,36.2902332789004));
#26620=CARTESIAN_POINT('Ctrl Pts',(-36.7466887285845,36.1942487579297,36.3700903781196));
#26621=CARTESIAN_POINT('Ctrl Pts',(-36.8165986145445,36.1649605139189,36.4508354726234));
#26622=CARTESIAN_POINT('Ctrl Pts',(-36.8869888020091,36.1392445887747,36.5322909400215));
#26623=CARTESIAN_POINT('Ctrl Pts',(-36.9573789894737,36.1135286636304,36.6137464074195));
#26624=CARTESIAN_POINT('Ctrl Pts',(-37.0282494330761,36.0913850737948,36.6959121952081));
#26625=CARTESIAN_POINT('Ctrl Pts',(-37.099444253601,36.0728622986046,36.7786075706066));
#26626=CARTESIAN_POINT('Ctrl Pts',(-37.1706390741258,36.0543395234144,36.8613029460051));
#26627=CARTESIAN_POINT('Ctrl Pts',(-37.242158225694,36.0394375746849,36.9445278557182));
#26628=CARTESIAN_POINT('Ctrl Pts',(-37.3138444126669,36.0281890202105,37.0280992502935));
#26629=CARTESIAN_POINT('Ctrl Pts',(-37.3855305996398,36.0169404657361,37.1116706448688));
#26630=CARTESIAN_POINT('Ctrl Pts',(-37.4573837758273,36.0093453126535,37.1955884704532));
#26631=CARTESIAN_POINT('Ctrl Pts',(-37.5292459198829,36.0054200750336,37.2796681647624));
#26632=CARTESIAN_POINT('Ctrl Pts',(-37.6011080639385,36.0014948374137,37.3637478590717));
#26633=CARTESIAN_POINT('Ctrl Pts',(-37.6729791295631,36.001239517684,37.4479893679309));
#26634=CARTESIAN_POINT('Ctrl Pts',(-37.7447010635687,36.0046545044396,37.5322074266633));
#26635=CARTESIAN_POINT('Ctrl Pts',(-37.8164229975742,36.0080694911953,37.6164254853956));
#26636=CARTESIAN_POINT('Ctrl Pts',(-37.8879957537558,36.015154782144,37.7006200397419));
#26637=CARTESIAN_POINT('Ctrl Pts',(-37.9592619410594,36.0258946393938,37.7846059361171));
#26638=CARTESIAN_POINT('Ctrl Pts',(-38.030528128363,36.0366344966437,37.8685918324923));
#26639=CARTESIAN_POINT('Ctrl Pts',(-38.1014877008803,36.0510289131925,37.9523690167908));
#26640=CARTESIAN_POINT('Ctrl Pts',(-38.1719846207352,36.0690460943914,38.0357532594855));
#26641=CARTESIAN_POINT('Ctrl Pts',(-38.2424815405902,36.0870632755903,38.1191375021802));
#26642=CARTESIAN_POINT('Ctrl Pts',(-38.3125157623724,36.1087032097581,38.2021287495561));
#26643=CARTESIAN_POINT('Ctrl Pts',(-38.3819332864673,36.1339181856529,38.2845445050272));
#26644=CARTESIAN_POINT('Ctrl Pts',(-38.4513508105622,36.1591331615475,38.3669602604983));
#26645=CARTESIAN_POINT('Ctrl Pts',(-38.5201515922563,36.1879231628604,38.4488004709756));
#26646=CARTESIAN_POINT('Ctrl Pts',(-38.5881843463173,36.2202247717368,38.5298851740706));
#26647=CARTESIAN_POINT('Ctrl Pts',(-38.6562171003783,36.2525263806133,38.6109698771655));
#26648=CARTESIAN_POINT('Ctrl Pts',(-38.7234817829854,36.2883395761889,38.6912990206478));
#26649=CARTESIAN_POINT('Ctrl Pts',(-38.7898304874834,36.3275855128724,38.7706959664435));
#26650=CARTESIAN_POINT('Ctrl Pts',(-38.8561791919814,36.3668314495559,38.8500929122391));
#26651=CARTESIAN_POINT('Ctrl Pts',(-38.9216118756344,36.4095101020185,38.9285576092055));
#26652=CARTESIAN_POINT('Ctrl Pts',(-38.9859846597225,36.4555275434794,39.0059175190987));
#26653=CARTESIAN_POINT('Ctrl Pts',(-39.0503574438107,36.5015449849401,39.083277428992));
#26654=CARTESIAN_POINT('Ctrl Pts',(-39.1136702868701,36.550901185717,39.1595325019814));
#26655=CARTESIAN_POINT('Ctrl Pts',(-39.1757839697923,36.6034875505365,39.234515057169));
#26656=CARTESIAN_POINT('Ctrl Pts',(-39.2378976527144,36.6560739153561,39.3094976123567));
#26657=CARTESIAN_POINT('Ctrl Pts',(-39.2988121354892,36.7118904103133,39.3832076014418));
#26658=CARTESIAN_POINT('Ctrl Pts',(-39.3583934698447,36.7708142486806,39.4554829370682));
#26659=CARTESIAN_POINT('Ctrl Pts',(-39.4179748042001,36.829738087048,39.5277582726946));
#26660=CARTESIAN_POINT('Ctrl Pts',(-39.4762229517554,36.8917692308458,39.5985989083033));
#26661=CARTESIAN_POINT('Ctrl Pts',(-39.5330098231711,36.9567712411799,39.6678490617289));
#26662=CARTESIAN_POINT('Ctrl Pts',(-39.5897966945868,37.021773251514,39.7370992151546));
#26663=CARTESIAN_POINT('Ctrl Pts',(-39.6451222532796,37.0897460864968,39.8047588417841));
#26664=CARTESIAN_POINT('Ctrl Pts',(-39.6988648312323,37.1605402542396,39.8706791486274));
#26665=CARTESIAN_POINT('Ctrl Pts',(-36.3144288446909,36.3782187397976,36.0390644866415));
#26666=CARTESIAN_POINT('Ctrl Pts',(-36.3832832065462,36.3349742844667,36.1180006296823));
#26667=CARTESIAN_POINT('Ctrl Pts',(-36.4530178150635,36.2952888355839,36.1981156434926));
#26668=CARTESIAN_POINT('Ctrl Pts',(-36.523471853133,36.2592536063736,36.2792247606169));
#26669=CARTESIAN_POINT('Ctrl Pts',(-36.5938633312875,36.2232503747738,36.3602618566107));
#26670=CARTESIAN_POINT('Ctrl Pts',(-36.6649729122354,36.1908909085033,36.4422912340599));
#26671=CARTESIAN_POINT('Ctrl Pts',(-36.7366369171835,36.1622494193356,36.5251240689158));
#26672=CARTESIAN_POINT('Ctrl Pts',(-36.8083009221317,36.1336079301679,36.6079569037717));
#26673=CARTESIAN_POINT('Ctrl Pts',(-36.8805193005059,36.108684438148,36.6915931375718));
#26674=CARTESIAN_POINT('Ctrl Pts',(-36.9531258359889,36.0875360567009,36.7758402656948));
#26675=CARTESIAN_POINT('Ctrl Pts',(-37.025732371472,36.0663876752538,36.8600873938177));
#26676=CARTESIAN_POINT('Ctrl Pts',(-37.0987270128334,36.0490144191481,36.9449453568138));
#26677=CARTESIAN_POINT('Ctrl Pts',(-37.171941769992,36.0354560422844,37.0302188540894));
#26678=CARTESIAN_POINT('Ctrl Pts',(-37.2451565271507,36.0218976654207,37.1154923513651));
#26679=CARTESIAN_POINT('Ctrl Pts',(-37.3185913484547,36.0121541772235,37.2011813227561));
#26680=CARTESIAN_POINT('Ctrl Pts',(-37.392077241905,36.0062477905694,37.2870885690652));
#26681=CARTESIAN_POINT('Ctrl Pts',(-37.4655631353554,36.0003414039153,37.3729958153742));
#26682=CARTESIAN_POINT('Ctrl Pts',(-37.5391000491155,35.998272122842,37.4591212759982));
#26683=CARTESIAN_POINT('Ctrl Pts',(-37.612518765662,36.0000445182044,37.5452667591572));
#26684=CARTESIAN_POINT('Ctrl Pts',(-37.6859374822086,36.0018169135668,37.6314122423163));
#26685=CARTESIAN_POINT('Ctrl Pts',(-37.7592379497577,36.0074309839979,37.7175776872464));
#26686=CARTESIAN_POINT('Ctrl Pts',(-37.8322515026438,36.0168736382935,37.8035648201072));
#26687=CARTESIAN_POINT('Ctrl Pts',(-37.9052650555298,36.0263162925892,37.8895519529678));
#26688=CARTESIAN_POINT('Ctrl Pts',(-37.9779916422593,36.0395875239842,37.9753607131126));
#26689=CARTESIAN_POINT('Ctrl Pts',(-38.0502639238318,36.0566566402252,38.0607936554889));
#26690=CARTESIAN_POINT('Ctrl Pts',(-38.1225362054044,36.0737257564662,38.1462265978652));
#26691=CARTESIAN_POINT('Ctrl Pts',(-38.1943541308527,36.0945927454211,38.2312836622219));
#26692=CARTESIAN_POINT('Ctrl Pts',(-38.2655524565242,36.1192094555603,38.3157691392955));
#26693=CARTESIAN_POINT('Ctrl Pts',(-38.3367507821957,36.1438261656996,38.4002546163691));
#26694=CARTESIAN_POINT('Ctrl Pts',(-38.4073294578828,36.1721925795798,38.4841684465799));
#26695=CARTESIAN_POINT('Ctrl Pts',(-38.4771260943151,36.2042433082775,38.5673175554497));
#26696=CARTESIAN_POINT('Ctrl Pts',(-38.5469227307473,36.2362940369752,38.6504666643194));
#26697=CARTESIAN_POINT('Ctrl Pts',(-38.615937278707,36.2720290578162,38.732850993213));
#26698=CARTESIAN_POINT('Ctrl Pts',(-38.6840109492129,36.3113660454538,38.8142809893088));
#26699=CARTESIAN_POINT('Ctrl Pts',(-38.7520846197189,36.3507030330916,38.8957109854046));
#26700=CARTESIAN_POINT('Ctrl Pts',(-38.819217364769,36.3936419597249,38.9761865912809));
#26701=CARTESIAN_POINT('Ctrl Pts',(-38.8852547250341,36.4400839422626,39.0555226464555));
#26702=CARTESIAN_POINT('Ctrl Pts',(-38.9512920852992,36.4865259248002,39.1348587016301));
#26703=CARTESIAN_POINT('Ctrl Pts',(-39.0162340142127,36.5364709304417,39.2130551501577));
#26704=CARTESIAN_POINT('Ctrl Pts',(-39.0799310915729,36.5898039729972,39.2899320743992));
#26705=CARTESIAN_POINT('Ctrl Pts',(-39.1436281689332,36.6431370155525,39.3668089986409));
#26706=CARTESIAN_POINT('Ctrl Pts',(-39.2060803498222,36.6998580573726,39.442366344384));
#26707=CARTESIAN_POINT('Ctrl Pts',(-39.2671439395029,36.7598365376979,39.5164302632599));
#26708=CARTESIAN_POINT('Ctrl Pts',(-39.3282075291836,36.8198150180233,39.5904941821358));
#26709=CARTESIAN_POINT('Ctrl Pts',(-39.3878824845926,36.8830508945285,39.6630646219134));
#26710=CARTESIAN_POINT('Ctrl Pts',(-39.4460314965102,36.9493986318733,39.7339746020575));
#26711=CARTESIAN_POINT('Ctrl Pts',(-39.5041805084277,37.0157463692181,39.8048845822015));
#26712=CARTESIAN_POINT('Ctrl Pts',(-39.5608035358426,37.0852059205947,39.8741340527016));
#26713=CARTESIAN_POINT('Ctrl Pts',(-39.6157702857969,37.1576174447781,39.941563667896));
#26714=CARTESIAN_POINT('Ctrl Pts',(-36.1599632550759,36.423437812919,36.0275461720274));
#26715=CARTESIAN_POINT('Ctrl Pts',(-36.229636845075,36.376666560942,36.1073050568148));
#26716=CARTESIAN_POINT('Ctrl Pts',(-36.3002901628524,36.3335735174028,36.1883649632048));
#26717=CARTESIAN_POINT('Ctrl Pts',(-36.3717528702068,36.2942625662383,36.2705304633556));
#26718=CARTESIAN_POINT('Ctrl Pts',(-36.4431521219947,36.2549865213736,36.3526230043567));
#26719=CARTESIAN_POINT('Ctrl Pts',(-36.5153592713935,36.2194858855877,36.4358191130872));
#26720=CARTESIAN_POINT('Ctrl Pts',(-36.5882005448549,36.1878460946234,36.5199185699963));
#26721=CARTESIAN_POINT('Ctrl Pts',(-36.6610418183162,36.1562063036593,36.6040180269053));
#26722=CARTESIAN_POINT('Ctrl Pts',(-36.7345171595216,36.1284273819797,36.6890207669698));
#26723=CARTESIAN_POINT('Ctrl Pts',(-36.8084497428955,36.1045761822694,36.7747222228044));
#26724=CARTESIAN_POINT('Ctrl Pts',(-36.8823823262693,36.0807249825591,36.860423678639));
#26725=CARTESIAN_POINT('Ctrl Pts',(-36.9567720946492,36.060801523259,36.9468237839821));
#26726=CARTESIAN_POINT('Ctrl Pts',(-37.0314400218015,36.0448537521174,37.0337146085525));
#26727=CARTESIAN_POINT('Ctrl Pts',(-37.1061079489537,36.0289059809758,37.1206054331229));
#26728=CARTESIAN_POINT('Ctrl Pts',(-37.1810539771475,36.0169339103229,37.2079869097394));
#26729=CARTESIAN_POINT('Ctrl Pts',(-37.2560977414554,36.0089663521146,37.295648746355));
#26730=CARTESIAN_POINT('Ctrl Pts',(-37.3311415057632,36.0009987939063,37.3833105829706));
#26731=CARTESIAN_POINT('Ctrl Pts',(-37.4062829481639,35.9970357543028,37.471252711808));
#26732=CARTESIAN_POINT('Ctrl Pts',(-37.4813412334466,35.9970867707455,37.5592634915561));
#26733=CARTESIAN_POINT('Ctrl Pts',(-37.5563995187293,35.9971377871883,37.6472742713042));
#26734=CARTESIAN_POINT('Ctrl Pts',(-37.6313745888614,36.0012028596377,37.7353536339158));
#26735=CARTESIAN_POINT('Ctrl Pts',(-37.7060860090234,36.0092722051006,37.8232896078133));
#26736=CARTESIAN_POINT('Ctrl Pts',(-37.7807974291853,36.0173415505635,37.9112255817108));
#26737=CARTESIAN_POINT('Ctrl Pts',(-37.8552451416127,36.0294151628007,37.9990180989049));
#26738=CARTESIAN_POINT('Ctrl Pts',(-37.9292499806237,36.0454639854869,38.0864558781395));
#26739=CARTESIAN_POINT('Ctrl Pts',(-38.0032548196346,36.0615128081731,38.173893657374));
#26740=CARTESIAN_POINT('Ctrl Pts',(-38.076816728011,36.0815368288997,38.260976631045));
#26741=CARTESIAN_POINT('Ctrl Pts',(-38.1497586718448,36.1054878579077,38.3474952254818));
#26742=CARTESIAN_POINT('Ctrl Pts',(-38.2227006156786,36.1294388869157,38.4340138199186));
#26743=CARTESIAN_POINT('Ctrl Pts',(-38.2950225385736,36.1573169056868,38.519967968228));
#26744=CARTESIAN_POINT('Ctrl Pts',(-38.3665503907676,36.1890548230498,38.6051508133676));
#26745=CARTESIAN_POINT('Ctrl Pts',(-38.4380782429617,36.2207927404126,38.6903336585073));
#26746=CARTESIAN_POINT('Ctrl Pts',(-38.5088119691518,36.2563905318285,38.7747451346167));
#26747=CARTESIAN_POINT('Ctrl Pts',(-38.5785813417265,36.29576252774,38.8581820972448));
#26748=CARTESIAN_POINT('Ctrl Pts',(-38.6483507143011,36.3351345236515,38.941619059873));
#26749=CARTESIAN_POINT('Ctrl Pts',(-38.7171556793168,36.3782806936176,39.024081444509));
#26750=CARTESIAN_POINT('Ctrl Pts',(-38.7848306509137,36.4250972021714,39.1053707973808));
#26751=CARTESIAN_POINT('Ctrl Pts',(-38.8525056225106,36.4719137107252,39.1866601502525));
#26752=CARTESIAN_POINT('Ctrl Pts',(-38.9190505483647,36.5224005216697,39.2667764085097));
#26753=CARTESIAN_POINT('Ctrl Pts',(-38.9843052816209,36.57643613357,39.3455267645619));
#26754=CARTESIAN_POINT('Ctrl Pts',(-39.049560014877,36.6304717454703,39.4242771206141));
#26755=CARTESIAN_POINT('Ctrl Pts',(-39.1135245050824,36.6880561165477,39.5016615135742));
#26756=CARTESIAN_POINT('Ctrl Pts',(-39.1760448154521,36.749050664396,39.5774937103522));
#26757=CARTESIAN_POINT('Ctrl Pts',(-39.2385651258217,36.8100452122444,39.6533259071301));
#26758=CARTESIAN_POINT('Ctrl Pts',(-39.299641208017,36.8744498897049,39.727605849095));
#26759=CARTESIAN_POINT('Ctrl Pts',(-39.3591260764884,36.9421097006389,39.8001547743209));
#26760=CARTESIAN_POINT('Ctrl Pts',(-39.4186109449598,37.0097695115729,39.8727036995467));
#26761=CARTESIAN_POINT('Ctrl Pts',(-39.4765045537157,37.0806844036681,39.9435215519411));
#26762=CARTESIAN_POINT('Ctrl Pts',(-39.5326675761395,37.1546837133193,40.0124379014345));
#26763=CARTESIAN_POINT('Ctrl Pts',(-36.0054976654609,36.4686568860403,36.0160278574133));
#26764=CARTESIAN_POINT('Ctrl Pts',(-36.0759904836038,36.4183588374172,36.0966094839474));
#26765=CARTESIAN_POINT('Ctrl Pts',(-36.1475625106413,36.3718581992216,36.178614282917));
#26766=CARTESIAN_POINT('Ctrl Pts',(-36.2200338872806,36.3292715261031,36.2618361660942));
#26767=CARTESIAN_POINT('Ctrl Pts',(-36.2924409127019,36.2867226679733,36.3449841521028));
#26768=CARTESIAN_POINT('Ctrl Pts',(-36.3657456305516,36.248080862672,36.4293469921147));
#26769=CARTESIAN_POINT('Ctrl Pts',(-36.4397641725262,36.2134427699113,36.5147130710767));
#26770=CARTESIAN_POINT('Ctrl Pts',(-36.5137827145008,36.1788046771507,36.6000791500389));
#26771=CARTESIAN_POINT('Ctrl Pts',(-36.5885150185374,36.1481703258115,36.6864483963677));
#26772=CARTESIAN_POINT('Ctrl Pts',(-36.663773649802,36.121616307838,36.773604179914));
#26773=CARTESIAN_POINT('Ctrl Pts',(-36.7390322810665,36.0950622898643,36.8607599634603));
#26774=CARTESIAN_POINT('Ctrl Pts',(-36.8148171764651,36.07258862737,36.9487022111505));
#26775=CARTESIAN_POINT('Ctrl Pts',(-36.8909382736109,36.0542514619504,37.0372103630156));
#26776=CARTESIAN_POINT('Ctrl Pts',(-36.9670593707568,36.0359142965309,37.1257185148807));
#26777=CARTESIAN_POINT('Ctrl Pts',(-37.0435166058402,36.0217136434224,37.2147924967226));
#26778=CARTESIAN_POINT('Ctrl Pts',(-37.1201182410057,36.0116849136598,37.3042089236448));
#26779=CARTESIAN_POINT('Ctrl Pts',(-37.196719876171,36.0016561838974,37.3936253505669));
#26780=CARTESIAN_POINT('Ctrl Pts',(-37.2734658472122,35.9957993857637,37.4833841476179));
#26781=CARTESIAN_POINT('Ctrl Pts',(-37.3501637012311,35.9941290232867,37.5732602239549));
#26782=CARTESIAN_POINT('Ctrl Pts',(-37.42686155525,35.9924586608097,37.663136300292));
#26783=CARTESIAN_POINT('Ctrl Pts',(-37.5035112279651,35.9949747352775,37.7531295805852));
#26784=CARTESIAN_POINT('Ctrl Pts',(-37.579920515403,36.0016707719076,37.8430143955194));
#26785=CARTESIAN_POINT('Ctrl Pts',(-37.6563298028409,36.0083668085377,37.9328992104537));
#26786=CARTESIAN_POINT('Ctrl Pts',(-37.7324986409661,36.0192428016173,38.0226754846973));
#26787=CARTESIAN_POINT('Ctrl Pts',(-37.8082360374155,36.0342713307486,38.1121181007901));
#26788=CARTESIAN_POINT('Ctrl Pts',(-37.8839734338648,36.0492998598799,38.2015607168829));
#26789=CARTESIAN_POINT('Ctrl Pts',(-37.9592793251693,36.0684809123782,38.2906695998681));
#26790=CARTESIAN_POINT('Ctrl Pts',(-38.0339648871654,36.091766260255,38.3792213116681));
#26791=CARTESIAN_POINT('Ctrl Pts',(-38.1086504491616,36.1150516081317,38.4677730234682));
#26792=CARTESIAN_POINT('Ctrl Pts',(-38.1827156192643,36.1424412317938,38.555767489876));
#26793=CARTESIAN_POINT('Ctrl Pts',(-38.2559746872202,36.1738663378219,38.6429840712856));
#26794=CARTESIAN_POINT('Ctrl Pts',(-38.3292337551761,36.20529144385,38.7302006526952));
#26795=CARTESIAN_POINT('Ctrl Pts',(-38.4016866595967,36.2407520058409,38.8166392760205));
#26796=CARTESIAN_POINT('Ctrl Pts',(-38.4731517342401,36.2801590100262,38.9020832051809));
#26797=CARTESIAN_POINT('Ctrl Pts',(-38.5446168088833,36.3195660142115,38.9875271343413));
#26798=CARTESIAN_POINT('Ctrl Pts',(-38.6150939938646,36.3629194275101,39.0719762977373));
#26799=CARTESIAN_POINT('Ctrl Pts',(-38.6844065767933,36.4101104620801,39.1552189483062));
#26800=CARTESIAN_POINT('Ctrl Pts',(-38.753719159722,36.45730149665,39.2384615988751));
#26801=CARTESIAN_POINT('Ctrl Pts',(-38.8218670825167,36.5083301128978,39.3204976668618));
#26802=CARTESIAN_POINT('Ctrl Pts',(-38.8886794716687,36.5630682941429,39.4011214547246));
#26803=CARTESIAN_POINT('Ctrl Pts',(-38.9554918608208,36.617806475388,39.4817452425874));
#26804=CARTESIAN_POINT('Ctrl Pts',(-39.0209686603426,36.6762541757227,39.5609566827645));
#26805=CARTESIAN_POINT('Ctrl Pts',(-39.0849456914012,36.7382647910941,39.6385571574444));
#26806=CARTESIAN_POINT('Ctrl Pts',(-39.1489227224598,36.8002754064656,39.7161576321244));
#26807=CARTESIAN_POINT('Ctrl Pts',(-39.2113999314413,36.8658488848813,39.7921470762765));
#26808=CARTESIAN_POINT('Ctrl Pts',(-39.2722206564667,36.9348207694045,39.8663349465842));
#26809=CARTESIAN_POINT('Ctrl Pts',(-39.333041381492,37.0037926539277,39.9405228168919));
#26810=CARTESIAN_POINT('Ctrl Pts',(-39.3922055715889,37.0761628867415,40.0129090511807));
#26811=CARTESIAN_POINT('Ctrl Pts',(-39.4495648664821,37.1517499818605,40.0833121349731));
#26812=CARTESIAN_POINT('Ctrl Pts',(-35.8535977491494,36.5168641145602,36.0072213658969));
#26813=CARTESIAN_POINT('Ctrl Pts',(-35.9247900751538,36.4629824222449,36.088486901381));
#26814=CARTESIAN_POINT('Ctrl Pts',(-35.9971669834831,36.4130120864817,36.1713048624591));
#26815=CARTESIAN_POINT('Ctrl Pts',(-36.0705389847832,36.3670836000417,36.2554584119513));
#26816=CARTESIAN_POINT('Ctrl Pts',(-36.1438458351524,36.3211958959654,36.3395372369984));
#26817=CARTESIAN_POINT('Ctrl Pts',(-36.2181459453587,36.2793429079946,36.4249492030928));
#26818=CARTESIAN_POINT('Ctrl Pts',(-36.293245158042,36.2416337108208,36.5114711057138));
#26819=CARTESIAN_POINT('Ctrl Pts',(-36.3683443707253,36.2039245136471,36.5979930083348));
#26820=CARTESIAN_POINT('Ctrl Pts',(-36.4442426175417,36.170359141384,36.6856247687362));
#26821=CARTESIAN_POINT('Ctrl Pts',(-36.5207415821637,36.1410250303205,36.774137402972));
#26822=CARTESIAN_POINT('Ctrl Pts',(-36.5972405467856,36.111690919257,36.8626500372078));
#26823=CARTESIAN_POINT('Ctrl Pts',(-36.6743401596069,36.0865880958987,36.9520434647347));
#26824=CARTESIAN_POINT('Ctrl Pts',(-36.7518389803048,36.0657819033363,37.0420841172522));
#26825=CARTESIAN_POINT('Ctrl Pts',(-36.8293378010027,36.0449757107739,37.1321247697696));
#26826=CARTESIAN_POINT('Ctrl Pts',(-36.9072357590715,36.0284661677672,37.2228125653567));
#26827=CARTESIAN_POINT('Ctrl Pts',(-36.9853293413838,36.0162961846062,37.3139105702477));
#26828=CARTESIAN_POINT('Ctrl Pts',(-37.0634229236962,36.0041262014452,37.4050085751388));
#26829=CARTESIAN_POINT('Ctrl Pts',(-37.1417120592141,35.9962957890467,37.496516706462));
#26830=CARTESIAN_POINT('Ctrl Pts',(-37.2199922239388,35.9928252022519,37.5881959013455));
#26831=CARTESIAN_POINT('Ctrl Pts',(-37.2982723886635,35.989354615457,37.6798750962289));
#26832=CARTESIAN_POINT('Ctrl Pts',(-37.3765435113947,35.9902438572833,37.7717252712815));
#26833=CARTESIAN_POINT('Ctrl Pts',(-37.4546011244074,35.9954904225816,37.8635064819135));
#26834=CARTESIAN_POINT('Ctrl Pts',(-37.5326587374201,36.0007369878799,37.9552876925455));
#26835=CARTESIAN_POINT('Ctrl Pts',(-37.6105027697224,36.0103408717529,38.0469998552811));
#26836=CARTESIAN_POINT('Ctrl Pts',(-37.6879298766621,36.0242768231652,38.1384033957348));
#26837=CARTESIAN_POINT('Ctrl Pts',(-37.7653569836018,36.0382127745774,38.2298069361886));
#26838=CARTESIAN_POINT('Ctrl Pts',(-37.8423670947653,36.0564807807428,38.3209017712344));
#26839=CARTESIAN_POINT('Ctrl Pts',(-37.9187590494708,36.0790329774082,38.4114499466273));
#26840=CARTESIAN_POINT('Ctrl Pts',(-37.9951510041764,36.1015851740735,38.5019981220201));
#26841=CARTESIAN_POINT('Ctrl Pts',(-38.0709247329551,36.1284215406308,38.5919995554163));
#26842=CARTESIAN_POINT('Ctrl Pts',(-38.1458823085678,36.1594718501479,38.6812191541513));
#26843=CARTESIAN_POINT('Ctrl Pts',(-38.2208398841804,36.1905221596649,38.7704387528863));
#26844=CARTESIAN_POINT('Ctrl Pts',(-38.2949812384645,36.2257863838195,38.8588764358279));
#26845=CARTESIAN_POINT('Ctrl Pts',(-38.3681127102037,36.2651723000987,38.9463011983719));
#26846=CARTESIAN_POINT('Ctrl Pts',(-38.4412441819429,36.3045582163779,39.033725960916));
#26847=CARTESIAN_POINT('Ctrl Pts',(-38.5133657046363,36.348065788893,39.1201377235641));
#26848=CARTESIAN_POINT('Ctrl Pts',(-38.5842888934035,36.3955812812933,39.2053107749063));
#26849=CARTESIAN_POINT('Ctrl Pts',(-38.6552120821707,36.4430967736936,39.2904838262485));
#26850=CARTESIAN_POINT('Ctrl Pts',(-38.7249368725185,36.4946201427111,39.3744180888342));
#26851=CARTESIAN_POINT('Ctrl Pts',(-38.7932811386868,36.5500167320324,39.4568943219588));
#26852=CARTESIAN_POINT('Ctrl Pts',(-38.8616254048551,36.6054133213537,39.5393705550833));
#26853=CARTESIAN_POINT('Ctrl Pts',(-38.9285890846943,36.6646830805569,39.6203886837473));
#26854=CARTESIAN_POINT('Ctrl Pts',(-38.9939972617029,36.7276711362782,39.6997370817098));
#26855=CARTESIAN_POINT('Ctrl Pts',(-39.0594054387115,36.7906591919996,39.7790854796723));
#26856=CARTESIAN_POINT('Ctrl Pts',(-39.1232580534071,36.857365486926,39.8567640747754));
#26857=CARTESIAN_POINT('Ctrl Pts',(-39.1853883110917,36.92761573893,39.932569959291));
#26858=CARTESIAN_POINT('Ctrl Pts',(-39.2475185687763,36.9978659909341,40.0083758438067));
#26859=CARTESIAN_POINT('Ctrl Pts',(-39.3079264129444,37.0716601361098,40.0823089487944));
#26860=CARTESIAN_POINT('Ctrl Pts',(-39.3664540409007,37.1488053930167,40.1541761436298));
#26861=CARTESIAN_POINT('Ctrl Pts',(-35.7040417827465,36.5677479921179,36.0008564624337));
#26862=CARTESIAN_POINT('Ctrl Pts',(-35.7758191971864,36.5102371490812,36.0826718939149));
#26863=CARTESIAN_POINT('Ctrl Pts',(-35.8488922038129,36.4567456200151,36.1661759105181));
#26864=CARTESIAN_POINT('Ctrl Pts',(-35.9230616496862,36.4074191785411,36.2511409301588));
#26865=CARTESIAN_POINT('Ctrl Pts',(-35.9971652365349,36.3581365366571,36.3360305048066));
#26866=CARTESIAN_POINT('Ctrl Pts',(-36.0723632430923,36.3130116375408,36.422378405151));
#26867=CARTESIAN_POINT('Ctrl Pts',(-36.1484510914768,36.2721672445033,36.5099497197717));
#26868=CARTESIAN_POINT('Ctrl Pts',(-36.2245389398613,36.2313228514658,36.5975210343924));
#26869=CARTESIAN_POINT('Ctrl Pts',(-36.3015165548838,36.1947590048691,36.6863156767524));
#26870=CARTESIAN_POINT('Ctrl Pts',(-36.3791745171975,36.1625751774866,36.7760920790142));
#26871=CARTESIAN_POINT('Ctrl Pts',(-36.4568324795112,36.1303913501041,36.8658684812761));
#26872=CARTESIAN_POINT('Ctrl Pts',(-36.5351707123754,36.1025875737396,36.9566265547237));
#26873=CARTESIAN_POINT('Ctrl Pts',(-36.6139760948518,36.0792394891969,37.0481193899609));
#26874=CARTESIAN_POINT('Ctrl Pts',(-36.6927814773281,36.0558914046543,37.139612225198));
#26875=CARTESIAN_POINT('Ctrl Pts',(-36.7720539315419,36.0369990350059,37.2318397318125));
#26876=CARTESIAN_POINT('Ctrl Pts',(-36.8515777949845,36.0226137773715,37.3245510027818));
#26877=CARTESIAN_POINT('Ctrl Pts',(-36.9311016584271,36.0082285197373,37.4172622737511));
#26878=CARTESIAN_POINT('Ctrl Pts',(-37.0108768525138,35.9983503883324,37.510457217459));
#26879=CARTESIAN_POINT('Ctrl Pts',(-37.0906863470207,35.9930062568374,37.6038822949484));
#26880=CARTESIAN_POINT('Ctrl Pts',(-37.1704958415277,35.9876621253424,37.6973073724378));
#26881=CARTESIAN_POINT('Ctrl Pts',(-37.2503395575878,35.9868519990383,37.7909624913871));
#26882=CARTESIAN_POINT('Ctrl Pts',(-37.3300002785618,35.9905780818921,37.8845928609221));
#26883=CARTESIAN_POINT('Ctrl Pts',(-37.4096609995357,35.9943041647459,37.978223230457));
#26884=CARTESIAN_POINT('Ctrl Pts',(-37.4891386467036,36.0025664530755,38.0718287580532));
#26885=CARTESIAN_POINT('Ctrl Pts',(-37.5682169993246,36.0153424691381,38.1651547877508));
#26886=CARTESIAN_POINT('Ctrl Pts',(-37.6472953519455,36.0281184852008,38.2584808174484));
#26887=CARTESIAN_POINT('Ctrl Pts',(-37.7259743318751,36.0454082163714,38.3515272570235));
#26888=CARTESIAN_POINT('Ctrl Pts',(-37.804039891165,36.0671646255444,38.4440409715282));
#26889=CARTESIAN_POINT('Ctrl Pts',(-37.8821054504548,36.0889210347174,38.5365546860328));
#26890=CARTESIAN_POINT('Ctrl Pts',(-37.9595575119613,36.1151441003934,38.6285355840458));
#26891=CARTESIAN_POINT('Ctrl Pts',(-38.0361853655954,36.1457624821276,38.7197334294491));
#26892=CARTESIAN_POINT('Ctrl Pts',(-38.1128132192295,36.1763808638618,38.8109312748524));
#26893=CARTESIAN_POINT('Ctrl Pts',(-38.1886167892683,36.2113945313976,38.9013459775251));
#26894=CARTESIAN_POINT('Ctrl Pts',(-38.2633898503812,36.2507082292586,38.9907315622191));
#26895=CARTESIAN_POINT('Ctrl Pts',(-38.338162911494,36.2900219271197,39.0801171469131));
#26896=CARTESIAN_POINT('Ctrl Pts',(-38.411905389791,36.3336356164567,39.1684735252984));
#26897=CARTESIAN_POINT('Ctrl Pts',(-38.4844166671882,36.381430645239,39.2555603218448));
#26898=CARTESIAN_POINT('Ctrl Pts',(-38.5569279445854,36.4292256740213,39.3426471183912));
#26899=CARTESIAN_POINT('Ctrl Pts',(-38.6282079494279,36.4812019950186,39.4284642470403));
#26900=CARTESIAN_POINT('Ctrl Pts',(-38.6980627628468,36.537218205471,39.5127782403483));
#26901=CARTESIAN_POINT('Ctrl Pts',(-38.7679175762657,36.5932344159235,39.5970922336563));
#26902=CARTESIAN_POINT('Ctrl Pts',(-38.8363471292311,36.6532904604767,39.679903008305));
#26903=CARTESIAN_POINT('Ctrl Pts',(-38.903165257593,36.7172229552999,39.7609852757047));
#26904=CARTESIAN_POINT('Ctrl Pts',(-38.9699833859549,36.7811554501232,39.8420675431044));
#26905=CARTESIAN_POINT('Ctrl Pts',(-39.0351900236842,36.8489643320392,39.9214212231304));
#26906=CARTESIAN_POINT('Ctrl Pts',(-39.098607774645,36.9204651254473,39.9988304322975));
#26907=CARTESIAN_POINT('Ctrl Pts',(-39.1620255256058,36.9919659188554,40.0762396414646));
#26908=CARTESIAN_POINT('Ctrl Pts',(-39.2236543271292,37.0671585530995,40.1517043032776));
#26909=CARTESIAN_POINT('Ctrl Pts',(-39.2833265166636,37.1458384649135,40.2250191144136));
#26910=CARTESIAN_POINT('Ctrl Pts',(-35.5544858163436,36.6186318696757,35.9944915589704));
#26911=CARTESIAN_POINT('Ctrl Pts',(-35.6268483192189,36.5574918759175,36.0768568864488));
#26912=CARTESIAN_POINT('Ctrl Pts',(-35.7006174241427,36.5004791535485,36.1610469585772));
#26913=CARTESIAN_POINT('Ctrl Pts',(-35.7755843145893,36.4477547570404,36.2468234483664));
#26914=CARTESIAN_POINT('Ctrl Pts',(-35.8504846379174,36.3950771773488,36.3325237726148));
#26915=CARTESIAN_POINT('Ctrl Pts',(-35.9265805408259,36.346680367087,36.4198076072092));
#26916=CARTESIAN_POINT('Ctrl Pts',(-36.0036570249117,36.3027007781857,36.5084283338296));
#26917=CARTESIAN_POINT('Ctrl Pts',(-36.0807335089974,36.2587211892845,36.59704906045));
#26918=CARTESIAN_POINT('Ctrl Pts',(-36.1587904922259,36.2191588683541,36.6870065847686));
#26919=CARTESIAN_POINT('Ctrl Pts',(-36.2376074522313,36.1841253246526,36.7780467550565));
#26920=CARTESIAN_POINT('Ctrl Pts',(-36.3164244122368,36.1490917809511,36.8690869253443));
#26921=CARTESIAN_POINT('Ctrl Pts',(-36.396001265144,36.1185870515805,36.9612096447127));
#26922=CARTESIAN_POINT('Ctrl Pts',(-36.4761132093987,36.0926970750576,37.0541546626696));
#26923=CARTESIAN_POINT('Ctrl Pts',(-36.5562251536535,36.0668070985348,37.1470996806264));
#26924=CARTESIAN_POINT('Ctrl Pts',(-36.6368721040124,36.0455319022446,37.2408668982683));
#26925=CARTESIAN_POINT('Ctrl Pts',(-36.7178262485852,36.028931370137,37.3351914353158));
#26926=CARTESIAN_POINT('Ctrl Pts',(-36.798780393158,36.0123308380293,37.4295159723634));
#26927=CARTESIAN_POINT('Ctrl Pts',(-36.8800416458136,36.0004049876181,37.5243977284558));
#26928=CARTESIAN_POINT('Ctrl Pts',(-36.9613804701027,35.9931873114229,37.6195686885513));
#26929=CARTESIAN_POINT('Ctrl Pts',(-37.0427192943918,35.9859696352278,37.7147396486466));
#26930=CARTESIAN_POINT('Ctrl Pts',(-37.124135603781,35.9834601407934,37.8101997114927));
#26931=CARTESIAN_POINT('Ctrl Pts',(-37.2053994327162,35.9856657412027,37.9056792399306));
#26932=CARTESIAN_POINT('Ctrl Pts',(-37.2866632616515,35.9878713416119,38.0011587683686));
#26933=CARTESIAN_POINT('Ctrl Pts',(-37.3677745236849,35.994792034398,38.0966576608254));
#26934=CARTESIAN_POINT('Ctrl Pts',(-37.448504121987,36.0064081151111,38.1919061797668));
#26935=CARTESIAN_POINT('Ctrl Pts',(-37.5292337202892,36.0180241958241,38.2871546987081));
#26936=CARTESIAN_POINT('Ctrl Pts',(-37.609581568985,36.0343356519999,38.3821527428127));
#26937=CARTESIAN_POINT('Ctrl Pts',(-37.6893207328591,36.0552962736806,38.4766319964291));
#26938=CARTESIAN_POINT('Ctrl Pts',(-37.7690598967332,36.0762568953614,38.5711112500455));
#26939=CARTESIAN_POINT('Ctrl Pts',(-37.8481902909676,36.1018666601559,38.6650716126754));
#26940=CARTESIAN_POINT('Ctrl Pts',(-37.9264884226231,36.1320531141073,38.7582477047469));
#26941=CARTESIAN_POINT('Ctrl Pts',(-38.0047865542786,36.1622395680588,38.8514237968184));
#26942=CARTESIAN_POINT('Ctrl Pts',(-38.0822523400722,36.1970026789757,38.9438155192224));
#26943=CARTESIAN_POINT('Ctrl Pts',(-38.1586669905587,36.2362441584186,39.0351619260663));
#26944=CARTESIAN_POINT('Ctrl Pts',(-38.2350816410452,36.2754856378615,39.1265083329102));
#26945=CARTESIAN_POINT('Ctrl Pts',(-38.3104450749457,36.3192054440204,39.2168093270328));
#26946=CARTESIAN_POINT('Ctrl Pts',(-38.384544440973,36.3672800091847,39.3058098687833));
#26947=CARTESIAN_POINT('Ctrl Pts',(-38.4586438070002,36.415354574349,39.3948104105338));
#26948=CARTESIAN_POINT('Ctrl Pts',(-38.5314790263374,36.467783847326,39.4825104052464));
#26949=CARTESIAN_POINT('Ctrl Pts',(-38.6028443870069,36.5244196789096,39.5686621587378));
#26950=CARTESIAN_POINT('Ctrl Pts',(-38.6742097476763,36.5810555104933,39.6548139122292));
#26951=CARTESIAN_POINT('Ctrl Pts',(-38.744105173768,36.6418978403966,39.7394173328626));
#26952=CARTESIAN_POINT('Ctrl Pts',(-38.8123332534831,36.7067747743217,39.8222334696996));
#26953=CARTESIAN_POINT('Ctrl Pts',(-38.8805613331982,36.7716517082468,39.9050496065365));
#26954=CARTESIAN_POINT('Ctrl Pts',(-38.9471219939613,36.8405631771523,39.9860783714854));
#26955=CARTESIAN_POINT('Ctrl Pts',(-39.0118272381983,36.9133145119646,40.065090905304));
#26956=CARTESIAN_POINT('Ctrl Pts',(-39.0765324824353,36.9860658467768,40.1441034391225));
#26957=CARTESIAN_POINT('Ctrl Pts',(-39.139382241314,37.0626569700893,40.2210996577609));
#26958=CARTESIAN_POINT('Ctrl Pts',(-39.2001989924265,37.1428715368103,40.2958620851973));
#26959=CARTESIAN_POINT('Ctrl Pts',(-35.4072750999858,36.6721941387054,35.9905697714741));
#26960=CARTESIAN_POINT('Ctrl Pts',(-35.4801082384467,36.607379442505,36.0733509486624));
#26961=CARTESIAN_POINT('Ctrl Pts',(-35.5544646259996,36.5467939873462,36.1580999369808));
#26962=CARTESIAN_POINT('Ctrl Pts',(-35.6301257489358,36.4906154512438,36.2445676684546));
#26963=CARTESIAN_POINT('Ctrl Pts',(-35.7057196883076,36.4344867990733,36.3309586205972));
#26964=CARTESIAN_POINT('Ctrl Pts',(-35.7826159602713,36.3827573072814,36.4190651657937));
#26965=CARTESIAN_POINT('Ctrl Pts',(-35.8605890143666,36.335578390006,36.5086288612754));
#26966=CARTESIAN_POINT('Ctrl Pts',(-35.9385620684619,36.2883994727305,36.5981925567571));
#26967=CARTESIAN_POINT('Ctrl Pts',(-36.0176118152452,36.2457711838453,36.6892132997768));
#26968=CARTESIAN_POINT('Ctrl Pts',(-36.0975064077398,36.2078182611662,36.7814241245148));
#26969=CARTESIAN_POINT('Ctrl Pts',(-36.1774010002343,36.1698653384872,36.8736349492527));
#26970=CARTESIAN_POINT('Ctrl Pts',(-36.2581403468076,36.1365878253204,36.9670357499442));
#26971=CARTESIAN_POINT('Ctrl Pts',(-36.3394876625489,36.1080830540372,37.0613526021471));
#26972=CARTESIAN_POINT('Ctrl Pts',(-36.4208349782902,36.0795782827539,37.1556694543499));
#26973=CARTESIAN_POINT('Ctrl Pts',(-36.502790169914,36.0558462858404,37.2509022499006));
#26974=CARTESIAN_POINT('Ctrl Pts',(-36.5851129019827,36.0369564215669,37.3467717108003));
#26975=CARTESIAN_POINT('Ctrl Pts',(-36.6674356340514,36.0180665572934,37.4426411717001));
#26976=CARTESIAN_POINT('Ctrl Pts',(-36.7501258121725,36.0040188471366,37.5391471880195));
#26977=CARTESIAN_POINT('Ctrl Pts',(-36.8329409584958,35.9948542703932,37.6360067645168));
#26978=CARTESIAN_POINT('Ctrl Pts',(-36.9157561048191,35.9856896936499,37.732866341014));
#26979=CARTESIAN_POINT('Ctrl Pts',(-36.9986961243973,35.9814082606621,37.8300793666369));
#26980=CARTESIAN_POINT('Ctrl Pts',(-37.0815178175531,35.9820223330219,37.9273607868886));
#26981=CARTESIAN_POINT('Ctrl Pts',(-37.1643395107089,35.9826364053818,38.0246422071404));
#26982=CARTESIAN_POINT('Ctrl Pts',(-37.2470427824952,35.9881459822369,38.1219919104955));
#26983=CARTESIAN_POINT('Ctrl Pts',(-37.3293851361536,35.9985347362742,38.219124453167));
#26984=CARTESIAN_POINT('Ctrl Pts',(-37.411727489812,36.0089234903114,38.3162569958385));
#26985=CARTESIAN_POINT('Ctrl Pts',(-37.4937088309511,36.0241914094893,38.4131722664797));
#26986=CARTESIAN_POINT('Ctrl Pts',(-37.5750887863036,36.0442935743273,38.5095861041859));
#26987=CARTESIAN_POINT('Ctrl Pts',(-37.6564687416562,36.0643957391652,38.6059999418921));
#26988=CARTESIAN_POINT('Ctrl Pts',(-37.7372472179389,36.0893321265037,38.7019122361468));
#26989=CARTESIAN_POINT('Ctrl Pts',(-37.8171873734666,36.1190294887985,38.7970417735272));
#26990=CARTESIAN_POINT('Ctrl Pts',(-37.8971275289942,36.1487268510933,38.8921713109075));
#26991=CARTESIAN_POINT('Ctrl Pts',(-37.9762292721368,36.1831851542028,38.9865179823737));
#26992=CARTESIAN_POINT('Ctrl Pts',(-38.0542606801644,36.2223032524384,39.079805169276));
#26993=CARTESIAN_POINT('Ctrl Pts',(-38.1322920881921,36.261421350674,39.1730923561784));
#26994=CARTESIAN_POINT('Ctrl Pts',(-38.2092530716641,36.3051991991118,39.2653199515914));
#26995=CARTESIAN_POINT('Ctrl Pts',(-38.2849179853468,36.3535083471339,39.3562175519869));
#26996=CARTESIAN_POINT('Ctrl Pts',(-38.3605828990296,36.4018174951558,39.4471151523824));
#26997=CARTESIAN_POINT('Ctrl Pts',(-38.4349516561949,36.4546578873189,39.5366826535746));
#26998=CARTESIAN_POINT('Ctrl Pts',(-38.5078062108692,36.5118745211112,39.6246574510852));
#26999=CARTESIAN_POINT('Ctrl Pts',(-38.5806607655435,36.5690911549036,39.7126322485958));
#27000=CARTESIAN_POINT('Ctrl Pts',(-38.6520010342182,36.6306839646873,39.7990142415882));
#27001=CARTESIAN_POINT('Ctrl Pts',(-38.7216178474355,36.6964723045064,39.8835501628792));
#27002=CARTESIAN_POINT('Ctrl Pts',(-38.7912346606527,36.7622606443254,39.9680860841702));
#27003=CARTESIAN_POINT('Ctrl Pts',(-38.8591279386121,36.8322444387312,40.0507758368621));
#27004=CARTESIAN_POINT('Ctrl Pts',(-38.9250986136492,36.9062184568694,40.1313769746322));
#27005=CARTESIAN_POINT('Ctrl Pts',(-38.9910692886862,36.9801924750076,40.2119781124024));
#27006=CARTESIAN_POINT('Ctrl Pts',(-39.0551172851754,37.0581566320604,40.2904905428586));
#27007=CARTESIAN_POINT('Ctrl Pts',(-39.1170548033789,37.1398823147253,40.366684060748));
#27008=CARTESIAN_POINT('Ctrl Pts',(-35.2622498364415,36.7281963563022,35.9888869492133));
#27009=CARTESIAN_POINT('Ctrl Pts',(-35.3354429836358,36.65967121659,36.0719528236328));
#27010=CARTESIAN_POINT('Ctrl Pts',(-35.410281415356,36.5954705570286,36.1571363122166));
#27011=CARTESIAN_POINT('Ctrl Pts',(-35.4865369655357,36.5357900959079,36.2441777084119));
#27012=CARTESIAN_POINT('Ctrl Pts',(-35.5627248043271,36.476162628266,36.3311418158883));
#27013=CARTESIAN_POINT('Ctrl Pts',(-35.6403271517951,36.4210474089236,36.419960425412));
#27014=CARTESIAN_POINT('Ctrl Pts',(-35.7191078392476,36.3706121710703,36.5103632336284));
#27015=CARTESIAN_POINT('Ctrl Pts',(-35.7978885267002,36.320176933217,36.6007660418448));
#27016=CARTESIAN_POINT('Ctrl Pts',(-35.8778474567011,36.2744217392313,36.6927529369434));
#27017=CARTESIAN_POINT('Ctrl Pts',(-35.9587412887259,36.2334858367607,36.7860439734662));
#27018=CARTESIAN_POINT('Ctrl Pts',(-36.0396351207508,36.1925499342901,36.879335009989));
#27019=CARTESIAN_POINT('Ctrl Pts',(-36.1214637547498,36.1564333739643,36.9739300725531));
#27020=CARTESIAN_POINT('Ctrl Pts',(-36.2039781600931,36.1252460699945,37.0695412782153));
#27021=CARTESIAN_POINT('Ctrl Pts',(-36.2864925654364,36.0940587660247,37.1651524838775));
#27022=CARTESIAN_POINT('Ctrl Pts',(-36.3696926400698,36.0678007569836,37.2617797143853));
#27023=CARTESIAN_POINT('Ctrl Pts',(-36.4533251796323,36.0465519543668,37.3591289022602));
#27024=CARTESIAN_POINT('Ctrl Pts',(-36.5369577191948,36.0253031517499,37.4564780901352));
#27025=CARTESIAN_POINT('Ctrl Pts',(-36.6210226202494,36.0090635818379,37.5545491149753));
#27026=CARTESIAN_POINT('Ctrl Pts',(-36.7052640464922,35.9978826668211,37.6530435153755));
#27027=CARTESIAN_POINT('Ctrl Pts',(-36.789505472735,35.9867017518044,37.7515379157757));
#27028=CARTESIAN_POINT('Ctrl Pts',(-36.873923319976,35.9805795055114,37.8504555699178));
#27029=CARTESIAN_POINT('Ctrl Pts',(-36.9582606777837,35.9795345598903,37.9494954398334));
#27030=CARTESIAN_POINT('Ctrl Pts',(-37.0425980355914,35.9784896142691,38.0485353097491));
#27031=CARTESIAN_POINT('Ctrl Pts',(-37.1268547996569,35.9825219706122,38.1476972729454));
#27032=CARTESIAN_POINT('Ctrl Pts',(-37.2107745497763,35.9916193571731,38.2466795479439));
#27033=CARTESIAN_POINT('Ctrl Pts',(-37.2946942998957,36.0007167437339,38.3456618229425));
#27034=CARTESIAN_POINT('Ctrl Pts',(-37.3782769322767,36.0148791492609,38.4444642873216));
#27035=CARTESIAN_POINT('Ctrl Pts',(-37.461268078313,36.0340634730374,38.5427862536723));
#27036=CARTESIAN_POINT('Ctrl Pts',(-37.5442592243492,36.0532477968139,38.641108220023));
#27037=CARTESIAN_POINT('Ctrl Pts',(-37.6266587813969,36.0774540151126,38.7389495667403));
#27038=CARTESIAN_POINT('Ctrl Pts',(-37.7082159813253,36.1066084606916,38.8360125314027));
#27039=CARTESIAN_POINT('Ctrl Pts',(-37.7897731812537,36.1357629062705,38.9330754960651));
#27040=CARTESIAN_POINT('Ctrl Pts',(-37.8704879231926,36.1698655430712,39.0293599586248));
#27041=CARTESIAN_POINT('Ctrl Pts',(-37.9501145664407,36.2088125858941,39.1245728947555));
#27042=CARTESIAN_POINT('Ctrl Pts',(-38.029741209689,36.2477596287169,39.2197858308861));
#27043=CARTESIAN_POINT('Ctrl Pts',(-38.1082796557639,36.291551029392,39.3139271228279));
#27044=CARTESIAN_POINT('Ctrl Pts',(-38.185490887127,36.3400535167211,39.4067102686062));
#27045=CARTESIAN_POINT('Ctrl Pts',(-38.2627021184901,36.3885560040504,39.4994934143845));
#27046=CARTESIAN_POINT('Ctrl Pts',(-38.338586039646,36.4417695180457,39.5909182992447));
#27047=CARTESIAN_POINT('Ctrl Pts',(-38.4129117116221,36.4995321130133,39.6807066881051));
#27048=CARTESIAN_POINT('Ctrl Pts',(-38.4872373835982,36.5572947079808,39.7704950769655));
#27049=CARTESIAN_POINT('Ctrl Pts',(-38.5600047144681,36.6196063124796,39.8586468587756));
#27050=CARTESIAN_POINT('Ctrl Pts',(-38.6309922500372,36.6862772924249,39.94489375955));
#27051=CARTESIAN_POINT('Ctrl Pts',(-38.7019797856063,36.7529482723702,40.0311406603245));
#27052=CARTESIAN_POINT('Ctrl Pts',(-38.771187438077,36.8239785453029,40.1154825733928));
#27053=CARTESIAN_POINT('Ctrl Pts',(-38.8384045864911,36.89915194345,40.1976628194154));
#27054=CARTESIAN_POINT('Ctrl Pts',(-38.9056217349053,36.974325341597,40.279843065438));
#27055=CARTESIAN_POINT('Ctrl Pts',(-38.9708482961285,37.0536417719834,40.3598615427741));
#27056=CARTESIAN_POINT('Ctrl Pts',(-39.0338857649331,37.1368598494162,40.4374747296777));
#27057=CARTESIAN_POINT('Ctrl Pts',(-35.1172245728972,36.7841985738989,35.9872041269524));
#27058=CARTESIAN_POINT('Ctrl Pts',(-35.1907777288249,36.711962990675,36.0705546986032));
#27059=CARTESIAN_POINT('Ctrl Pts',(-35.2660982047123,36.6441471267109,36.1561726874525));
#27060=CARTESIAN_POINT('Ctrl Pts',(-35.3429481821355,36.580964740572,36.2437877483692));
#27061=CARTESIAN_POINT('Ctrl Pts',(-35.4197299203466,36.5178384574586,36.3313250111794));
#27062=CARTESIAN_POINT('Ctrl Pts',(-35.4980383433188,36.4593375105657,36.4208556850302));
#27063=CARTESIAN_POINT('Ctrl Pts',(-35.5776266641287,36.4056459521345,36.5120976059814));
#27064=CARTESIAN_POINT('Ctrl Pts',(-35.6572149849385,36.3519543937034,36.6033395269325));
#27065=CARTESIAN_POINT('Ctrl Pts',(-35.7380830981569,36.3030722946172,36.6962925741101));
#27066=CARTESIAN_POINT('Ctrl Pts',(-35.8199761697121,36.2591534123552,36.7906638224176));
#27067=CARTESIAN_POINT('Ctrl Pts',(-35.9018692412672,36.2152345300931,36.8850350707252));
#27068=CARTESIAN_POINT('Ctrl Pts',(-35.9847871626919,36.1762789226082,36.980824395162));
#27069=CARTESIAN_POINT('Ctrl Pts',(-36.0684686576372,36.1424090859519,37.0777299542835));
#27070=CARTESIAN_POINT('Ctrl Pts',(-36.1521501525826,36.1085392492955,37.174635513405));
#27071=CARTESIAN_POINT('Ctrl Pts',(-36.2365951102256,36.0797552281268,37.27265717887));
#27072=CARTESIAN_POINT('Ctrl Pts',(-36.321537457282,36.0561474871666,37.3714860937201));
#27073=CARTESIAN_POINT('Ctrl Pts',(-36.4064798043383,36.0325397462063,37.4703150085703));
#27074=CARTESIAN_POINT('Ctrl Pts',(-36.4919194283263,36.0141083165392,37.5699510419312));
#27075=CARTESIAN_POINT('Ctrl Pts',(-36.5775871344886,36.0009110632491,37.6700802662343));
#27076=CARTESIAN_POINT('Ctrl Pts',(-36.6632548406509,35.9877138099589,37.7702094905375));
#27077=CARTESIAN_POINT('Ctrl Pts',(-36.7491505155547,35.9797507503608,37.8708317731987));
#27078=CARTESIAN_POINT('Ctrl Pts',(-36.8350035380143,35.9770467867587,37.9716300927782));
#27079=CARTESIAN_POINT('Ctrl Pts',(-36.9208565604738,35.9743428231565,38.0724284123577));
#27080=CARTESIAN_POINT('Ctrl Pts',(-37.0066668168186,35.9768979589874,38.1734026353953));
#27081=CARTESIAN_POINT('Ctrl Pts',(-37.092163963399,35.9847039780719,38.274234642721));
#27082=CARTESIAN_POINT('Ctrl Pts',(-37.1776611099795,35.9925099971564,38.3750666500466));
#27083=CARTESIAN_POINT('Ctrl Pts',(-37.2628450336024,36.0055668890324,38.4757563081636));
#27084=CARTESIAN_POINT('Ctrl Pts',(-37.3474473703222,36.0238333717476,38.5759864031588));
#27085=CARTESIAN_POINT('Ctrl Pts',(-37.4320497070421,36.0420998544626,38.6762164981539));
#27086=CARTESIAN_POINT('Ctrl Pts',(-37.5160703448549,36.0655759037215,38.7759868973337));
#27087=CARTESIAN_POINT('Ctrl Pts',(-37.5992445891841,36.0941874325846,38.8749832892782));
#27088=CARTESIAN_POINT('Ctrl Pts',(-37.6824188335133,36.1227989614476,38.9739796812228));
#27089=CARTESIAN_POINT('Ctrl Pts',(-37.7647465742484,36.1565459319396,39.072201934876));
#27090=CARTESIAN_POINT('Ctrl Pts',(-37.8459684527171,36.1953219193496,39.169340620235));
#27091=CARTESIAN_POINT('Ctrl Pts',(-37.9271903311858,36.2340979067598,39.2664793055939));
#27092=CARTESIAN_POINT('Ctrl Pts',(-38.0073062398638,36.2779028596721,39.3625342940644));
#27093=CARTESIAN_POINT('Ctrl Pts',(-38.0860637889071,36.3265986863085,39.4572029852256));
#27094=CARTESIAN_POINT('Ctrl Pts',(-38.1648213379505,36.375294512945,39.5518716763867));
#27095=CARTESIAN_POINT('Ctrl Pts',(-38.2422204230971,36.4288811487726,39.6451539449147));
#27096=CARTESIAN_POINT('Ctrl Pts',(-38.318017212375,36.4871897049153,39.736755925125));
#27097=CARTESIAN_POINT('Ctrl Pts',(-38.3938140016529,36.5454982610581,39.8283579053353));
#27098=CARTESIAN_POINT('Ctrl Pts',(-38.468008394718,36.6085286602719,39.9182794759629));
#27099=CARTESIAN_POINT('Ctrl Pts',(-38.540366652639,36.6760822803433,40.0062373562209));
#27100=CARTESIAN_POINT('Ctrl Pts',(-38.61272491056,36.7436359004149,40.0941952364787));
#27101=CARTESIAN_POINT('Ctrl Pts',(-38.6832469375418,36.8157126518747,40.1801893099235));
#27102=CARTESIAN_POINT('Ctrl Pts',(-38.7517105593331,36.8920854300305,40.2639486641986));
#27103=CARTESIAN_POINT('Ctrl Pts',(-38.8201741811244,36.9684582081863,40.3477080184737));
#27104=CARTESIAN_POINT('Ctrl Pts',(-38.8865793070816,37.0491269119063,40.4292325426895));
#27105=CARTESIAN_POINT('Ctrl Pts',(-38.9507167264873,37.133837384107,40.5082653986073));
#27106=CARTESIAN_POINT('Ctrl Pts',(-34.9743855755961,36.8426418770279,35.9877612574109));
#27107=CARTESIAN_POINT('Ctrl Pts',(-35.0481880902205,36.7666600782349,36.0712653535917));
#27108=CARTESIAN_POINT('Ctrl Pts',(-35.123885349332,36.6951865080667,36.1571934070156));
#27109=CARTESIAN_POINT('Ctrl Pts',(-35.2012299269113,36.6284543820813,36.2452645362456));
#27110=CARTESIAN_POINT('Ctrl Pts',(-35.2785058260965,36.5617815111257,36.3332574624016));
#27111=CARTESIAN_POINT('Ctrl Pts',(-35.35742600984,36.4998417620662,36.4233895351976));
#27112=CARTESIAN_POINT('Ctrl Pts',(-35.4377330067502,36.4428368630046,36.5153666938478));
#27113=CARTESIAN_POINT('Ctrl Pts',(-35.5180400036605,36.3858319639429,36.6073438524981));
#27114=CARTESIAN_POINT('Ctrl Pts',(-35.5997336997324,36.3337619955086,36.7011659664208));
#27115=CARTESIAN_POINT('Ctrl Pts',(-35.6825475983504,36.2867965062328,36.7965269652247));
#27116=CARTESIAN_POINT('Ctrl Pts',(-35.7653614969684,36.239831016957,36.8918879640286));
#27117=CARTESIAN_POINT('Ctrl Pts',(-35.8492954805879,36.1979700732353,36.9887877123526));
#27118=CARTESIAN_POINT('Ctrl Pts',(-35.9340757647227,36.1613499408784,37.0869101256075));
#27119=CARTESIAN_POINT('Ctrl Pts',(-36.0188560488575,36.1247298085214,37.1850325388624));
#27120=CARTESIAN_POINT('Ctrl Pts',(-36.1044825131889,36.0933505392597,37.2843774777892));
#27121=CARTESIAN_POINT('Ctrl Pts',(-36.1906758700819,36.0673142298672,37.3846209041141));
#27122=CARTESIAN_POINT('Ctrl Pts',(-36.276869226975,36.0412779204747,37.4848643304389));
#27123=CARTESIAN_POINT('Ctrl Pts',(-36.3636293541202,36.0205846076808,37.5860061019117));
#27124=CARTESIAN_POINT('Ctrl Pts',(-36.4506732812072,36.0053015554969,37.6877163387799));
#27125=CARTESIAN_POINT('Ctrl Pts',(-36.5377172082942,35.9900185033129,37.7894265756482));
#27126=CARTESIAN_POINT('Ctrl Pts',(-36.6250448118189,35.9801457332289,37.8917051335964));
#27127=CARTESIAN_POINT('Ctrl Pts',(-36.7123712831683,35.9757152396661,37.9942184415413));
#27128=CARTESIAN_POINT('Ctrl Pts',(-36.7996977545177,35.9712847461032,38.0967317494861));
#27129=CARTESIAN_POINT('Ctrl Pts',(-36.8870229697971,35.9722965351728,38.199479661986));
#27130=CARTESIAN_POINT('Ctrl Pts',(-36.9740621383579,35.978747124609,38.3021270907198));
#27131=CARTESIAN_POINT('Ctrl Pts',(-37.0611013069187,35.9851977140451,38.4047745194536));
#27132=CARTESIAN_POINT('Ctrl Pts',(-37.147854305282,35.9970870945416,38.5073213188002));
#27133=CARTESIAN_POINT('Ctrl Pts',(-37.2340382168427,36.0143763311173,38.6094330670883));
#27134=CARTESIAN_POINT('Ctrl Pts',(-37.3202221284034,36.0316655676929,38.7115448153763));
#27135=CARTESIAN_POINT('Ctrl Pts',(-37.405836830902,36.054354635685,38.8132213677531));
#27136=CARTESIAN_POINT('Ctrl Pts',(-37.4906031255867,36.0823694022728,38.914131148664));
#27137=CARTESIAN_POINT('Ctrl Pts',(-37.5753694202713,36.1103841688607,39.0150409295749));
#27138=CARTESIAN_POINT('Ctrl Pts',(-37.6592871868977,36.1437245941859,39.1151837958783));
#27139=CARTESIAN_POINT('Ctrl Pts',(-37.7420827641078,36.1822818317011,39.2142331789989));
#27140=CARTESIAN_POINT('Ctrl Pts',(-37.8248783413179,36.2208390692164,39.3132825621194));
#27141=CARTESIAN_POINT('Ctrl Pts',(-37.906551611665,36.2646130641274,39.4112383215582));
#27142=CARTESIAN_POINT('Ctrl Pts',(-37.9868362346136,36.3134609663522,39.5077810239121));
#27143=CARTESIAN_POINT('Ctrl Pts',(-38.0671208575622,36.362308868577,39.604323726266));
#27144=CARTESIAN_POINT('Ctrl Pts',(-38.1460167192277,36.4162306087426,39.6994532345935));
#27145=CARTESIAN_POINT('Ctrl Pts',(-38.2232665356069,36.475050264875,39.7928593323378));
#27146=CARTESIAN_POINT('Ctrl Pts',(-38.300516351986,36.5338699210074,39.886265430082));
#27147=CARTESIAN_POINT('Ctrl Pts',(-38.3761200134976,36.5975874096069,39.9779479847499));
#27148=CARTESIAN_POINT('Ctrl Pts',(-38.4498309693652,36.6659948838339,40.0676080182377));
#27149=CARTESIAN_POINT('Ctrl Pts',(-38.5235419252329,36.7344023580609,40.1572680517256));
#27150=CARTESIAN_POINT('Ctrl Pts',(-38.5953600708919,36.8074997208323,40.2449054368509));
#27151=CARTESIAN_POINT('Ctrl Pts',(-38.6650511955598,36.8850485553831,40.3302343823459));
#27152=CARTESIAN_POINT('Ctrl Pts',(-38.7347423202279,36.9625973899338,40.415563327841));
#27153=CARTESIAN_POINT('Ctrl Pts',(-38.8023063250372,37.0445975862294,40.4985837126617));
#27154=CARTESIAN_POINT('Ctrl Pts',(-38.8675228655817,37.1307817116115,40.5790247948543));
#27155=CARTESIAN_POINT('Ctrl Pts',(-34.8336193643568,36.9033396115506,35.9904016908844));
#27156=CARTESIAN_POINT('Ctrl Pts',(-34.9075633574833,36.8235846665107,36.0739295021119));
#27157=CARTESIAN_POINT('Ctrl Pts',(-34.9835346561969,36.7484189640353,36.1600443950741));
#27158=CARTESIAN_POINT('Ctrl Pts',(-35.0612763540517,36.6780966665432,36.2484551606249));
#27159=CARTESIAN_POINT('Ctrl Pts',(-35.138949020888,36.6078368119867,36.3367874215202));
#27160=CARTESIAN_POINT('Ctrl Pts',(-35.2183888259916,36.542411871719,36.4274113451302));
#27161=CARTESIAN_POINT('Ctrl Pts',(-35.2993276161375,36.4820426910545,36.5200210256517));
#27162=CARTESIAN_POINT('Ctrl Pts',(-35.3802664062833,36.4216735103901,36.6126307061731));
#27163=CARTESIAN_POINT('Ctrl Pts',(-35.4627040582955,36.3663601812011,36.707226002669));
#27164=CARTESIAN_POINT('Ctrl Pts',(-35.5463622995597,36.3162894165289,36.8034876037588));
#27165=CARTESIAN_POINT('Ctrl Pts',(-35.630020540824,36.2662186518567,36.8997492048486));
#27166=CARTESIAN_POINT('Ctrl Pts',(-35.7148992440258,36.2213905279009,36.9976769640377));
#27167=CARTESIAN_POINT('Ctrl Pts',(-35.8007118966545,36.1819563643431,37.096940321043));
#27168=CARTESIAN_POINT('Ctrl Pts',(-35.8865245492833,36.1425222007853,37.1962036780483));
#27169=CARTESIAN_POINT('Ctrl Pts',(-35.9732710207459,36.108482057638,37.2968024818071));
#27170=CARTESIAN_POINT('Ctrl Pts',(-36.0606584937822,36.0799508391881,37.3983971557854));
#27171=CARTESIAN_POINT('Ctrl Pts',(-36.1480459668184,36.0514196207383,37.4999918297637));
#27172=CARTESIAN_POINT('Ctrl Pts',(-36.2360743084386,36.0283973704059,37.6025822193508));
#27173=CARTESIAN_POINT('Ctrl Pts',(-36.3244463743625,36.0109618010034,37.7058220253105));
#27174=CARTESIAN_POINT('Ctrl Pts',(-36.4128184402864,35.9935262316009,37.8090618312702));
#27175=CARTESIAN_POINT('Ctrl Pts',(-36.5015340960261,35.9816773696623,37.9129508964882));
#27176=CARTESIAN_POINT('Ctrl Pts',(-36.5902938772363,35.9754552116421,38.0171385379805));
#27177=CARTESIAN_POINT('Ctrl Pts',(-36.6790536584466,35.9692330536221,38.1213261794728));
#27178=CARTESIAN_POINT('Ctrl Pts',(-36.7678574300494,35.9686376089895,38.2258122386827));
#27179=CARTESIAN_POINT('Ctrl Pts',(-36.8564054302601,35.9736708876989,38.3302440174417));
#27180=CARTESIAN_POINT('Ctrl Pts',(-36.9449534304708,35.9787041664084,38.4346757962008));
#27181=CARTESIAN_POINT('Ctrl Pts',(-37.0332455245334,35.9893661608002,38.5390531355806));
#27182=CARTESIAN_POINT('Ctrl Pts',(-37.1209836778578,36.0056208807534,38.6430237044025));
#27183=CARTESIAN_POINT('Ctrl Pts',(-37.2087218311821,36.0218756007066,38.7469942732243));
#27184=CARTESIAN_POINT('Ctrl Pts',(-37.2959059102448,36.0437230214842,38.8505579132615));
#27185=CARTESIAN_POINT('Ctrl Pts',(-37.382241620618,36.0710893959725,38.9533650400202));
#27186=CARTESIAN_POINT('Ctrl Pts',(-37.4685773309913,36.0984557704607,39.0561721667788));
#27187=CARTESIAN_POINT('Ctrl Pts',(-37.5540645412861,36.1313410570124,39.1582226238029));
#27188=CARTESIAN_POINT('Ctrl Pts',(-37.6384146849442,36.1696342496195,39.2591719344269));
#27189=CARTESIAN_POINT('Ctrl Pts',(-37.7227648286024,36.2079274422265,39.3601212450509));
#27190=CARTESIAN_POINT('Ctrl Pts',(-37.8059777772566,36.2516284826128,39.4599692556463));
#27191=CARTESIAN_POINT('Ctrl Pts',(-37.8877726412378,36.3005898556264,39.5583789240207));
#27192=CARTESIAN_POINT('Ctrl Pts',(-37.969567505219,36.3495512286401,39.6567885923951));
#27193=CARTESIAN_POINT('Ctrl Pts',(-38.0499441600487,36.4037728597698,39.7537597687849));
#27194=CARTESIAN_POINT('Ctrl Pts',(-38.1286312901165,36.4630717210582,39.8489651219026));
#27195=CARTESIAN_POINT('Ctrl Pts',(-38.2073184201842,36.5223705823465,39.9441704750202));
#27196=CARTESIAN_POINT('Ctrl Pts',(-38.2843159057409,36.5867465835503,40.0376098599784));
#27197=CARTESIAN_POINT('Ctrl Pts',(-38.3593638377389,36.6559824201038,40.1289678672367));
#27198=CARTESIAN_POINT('Ctrl Pts',(-38.434411769737,36.7252182566573,40.2203258744951));
#27199=CARTESIAN_POINT('Ctrl Pts',(-38.5075100339655,36.7993138231947,40.3096023650212));
#27200=CARTESIAN_POINT('Ctrl Pts',(-38.5784118834031,36.8780190062483,40.3964959813431));
#27201=CARTESIAN_POINT('Ctrl Pts',(-38.6493137328406,36.9567241893019,40.4833895976649));
#27202=CARTESIAN_POINT('Ctrl Pts',(-38.718019059586,37.0400388690951,40.5679002075443));
#27203=CARTESIAN_POINT('Ctrl Pts',(-38.7842959452082,37.1276818125601,40.6497425409889));
#27204=CARTESIAN_POINT('Ctrl Pts',(-34.6928531531176,36.9640373460733,35.993042124358));
#27205=CARTESIAN_POINT('Ctrl Pts',(-34.7669386247461,36.8805092547864,36.0765936506321));
#27206=CARTESIAN_POINT('Ctrl Pts',(-34.8431839630618,36.8016514200038,36.1628953831327));
#27207=CARTESIAN_POINT('Ctrl Pts',(-34.9213227811921,36.7277389510052,36.2516457850041));
#27208=CARTESIAN_POINT('Ctrl Pts',(-34.9993922156795,36.6538921128476,36.3403173806389));
#27209=CARTESIAN_POINT('Ctrl Pts',(-35.0793516421433,36.5849819813717,36.4314331550628));
#27210=CARTESIAN_POINT('Ctrl Pts',(-35.1609222255247,36.5212485191045,36.5246753574555));
#27211=CARTESIAN_POINT('Ctrl Pts',(-35.242492808906,36.4575150568373,36.6179175598482));
#27212=CARTESIAN_POINT('Ctrl Pts',(-35.3256744168587,36.3989583668936,36.7132860389173));
#27213=CARTESIAN_POINT('Ctrl Pts',(-35.4101770007691,36.345782326825,36.810448242293));
#27214=CARTESIAN_POINT('Ctrl Pts',(-35.4946795846796,36.2926062867564,36.9076104456687));
#27215=CARTESIAN_POINT('Ctrl Pts',(-35.5805030074637,36.2448109825665,37.0065662157227));
#27216=CARTESIAN_POINT('Ctrl Pts',(-35.6673480285863,36.2025627878079,37.1069705164784));
#27217=CARTESIAN_POINT('Ctrl Pts',(-35.7541930497091,36.1603145930492,37.2073748172342));
#27218=CARTESIAN_POINT('Ctrl Pts',(-35.842059528303,36.1236135760163,37.309227485825));
#27219=CARTESIAN_POINT('Ctrl Pts',(-35.9306411174824,36.0925874485091,37.4121734074567));
#27220=CARTESIAN_POINT('Ctrl Pts',(-36.0192227066619,36.0615613210019,37.5151193290884));
#27221=CARTESIAN_POINT('Ctrl Pts',(-36.108519262757,36.036210133131,37.61915833679));
#27222=CARTESIAN_POINT('Ctrl Pts',(-36.1982194675179,36.0166220465098,37.7239277118411));
#27223=CARTESIAN_POINT('Ctrl Pts',(-36.2879196722787,35.9970339598887,37.8286970868923));
#27224=CARTESIAN_POINT('Ctrl Pts',(-36.3780233802332,35.9832090060956,37.93419665938));
#27225=CARTESIAN_POINT('Ctrl Pts',(-36.4682164713043,35.9751951836183,38.0400586344198));
#27226=CARTESIAN_POINT('Ctrl Pts',(-36.5584095623755,35.9671813611409,38.1459206094595));
#27227=CARTESIAN_POINT('Ctrl Pts',(-36.6486918903018,35.9649786828061,38.2521448153794));
#27228=CARTESIAN_POINT('Ctrl Pts',(-36.7387487221623,35.968594650789,38.3583609441637));
#27229=CARTESIAN_POINT('Ctrl Pts',(-36.8288055540228,35.9722106187718,38.464577072948));
#27230=CARTESIAN_POINT('Ctrl Pts',(-36.9186367437849,35.9816452270589,38.5707849523611));
#27231=CARTESIAN_POINT('Ctrl Pts',(-37.0079291388729,35.9968654303896,38.6766143417166));
#27232=CARTESIAN_POINT('Ctrl Pts',(-37.0972215339608,36.0120856337203,38.7824437310722));
#27233=CARTESIAN_POINT('Ctrl Pts',(-37.1859749895875,36.0330914072835,38.88789445877));
#27234=CARTESIAN_POINT('Ctrl Pts',(-37.2738801156494,36.0598093896721,38.9925989313764));
#27235=CARTESIAN_POINT('Ctrl Pts',(-37.3617852417113,36.0865273720607,39.0973034039828));
#27236=CARTESIAN_POINT('Ctrl Pts',(-37.4488418956745,36.118957519839,39.2012614517275));
#27237=CARTESIAN_POINT('Ctrl Pts',(-37.5347466057807,36.1569866675378,39.304110689855));
#27238=CARTESIAN_POINT('Ctrl Pts',(-37.6206513158869,36.1950158152366,39.4069599279825));
#27239=CARTESIAN_POINT('Ctrl Pts',(-37.705403942848,36.2386439010982,39.5087001897343));
#27240=CARTESIAN_POINT('Ctrl Pts',(-37.7887090478619,36.2877187449007,39.6089768241292));
#27241=CARTESIAN_POINT('Ctrl Pts',(-37.8720141528758,36.3367935887032,39.7092534585241));
#27242=CARTESIAN_POINT('Ctrl Pts',(-37.9538716008697,36.391315110797,39.8080663029763));
#27243=CARTESIAN_POINT('Ctrl Pts',(-38.0339960446261,36.4510931772414,39.9050709114673));
#27244=CARTESIAN_POINT('Ctrl Pts',(-38.1141204883824,36.5108712436857,40.0020755199584));
#27245=CARTESIAN_POINT('Ctrl Pts',(-38.1925117979841,36.5759057574937,40.097271735207));
#27246=CARTESIAN_POINT('Ctrl Pts',(-38.2688967061126,36.6459699563737,40.1903277162358));
#27247=CARTESIAN_POINT('Ctrl Pts',(-38.3452816142411,36.7160341552536,40.2833836972645));
#27248=CARTESIAN_POINT('Ctrl Pts',(-38.4196599970392,36.7911279255571,40.3742992931915));
#27249=CARTESIAN_POINT('Ctrl Pts',(-38.4917725712463,36.8709894571135,40.4627575803402));
#27250=CARTESIAN_POINT('Ctrl Pts',(-38.5638851454534,36.9508509886701,40.5512158674888));
#27251=CARTESIAN_POINT('Ctrl Pts',(-38.6337317941347,37.0354801519608,40.6372167024268));
#27252=CARTESIAN_POINT('Ctrl Pts',(-38.7010690248348,37.1245819135087,40.7204602871234));
#27253=CARTESIAN_POINT('Ctrl Pts',(-34.5541602432366,37.0269902948154,35.9977665285712));
#27254=CARTESIAN_POINT('Ctrl Pts',(-34.6282792954805,36.9396621033914,36.0812119484611));
#27255=CARTESIAN_POINT('Ctrl Pts',(-34.7046959128131,36.8570776877087,36.1675772839025));
#27256=CARTESIAN_POINT('Ctrl Pts',(-34.7831343550503,36.7795345937814,36.2565508787775));
#27257=CARTESIAN_POINT('Ctrl Pts',(-34.8615031475922,36.7020603545216,36.3454454692308));
#27258=CARTESIAN_POINT('Ctrl Pts',(-34.9418900404055,36.6296186217796,36.4369435352596));
#27259=CARTESIAN_POINT('Ctrl Pts',(-35.0240055191768,36.5624699166282,36.5307155327172));
#27260=CARTESIAN_POINT('Ctrl Pts',(-35.1061209979481,36.4953212114768,36.6244875301747));
#27261=CARTESIAN_POINT('Ctrl Pts',(-35.1899649205664,36.4334656497696,36.7205332967659));
#27262=CARTESIAN_POINT('Ctrl Pts',(-35.2752353489086,36.3771256469852,36.818506943316));
#27263=CARTESIAN_POINT('Ctrl Pts',(-35.3605057772508,36.3207856442009,36.9164805898661));
#27264=CARTESIAN_POINT('Ctrl Pts',(-35.4472025637708,36.2699612975081,37.0163819468398));
#27265=CARTESIAN_POINT('Ctrl Pts',(-35.5350135199691,36.2248353183834,37.1178512699157));
#27266=CARTESIAN_POINT('Ctrl Pts',(-35.6228244761675,36.1797093392588,37.2193205929915));
#27267=CARTESIAN_POINT('Ctrl Pts',(-35.7117494501238,36.1402818054887,37.322357706613));
#27268=CARTESIAN_POINT('Ctrl Pts',(-35.8014682500023,36.106694411774,37.4265916006991));
#27269=CARTESIAN_POINT('Ctrl Pts',(-35.8911870498807,36.0731070180593,37.5308254947853));
#27270=CARTESIAN_POINT('Ctrl Pts',(-35.9816995204786,36.0453598222465,37.6362559890205));
#27271=CARTESIAN_POINT('Ctrl Pts',(-36.0726797711134,36.0235524845427,37.7425034778403));
#27272=CARTESIAN_POINT('Ctrl Pts',(-36.1636600217483,36.0017451468388,37.8487509666601));
#27273=CARTESIAN_POINT('Ctrl Pts',(-36.255107895051,35.9858777047353,37.9558152662862));
#27274=CARTESIAN_POINT('Ctrl Pts',(-36.3466941468655,35.9760070685835,38.0633109076383));
#27275=CARTESIAN_POINT('Ctrl Pts',(-36.4382803986801,35.9661364324317,38.1708065489904));
#27276=CARTESIAN_POINT('Ctrl Pts',(-36.5300048706022,35.9622626190992,38.2787333461486));
#27277=CARTESIAN_POINT('Ctrl Pts',(-36.6215373343988,35.9643993812032,38.3867027405372));
#27278=CARTESIAN_POINT('Ctrl Pts',(-36.7130697981954,35.9665361433072,38.4946721349258));
#27279=CARTESIAN_POINT('Ctrl Pts',(-36.8044100955656,35.9746834769709,38.6026839398195));
#27280=CARTESIAN_POINT('Ctrl Pts',(-36.8952293905873,35.9888118796016,38.7103493032797));
#27281=CARTESIAN_POINT('Ctrl Pts',(-36.9860486856089,36.0029402822323,38.8180146667399));
#27282=CARTESIAN_POINT('Ctrl Pts',(-37.0763468212224,36.0230497292377,38.9253334025781));
#27283=CARTESIAN_POINT('Ctrl Pts',(-37.1657987201138,36.0490676764313,39.0319191636385));
#27284=CARTESIAN_POINT('Ctrl Pts',(-37.2552506190054,36.0750856236247,39.138504924699));
#27285=CARTESIAN_POINT('Ctrl Pts',(-37.3438561264855,36.1070120258759,39.2443575266683));
#27286=CARTESIAN_POINT('Ctrl Pts',(-37.4312962630486,36.1447318205671,39.3490959072212));
#27287=CARTESIAN_POINT('Ctrl Pts',(-37.5187363996116,36.1824516152582,39.453834287774));
#27288=CARTESIAN_POINT('Ctrl Pts',(-37.6050110140502,36.2259647370456,39.5574582657969));
#27289=CARTESIAN_POINT('Ctrl Pts',(-37.6898095199542,36.2751144338207,39.6595948057618));
#27290=CARTESIAN_POINT('Ctrl Pts',(-37.7746080258582,36.3242641305957,39.7617313457267));
#27291=CARTESIAN_POINT('Ctrl Pts',(-37.857930276589,36.3790503172715,39.8623802710219));
#27292=CARTESIAN_POINT('Ctrl Pts',(-37.9394763137113,36.4392756810004,39.9611792570969));
#27293=CARTESIAN_POINT('Ctrl Pts',(-38.0210223508336,36.4995010447292,40.0599782431719));
#27294=CARTESIAN_POINT('Ctrl Pts',(-38.1007920333314,36.565165481293,40.1569271191858));
#27295=CARTESIAN_POINT('Ctrl Pts',(-38.178498189151,36.6360325375495,40.2516768786658));
#27296=CARTESIAN_POINT('Ctrl Pts',(-38.2562043449706,36.706899593806,40.3464266381459));
#27297=CARTESIAN_POINT('Ctrl Pts',(-38.3318468397324,36.7829691471553,40.4389771172502));
#27298=CARTESIAN_POINT('Ctrl Pts',(-38.4051533541858,36.8639673060839,40.5289951388672));
#27299=CARTESIAN_POINT('Ctrl Pts',(-38.4784598686392,36.9449654650124,40.6190131604841));
#27300=CARTESIAN_POINT('Ctrl Pts',(-38.5494302760069,37.0308920894196,40.7064985689482));
#27301=CARTESIAN_POINT('Ctrl Pts',(-38.6178090694252,37.121437820586,40.7911364139259));
#27302=CARTESIAN_POINT('Ctrl Pts',(-34.4174636369452,37.0920493708544,36.0044534955695));
#27303=CARTESIAN_POINT('Ctrl Pts',(-34.4915103886568,37.0009023997844,36.0876630582019));
#27304=CARTESIAN_POINT('Ctrl Pts',(-34.5679972742404,36.9145644290366,36.1739686895439));
#27305=CARTESIAN_POINT('Ctrl Pts',(-34.6466394145708,36.8333570035688,36.263048938941));
#27306=CARTESIAN_POINT('Ctrl Pts',(-34.7252117243315,36.7522216865249,36.3520500892121));
#27307=CARTESIAN_POINT('Ctrl Pts',(-34.8059353179264,36.6762079572462,36.443820767926));
#27308=CARTESIAN_POINT('Ctrl Pts',(-34.8885100776198,36.6055984229273,36.5380197860067));
#27309=CARTESIAN_POINT('Ctrl Pts',(-34.9710848373132,36.5349888886083,36.6322188040875));
#27310=CARTESIAN_POINT('Ctrl Pts',(-35.0555106106353,36.4697836796259,36.7288459876017));
#27311=CARTESIAN_POINT('Ctrl Pts',(-35.1414735157231,36.4102252187812,36.8275420917456));
#27312=CARTESIAN_POINT('Ctrl Pts',(-35.2274364208109,36.3506667579364,36.9262381958896));
#27313=CARTESIAN_POINT('Ctrl Pts',(-35.3149362989387,36.2967551552008,37.0270030384264));
#27314=CARTESIAN_POINT('Ctrl Pts',(-35.4036478392012,36.2486908455082,37.129461991381));
#27315=CARTESIAN_POINT('Ctrl Pts',(-35.4923593794637,36.2006265358157,37.2319209443357));
#27316=CARTESIAN_POINT('Ctrl Pts',(-35.5822824180598,36.1584096079143,37.3360738185234));
#27317=CARTESIAN_POINT('Ctrl Pts',(-35.6730826351516,36.1221970177602,37.4415333897958));
#27318=CARTESIAN_POINT('Ctrl Pts',(-35.7638828522433,36.0859844276062,37.5469929610681));
#27319=CARTESIAN_POINT('Ctrl Pts',(-35.855560080173,36.055776242064,37.6537590346999));
#27320=CARTESIAN_POINT('Ctrl Pts',(-35.9477734773,36.0316847704579,37.7614346710745));
#27321=CARTESIAN_POINT('Ctrl Pts',(-36.039986874427,36.0075932988519,37.8691103074492));
#27322=CARTESIAN_POINT('Ctrl Pts',(-36.1327362704844,35.9896185856657,37.9776953077495));
#27323=CARTESIAN_POINT('Ctrl Pts',(-36.2256768376776,35.9778274580804,38.0867859698732));
#27324=CARTESIAN_POINT('Ctrl Pts',(-36.3186174048707,35.9660363304952,38.195876631997));
#27325=CARTESIAN_POINT('Ctrl Pts',(-36.4117489715901,35.9604288102826,38.3054727545143));
#27326=CARTESIAN_POINT('Ctrl Pts',(-36.5047252891902,35.9610257453286,38.415166876128));
#27327=CARTESIAN_POINT('Ctrl Pts',(-36.5977016067903,35.9616226803746,38.5248609977418));
#27328=CARTESIAN_POINT('Ctrl Pts',(-36.6905225035954,35.9684240695771,38.6346529159078));
#27329=CARTESIAN_POINT('Ctrl Pts',(-36.7828428859823,35.9814046264313,38.7441344413914));
#27330=CARTESIAN_POINT('Ctrl Pts',(-36.8751632683692,35.9943851832855,38.853615966875));
#27331=CARTESIAN_POINT('Ctrl Pts',(-36.9669829658735,36.0135448838234,38.9627868975245));
#27332=CARTESIAN_POINT('Ctrl Pts',(-37.0579606071748,36.0388124952658,39.0712413528399));
#27333=CARTESIAN_POINT('Ctrl Pts',(-37.1489382484762,36.0640801067081,39.1796958081554));
#27334=CARTESIAN_POINT('Ctrl Pts',(-37.2390736655894,36.0954555823994,39.2874335878816));
#27335=CARTESIAN_POINT('Ctrl Pts',(-37.3280317490861,36.1328222732128,39.3940541397503));
#27336=CARTESIAN_POINT('Ctrl Pts',(-37.4169898325828,36.1701889640262,39.500674691619));
#27337=CARTESIAN_POINT('Ctrl Pts',(-37.5047704182067,36.2135468009659,39.6061778187612));
#27338=CARTESIAN_POINT('Ctrl Pts',(-37.5910471514259,36.2627345863541,39.7101712769985));
#27339=CARTESIAN_POINT('Ctrl Pts',(-37.6773238846452,36.3119223717422,39.8141647352358));
#27340=CARTESIAN_POINT('Ctrl Pts',(-37.7620966061544,36.3669400147562,39.91664833255));
#27341=CARTESIAN_POINT('Ctrl Pts',(-37.8450501441915,36.4275829683767,40.0172410509039));
#27342=CARTESIAN_POINT('Ctrl Pts',(-37.9280036822286,36.4882259219973,40.1178337692578));
#27343=CARTESIAN_POINT('Ctrl Pts',(-38.0091378836244,36.5544940742505,40.2165354229125));
#27344=CARTESIAN_POINT('Ctrl Pts',(-38.0881511040673,36.6261410504777,40.3129790545077));
#27345=CARTESIAN_POINT('Ctrl Pts',(-38.1671643245102,36.697788026705,40.4094226861029));
#27346=CARTESIAN_POINT('Ctrl Pts',(-38.2440564181065,36.7748136946141,40.5036081175607));
#27347=CARTESIAN_POINT('Ctrl Pts',(-38.3185415120401,36.8569316847805,40.5951851821307));
#27348=CARTESIAN_POINT('Ctrl Pts',(-38.3930266059737,36.9390496749468,40.6867622467008));
#27349=CARTESIAN_POINT('Ctrl Pts',(-38.465104562712,37.026259835744,40.7757307752912));
#27350=CARTESIAN_POINT('Ctrl Pts',(-38.5345074076489,37.1182379333905,40.8617599967831));
#27351=CARTESIAN_POINT('Ctrl Pts',(-34.2807670306538,37.1571084468935,36.0111404625678));
#27352=CARTESIAN_POINT('Ctrl Pts',(-34.3547414818331,37.0621426961774,36.0941141679427));
#27353=CARTESIAN_POINT('Ctrl Pts',(-34.4312986356677,36.9720511703645,36.1803600951854));
#27354=CARTESIAN_POINT('Ctrl Pts',(-34.5101444740912,36.8871794133564,36.2695469991044));
#27355=CARTESIAN_POINT('Ctrl Pts',(-34.5889203010707,36.8023830185282,36.3586547091934));
#27356=CARTESIAN_POINT('Ctrl Pts',(-34.6699805954473,36.7227972927127,36.4506980005925));
#27357=CARTESIAN_POINT('Ctrl Pts',(-34.7530146360628,36.6487269292264,36.5453240392963));
#27358=CARTESIAN_POINT('Ctrl Pts',(-34.8360486766783,36.5746565657399,36.6399500780003));
#27359=CARTESIAN_POINT('Ctrl Pts',(-34.9210563007041,36.5061017094822,36.7371586784375));
#27360=CARTESIAN_POINT('Ctrl Pts',(-35.0077116825375,36.4433247905771,36.8365772401753));
#27361=CARTESIAN_POINT('Ctrl Pts',(-35.0943670643709,36.3805478716719,36.9359958019131));
#27362=CARTESIAN_POINT('Ctrl Pts',(-35.1826700341066,36.3235490128934,37.0376241300129));
#27363=CARTESIAN_POINT('Ctrl Pts',(-35.2722821584332,36.272546372633,37.1410727128464));
#27364=CARTESIAN_POINT('Ctrl Pts',(-35.3618942827598,36.2215437323726,37.2445212956798));
#27365=CARTESIAN_POINT('Ctrl Pts',(-35.4528153859958,36.1765374103399,37.3497899304337));
#27366=CARTESIAN_POINT('Ctrl Pts',(-35.5446970203009,36.1376996237464,37.4564751788924));
#27367=CARTESIAN_POINT('Ctrl Pts',(-35.6365786546059,36.0988618371529,37.563160427351));
#27368=CARTESIAN_POINT('Ctrl Pts',(-35.7294206398673,36.0661926618815,37.6712620803793));
#27369=CARTESIAN_POINT('Ctrl Pts',(-35.8228671834865,36.0398170563733,37.7803658643088));
#27370=CARTESIAN_POINT('Ctrl Pts',(-35.9163137271057,36.013441450865,37.8894696482382));
#27371=CARTESIAN_POINT('Ctrl Pts',(-36.0103646459177,35.993359466596,37.9995753492128));
#27372=CARTESIAN_POINT('Ctrl Pts',(-36.1046595284896,35.9796478475772,38.1102610321082));
#27373=CARTESIAN_POINT('Ctrl Pts',(-36.1989544110615,35.9659362285585,38.2209467150036));
#27374=CARTESIAN_POINT('Ctrl Pts',(-36.2934930725781,35.9585950014659,38.3322121628799));
#27375=CARTESIAN_POINT('Ctrl Pts',(-36.3879132439816,35.957652109454,38.4436310117189));
#27376=CARTESIAN_POINT('Ctrl Pts',(-36.4823334153852,35.9567092174422,38.5550498605578));
#27377=CARTESIAN_POINT('Ctrl Pts',(-36.5766349116251,35.9621646621833,38.6666218919961));
#27378=CARTESIAN_POINT('Ctrl Pts',(-36.6704563813773,35.973997373261,38.7779195795031));
#27379=CARTESIAN_POINT('Ctrl Pts',(-36.7642778511296,35.9858300843386,38.8892172670101));
#27380=CARTESIAN_POINT('Ctrl Pts',(-36.8576191105247,36.0040400384092,39.0002403924709));
#27381=CARTESIAN_POINT('Ctrl Pts',(-36.9501224942359,36.0285573141003,39.1105635420414));
#27382=CARTESIAN_POINT('Ctrl Pts',(-37.042625877947,36.0530745897914,39.2208866916118));
#27383=CARTESIAN_POINT('Ctrl Pts',(-37.1342912046932,36.083899138923,39.3305096490948));
#27384=CARTESIAN_POINT('Ctrl Pts',(-37.2247672351236,36.1209127258585,39.4390123722794));
#27385=CARTESIAN_POINT('Ctrl Pts',(-37.3152432655539,36.1579263127941,39.547515095464));
#27386=CARTESIAN_POINT('Ctrl Pts',(-37.4045298223632,36.2011288648863,39.6548973717255));
#27387=CARTESIAN_POINT('Ctrl Pts',(-37.4922847828977,36.2503547388875,39.7607477482352));
#27388=CARTESIAN_POINT('Ctrl Pts',(-37.5800397434322,36.2995806128888,39.8665981247448));
#27389=CARTESIAN_POINT('Ctrl Pts',(-37.6662629357198,36.3548297122409,39.9709163940781));
#27390=CARTESIAN_POINT('Ctrl Pts',(-37.7506239746718,36.4158902557531,40.0733028447109));
#27391=CARTESIAN_POINT('Ctrl Pts',(-37.8349850136237,36.4769507992654,40.1756892953438));
#27392=CARTESIAN_POINT('Ctrl Pts',(-37.9174837339175,36.543822667208,40.2761437266394));
#27393=CARTESIAN_POINT('Ctrl Pts',(-37.9978040189836,36.616249563406,40.3742812303496));
#27394=CARTESIAN_POINT('Ctrl Pts',(-38.0781243040497,36.688676459604,40.4724187340598));
#27395=CARTESIAN_POINT('Ctrl Pts',(-38.1562659964805,36.766658242073,40.5682391178711));
#27396=CARTESIAN_POINT('Ctrl Pts',(-38.2319296698944,36.8498960634771,40.6613752253943));
#27397=CARTESIAN_POINT('Ctrl Pts',(-38.3075933433082,36.9331338848813,40.7545113329175));
#27398=CARTESIAN_POINT('Ctrl Pts',(-38.3807788494171,37.0216275820683,40.8449629816342));
#27399=CARTESIAN_POINT('Ctrl Pts',(-38.4512057458726,37.115038046195,40.9323835796403));
#27400=CARTESIAN_POINT('Ctrl Pts',(-34.1460670485564,37.2242742219759,36.0197904648656));
#27401=CARTESIAN_POINT('Ctrl Pts',(-34.2198633028138,37.1254709932035,36.1023985558072));
#27402=CARTESIAN_POINT('Ctrl Pts',(-34.2963896997116,37.0315989199376,36.1884614659634));
#27403=CARTESIAN_POINT('Ctrl Pts',(-34.3753432965714,36.9430291072631,36.2776384801598));
#27404=CARTESIAN_POINT('Ctrl Pts',(-34.4542267863025,36.8545379404703,36.3667363093075));
#27405=CARTESIAN_POINT('Ctrl Pts',(-34.5355330030382,36.7713398060557,36.4589425288971));
#27406=CARTESIAN_POINT('Ctrl Pts',(-34.618940697983,36.6937630110328,36.5538928082319));
#27407=CARTESIAN_POINT('Ctrl Pts',(-34.7023483929277,36.61618621601,36.6488430875667));
#27408=CARTESIAN_POINT('Ctrl Pts',(-34.7878573922997,36.5442309215851,36.7465372288016));
#27409=CARTESIAN_POINT('Ctrl Pts',(-34.8751298724766,36.4781810345725,36.8465892569098));
#27410=CARTESIAN_POINT('Ctrl Pts',(-34.9624023526535,36.4121311475598,36.9466412850182));
#27411=CARTESIAN_POINT('Ctrl Pts',(-35.0514381318324,36.3519868051728,37.049050991565));
#27412=CARTESIAN_POINT('Ctrl Pts',(-35.1418854798034,36.2979852747439,37.153413805841));
#27413=CARTESIAN_POINT('Ctrl Pts',(-35.2323328277744,36.2439837443151,37.257776620117));
#27414=CARTESIAN_POINT('Ctrl Pts',(-35.3241915561479,36.1961251379842,37.3640923247422));
#27415=CARTESIAN_POINT('Ctrl Pts',(-35.4170988059786,36.1545982125046,37.4719409485585));
#27416=CARTESIAN_POINT('Ctrl Pts',(-35.5100060558093,36.1130712870252,37.5797895723749));
#27417=CARTESIAN_POINT('Ctrl Pts',(-35.6039616336074,36.0778761285799,37.6891708907723));
#27418=CARTESIAN_POINT('Ctrl Pts',(-35.6985944172415,36.04915149517,37.7996528487545));
#27419=CARTESIAN_POINT('Ctrl Pts',(-35.7932272008757,36.0204268617601,37.9101348067368));
#27420=CARTESIAN_POINT('Ctrl Pts',(-35.8885369932823,35.9981728129329,38.0217171742356));
#27421=CARTESIAN_POINT('Ctrl Pts',(-35.984147339783,35.9824770144079,38.1339592242373));
#27422=CARTESIAN_POINT('Ctrl Pts',(-36.0797576862837,35.9667812158829,38.2462012742389));
#27423=CARTESIAN_POINT('Ctrl Pts',(-36.1756683877955,35.9576437001034,38.3591027730317));
#27424=CARTESIAN_POINT('Ctrl Pts',(-36.2715006297025,35.9551003502302,38.4722178016998));
#27425=CARTESIAN_POINT('Ctrl Pts',(-36.3673328716094,35.9525570003569,38.5853328303679));
#27426=CARTESIAN_POINT('Ctrl Pts',(-36.4630864543794,35.9566078214742,38.6986611534001));
#27427=CARTESIAN_POINT('Ctrl Pts',(-36.5583831945893,35.9672366325882,38.811755180936));
#27428=CARTESIAN_POINT('Ctrl Pts',(-36.6536799347991,35.9778654437021,38.924849208472));
#27429=CARTESIAN_POINT('Ctrl Pts',(-36.7485196340419,35.9950722224986,39.0377087050586));
#27430=CARTESIAN_POINT('Ctrl Pts',(-36.8425277261441,36.0187888531204,39.1498879439181));
#27431=CARTESIAN_POINT('Ctrl Pts',(-36.9365358182464,36.0425054837423,39.2620671827775));
#27432=CARTESIAN_POINT('Ctrl Pts',(-37.0297121074911,36.0727319166539,39.3735659303718));
#27433=CARTESIAN_POINT('Ctrl Pts',(-37.1216886023854,36.1093486402811,39.4839438422258));
#27434=CARTESIAN_POINT('Ctrl Pts',(-37.2136650972797,36.1459653639082,39.5943217540799));
#27435=CARTESIAN_POINT('Ctrl Pts',(-37.3044416063403,36.1889723018853,39.703578600413));
#27436=CARTESIAN_POINT('Ctrl Pts',(-37.393659618231,36.2381994916581,39.8112828957086));
#27437=CARTESIAN_POINT('Ctrl Pts',(-37.4828776301218,36.2874266814309,39.9189871910042));
#27438=CARTESIAN_POINT('Ctrl Pts',(-37.5705369591035,36.342874020407,40.025138711051));
#27439=CARTESIAN_POINT('Ctrl Pts',(-37.6562914046025,36.4043224379193,40.1293182359613));
#27440=CARTESIAN_POINT('Ctrl Pts',(-37.7420458501015,36.4657708554316,40.2334977608714));
#27441=CARTESIAN_POINT('Ctrl Pts',(-37.8258952335875,36.5332202234704,40.3357050737716));
#27442=CARTESIAN_POINT('Ctrl Pts',(-37.9075083986571,36.6064040936536,40.4355365302169));
#27443=CARTESIAN_POINT('Ctrl Pts',(-37.9891215637268,36.6795879638368,40.5353679866623));
#27444=CARTESIAN_POINT('Ctrl Pts',(-38.0684983404671,36.7585061837471,40.632823378828));
#27445=CARTESIAN_POINT('Ctrl Pts',(-38.145325231296,36.8428470315601,40.7275178245671));
#27446=CARTESIAN_POINT('Ctrl Pts',(-38.222152122125,36.9271878793732,40.822212270306));
#27447=CARTESIAN_POINT('Ctrl Pts',(-38.2964289670869,37.0169511794669,40.914145572481));
#27448=CARTESIAN_POINT('Ctrl Pts',(-38.3678624026918,37.1117823981211,41.0029546500012));
#27449=CARTESIAN_POINT('Ctrl Pts',(-34.0133169793171,37.2934251222052,36.0303088752264));
#27450=CARTESIAN_POINT('Ctrl Pts',(-34.0868306484354,37.1907737376081,36.1124205074871));
#27451=CARTESIAN_POINT('Ctrl Pts',(-34.1632264785125,37.0931013004299,36.1981758655312));
#27452=CARTESIAN_POINT('Ctrl Pts',(-34.2421929094087,37.0008061104388,36.2872252173864));
#27453=CARTESIAN_POINT('Ctrl Pts',(-34.3210892217803,36.9085928742915,36.3761954975512));
#27454=CARTESIAN_POINT('Ctrl Pts',(-34.4025513971612,36.8217475442532,36.4684537273036));
#27455=CARTESIAN_POINT('Ctrl Pts',(-34.4862478133071,36.7406236567121,36.5636243350232));
#27456=CARTESIAN_POINT('Ctrl Pts',(-34.5699442294529,36.6594997691709,36.6587949427428));
#27457=CARTESIAN_POINT('Ctrl Pts',(-34.6558747010474,36.5840975037473,36.7568777177077));
#27458=CARTESIAN_POINT('Ctrl Pts',(-34.7436894159758,36.5147238135561,36.8574733773083));
#27459=CARTESIAN_POINT('Ctrl Pts',(-34.8315041309041,36.4453501233649,36.958069036909));
#27460=CARTESIAN_POINT('Ctrl Pts',(-34.9212028947314,36.3820051620099,37.0611773584116));
#27461=CARTESIAN_POINT('Ctrl Pts',(-35.0124205551003,36.3249467988416,37.1663786008404));
#27462=CARTESIAN_POINT('Ctrl Pts',(-35.1036382154692,36.2678884356732,37.2715798432691));
#27463=CARTESIAN_POINT('Ctrl Pts',(-35.1963745704102,36.2171167970273,37.3788737736927));
#27464=CARTESIAN_POINT('Ctrl Pts',(-35.2902521019156,36.1728385678428,37.4878236120493));
#27465=CARTESIAN_POINT('Ctrl Pts',(-35.3841296334209,36.1285603386583,37.5967734504059));
#27466=CARTESIAN_POINT('Ctrl Pts',(-35.4791481336318,36.0907756169739,37.7073789554642));
#27467=CARTESIAN_POINT('Ctrl Pts',(-35.5749207942147,36.0596382196272,37.8191898661595));
#27468=CARTESIAN_POINT('Ctrl Pts',(-35.6706934547976,36.0285008222805,37.9310007768548));
#27469=CARTESIAN_POINT('Ctrl Pts',(-35.7672200636977,36.0040108182144,38.0440168456211));
#27470=CARTESIAN_POINT('Ctrl Pts',(-35.8641076732612,35.9862679031475,38.1577779982926));
#27471=CARTESIAN_POINT('Ctrl Pts',(-35.9609952828248,35.9685249880804,38.2715391509643));
#27472=CARTESIAN_POINT('Ctrl Pts',(-36.0582436785282,35.9575292012981,38.386045135657));
#27473=CARTESIAN_POINT('Ctrl Pts',(-36.1554569744145,35.953325305262,38.5008298129453));
#27474=CARTESIAN_POINT('Ctrl Pts',(-36.252670270301,35.9491214092257,38.6156144902337));
#27475=CARTESIAN_POINT('Ctrl Pts',(-36.3498482511257,35.9517094132437,38.7306776059673));
#27476=CARTESIAN_POINT('Ctrl Pts',(-36.4465953175821,35.9610787818779,38.8455507527104));
#27477=CARTESIAN_POINT('Ctrl Pts',(-36.5433423840385,35.970448150512,38.9604238994535));
#27478=CARTESIAN_POINT('Ctrl Pts',(-36.639658321914,35.9865988630172,39.0751068228598));
#27479=CARTESIAN_POINT('Ctrl Pts',(-36.7351510411702,36.0094651718792,39.1891326632086));
#27480=CARTESIAN_POINT('Ctrl Pts',(-36.8306437604265,36.0323314807412,39.3031585035574));
#27481=CARTESIAN_POINT('Ctrl Pts',(-36.9253130496283,36.0619133353305,39.4165270083786));
#27482=CARTESIAN_POINT('Ctrl Pts',(-37.0187735220362,36.0980903116474,39.5287766687835));
#27483=CARTESIAN_POINT('Ctrl Pts',(-37.1122339944442,36.1342672879641,39.6410263291885));
#27484=CARTESIAN_POINT('Ctrl Pts',(-37.2044854431228,36.1770393059071,39.7521568966399));
#27485=CARTESIAN_POINT('Ctrl Pts',(-37.2951523240567,36.2262322459843,39.8617159726101));
#27486=CARTESIAN_POINT('Ctrl Pts',(-37.3858192049906,36.2754251860615,39.9712750485804));
#27487=CARTESIAN_POINT('Ctrl Pts',(-37.4749013174297,36.3310389393525,40.0792623904894));
#27488=CARTESIAN_POINT('Ctrl Pts',(-37.5620360193267,36.39284710928,40.1852383954844));
#27489=CARTESIAN_POINT('Ctrl Pts',(-37.6491707212237,36.4546552792075,40.2912144004794));
#27490=CARTESIAN_POINT('Ctrl Pts',(-37.7343578196495,36.522657728919,40.3951788339138));
#27491=CARTESIAN_POINT('Ctrl Pts',(-37.8172505286675,36.5965776290162,40.496708469688));
#27492=CARTESIAN_POINT('Ctrl Pts',(-37.9001432376856,36.6704975291134,40.5982381054622));
#27493=CARTESIAN_POINT('Ctrl Pts',(-37.9807413737591,36.7503347159268,40.6973327187745));
#27494=CARTESIAN_POINT('Ctrl Pts',(-38.058716832039,36.8357641823352,40.7935889079489));
#27495=CARTESIAN_POINT('Ctrl Pts',(-38.1366922903187,36.9211936487438,40.8898450971234));
#27496=CARTESIAN_POINT('Ctrl Pts',(-38.2120448981555,37.012215205594,40.9832626490344));
#27497=CARTESIAN_POINT('Ctrl Pts',(-38.2844679045839,37.1084583156049,41.0734612726074));
#27498=CARTESIAN_POINT('Ctrl Pts',(-33.7253196498837,37.443445944854,36.0531282538614));
#27499=CARTESIAN_POINT('Ctrl Pts',(-33.798220258942,37.3324461005754,36.1341628337704));
#27500=CARTESIAN_POINT('Ctrl Pts',(-33.8743328281826,37.226528886849,36.2192509666488));
#27501=CARTESIAN_POINT('Ctrl Pts',(-33.9533271021394,37.1261516015003,36.3080233588493));
#27502=CARTESIAN_POINT('Ctrl Pts',(-34.0322512328483,37.025863446521,36.3967169252868));
#27503=CARTESIAN_POINT('Ctrl Pts',(-34.1140517558741,36.9311056339844,36.4890879895414));
#27504=CARTESIAN_POINT('Ctrl Pts',(-34.1983745440842,36.8422864346562,36.584736593143));
#27505=CARTESIAN_POINT('Ctrl Pts',(-34.2826973322941,36.7534672353282,36.6803851967446));
#27506=CARTESIAN_POINT('Ctrl Pts',(-34.3695421753479,36.6705868687782,36.7793111010353));
#27507=CARTESIAN_POINT('Ctrl Pts',(-34.4585332524524,36.5940022863859,36.881086153));
#27508=CARTESIAN_POINT('Ctrl Pts',(-34.547524329557,36.5174177039936,36.9828612049648));
#27509=CARTESIAN_POINT('Ctrl Pts',(-34.6386614188727,36.4471290949209,37.0874851508487));
#27510=CARTESIAN_POINT('Ctrl Pts',(-34.7315502490925,36.3834390239837,37.1945053382339));
#27511=CARTESIAN_POINT('Ctrl Pts',(-34.8244390793125,36.3197489530465,37.301525525619));
#27512=CARTESIAN_POINT('Ctrl Pts',(-34.9190794190056,36.2626575773783,37.4109416878363));
#27513=CARTESIAN_POINT('Ctrl Pts',(-35.0150619477641,36.2124104765838,37.5222805784061));
#27514=CARTESIAN_POINT('Ctrl Pts',(-35.1110444765225,36.1621633757894,37.6336194689758));
#27515=CARTESIAN_POINT('Ctrl Pts',(-35.2083689553143,36.1187606736282,37.746880810608));
#27516=CARTESIAN_POINT('Ctrl Pts',(-35.3066145450565,36.0823888566362,37.8615748447133));
#27517=CARTESIAN_POINT('Ctrl Pts',(-35.4048601347988,36.0460170396441,37.9762688788185));
#27518=CARTESIAN_POINT('Ctrl Pts',(-35.5040265909137,36.0166761971474,38.09239531987));
#27519=CARTESIAN_POINT('Ctrl Pts',(-35.6036851847274,35.9944921235898,38.2094521206313));
#27520=CARTESIAN_POINT('Ctrl Pts',(-35.7033437785412,35.9723080500322,38.3265089213925));
#27521=CARTESIAN_POINT('Ctrl Pts',(-35.8034942620323,35.9572807995434,38.4444957905543));
#27522=CARTESIAN_POINT('Ctrl Pts',(-35.9037037134776,35.9494743979637,38.5629027208967));
#27523=CARTESIAN_POINT('Ctrl Pts',(-36.003913164923,35.941667996384,38.6813096512391));
#27524=CARTESIAN_POINT('Ctrl Pts',(-36.1041813349894,35.941082462185,38.8001363481746));
#27525=CARTESIAN_POINT('Ctrl Pts',(-36.2040748411289,35.9477195077942,38.9188692411561));
#27526=CARTESIAN_POINT('Ctrl Pts',(-36.3039683472685,35.9543565534034,39.0376021341376));
#27527=CARTESIAN_POINT('Ctrl Pts',(-36.4034869409791,35.9682161614792,39.1562409278309));
#27528=CARTESIAN_POINT('Ctrl Pts',(-36.5022005147178,35.9892377225577,39.2742729152236));
#27529=CARTESIAN_POINT('Ctrl Pts',(-36.6009140884566,36.0102592836361,39.3923049026164));
#27530=CARTESIAN_POINT('Ctrl Pts',(-36.6988223966881,36.0384427447144,39.5097297901655));
#27531=CARTESIAN_POINT('Ctrl Pts',(-36.7955023142031,36.073665702312,39.6260401534171));
#27532=CARTESIAN_POINT('Ctrl Pts',(-36.8921822317181,36.1088886599098,39.7423505166686));
#27533=CARTESIAN_POINT('Ctrl Pts',(-36.987633518058,36.1511510258213,39.8575460663928));
#27534=CARTESIAN_POINT('Ctrl Pts',(-37.0814436773156,36.2002696622019,39.9711290339064));
#27535=CARTESIAN_POINT('Ctrl Pts',(-37.1752538365732,36.2493882985826,40.0847120014199));
#27536=CARTESIAN_POINT('Ctrl Pts',(-37.2674226354332,36.3053630827835,40.196682104292));
#27537=CARTESIAN_POINT('Ctrl Pts',(-37.3575517625599,36.3679517248826,40.3065555194336));
#27538=CARTESIAN_POINT('Ctrl Pts',(-37.4476808896867,36.4305403669817,40.4164289345753));
#27539=CARTESIAN_POINT('Ctrl Pts',(-37.5357701209128,36.4997427109428,40.5242053887811));
#27540=CARTESIAN_POINT('Ctrl Pts',(-37.6214387624945,36.5752594060612,40.6294191741335));
#27541=CARTESIAN_POINT('Ctrl Pts',(-37.7071074040762,36.6507761011797,40.7346329594859));
#27542=CARTESIAN_POINT('Ctrl Pts',(-37.7903552429203,36.7326069593742,40.8372838143524));
#27543=CARTESIAN_POINT('Ctrl Pts',(-37.8708224841454,36.8203981514681,40.9369281594897));
#27544=CARTESIAN_POINT('Ctrl Pts',(-37.9512897253705,36.908189343562,41.036572504627));
#27545=CARTESIAN_POINT('Ctrl Pts',(-38.0289761687888,37.0019406510458,41.1332100922236));
#27546=CARTESIAN_POINT('Ctrl Pts',(-38.1035460197056,37.101246817389,41.2264232946562));
#27547=CARTESIAN_POINT('Ctrl Pts',(-33.4464716391097,37.6027954918844,36.0847240772064));
#27548=CARTESIAN_POINT('Ctrl Pts',(-33.5182678730472,37.4833965665413,36.1640670442977));
#27549=CARTESIAN_POINT('Ctrl Pts',(-33.5936274837347,37.3691410204676,36.2479030934173));
#27550=CARTESIAN_POINT('Ctrl Pts',(-33.6722029585856,37.2605528414183,36.3358454797662));
#27551=CARTESIAN_POINT('Ctrl Pts',(-33.7507086620627,37.1520610836308,36.4237097773588));
#27552=CARTESIAN_POINT('Ctrl Pts',(-33.8324242998089,37.0492269351005,36.5156728750437));
#27553=CARTESIAN_POINT('Ctrl Pts',(-33.9169739581447,36.9525210040537,36.6113116112086));
#27554=CARTESIAN_POINT('Ctrl Pts',(-34.0015236164805,36.8558150730067,36.7069503473736));
#27555=CARTESIAN_POINT('Ctrl Pts',(-34.0889070572831,36.7652376288277,36.806264452547));
#27556=CARTESIAN_POINT('Ctrl Pts',(-34.1787224889782,36.681203003299,36.9087972015629));
#27557=CARTESIAN_POINT('Ctrl Pts',(-34.2685379206733,36.5971683777704,37.0113299505787));
#27558=CARTESIAN_POINT('Ctrl Pts',(-34.3607850905433,36.5196768047354,37.1170810548562));
#27559=CARTESIAN_POINT('Ctrl Pts',(-34.4550400125873,36.4490825631191,37.2255644135308));
#27560=CARTESIAN_POINT('Ctrl Pts',(-34.5492949346313,36.3784883215028,37.3340477722053));
#27561=CARTESIAN_POINT('Ctrl Pts',(-34.6455573438433,36.3147916074869,37.4452630802213));
#27562=CARTESIAN_POINT('Ctrl Pts',(-34.7433849450011,36.2582834200688,37.5586993159057));
#27563=CARTESIAN_POINT('Ctrl Pts',(-34.8412125461588,36.2017752326507,37.67213555159));
#27564=CARTESIAN_POINT('Ctrl Pts',(-34.9406050643861,36.1524557285732,37.7877923961955));
#27565=CARTESIAN_POINT('Ctrl Pts',(-35.0411059467308,36.1105499784281,37.9051385885108));
#27566=CARTESIAN_POINT('Ctrl Pts',(-35.1416068290756,36.0686442282829,38.0224847808262));
#27567=CARTESIAN_POINT('Ctrl Pts',(-35.2432157932981,36.0341523479556,38.1415199913194));
#27568=CARTESIAN_POINT('Ctrl Pts',(-35.3454662095403,36.0072314337289,38.2616975841894));
#27569=CARTESIAN_POINT('Ctrl Pts',(-35.4477166257825,35.9803105195023,38.3818751770595));
#27570=CARTESIAN_POINT('Ctrl Pts',(-35.550608207014,35.9609606453576,38.503194814994));
#27571=CARTESIAN_POINT('Ctrl Pts',(-35.6536685185057,35.9492695084397,38.6250994918713));
#27572=CARTESIAN_POINT('Ctrl Pts',(-35.7567288299973,35.9375783715217,38.7470041687487));
#27573=CARTESIAN_POINT('Ctrl Pts',(-35.8599575825441,35.933546003242,38.86949354255));
#27574=CARTESIAN_POINT('Ctrl Pts',(-35.9628808608495,35.9371899107033,38.9920053348079));
#27575=CARTESIAN_POINT('Ctrl Pts',(-36.0658041391548,35.9408338181645,39.1145171270658));
#27576=CARTESIAN_POINT('Ctrl Pts',(-36.1684216544745,35.9521539899298,39.2370509941715));
#27577=CARTESIAN_POINT('Ctrl Pts',(-36.2702623481083,35.9710975931683,39.359044530537));
#27578=CARTESIAN_POINT('Ctrl Pts',(-36.3721030417422,35.9900411964069,39.4810380669025));
#27579=CARTESIAN_POINT('Ctrl Pts',(-36.4731666280375,36.016608176944,39.6024909304591));
#27580=CARTESIAN_POINT('Ctrl Pts',(-36.5729892153952,36.0506758543964,39.722845734098));
#27581=CARTESIAN_POINT('Ctrl Pts',(-36.6728118027528,36.0847435318488,39.8432005377368));
#27582=CARTESIAN_POINT('Ctrl Pts',(-36.771393111214,36.1263118098031,39.9624569440451));
#27583=CARTESIAN_POINT('Ctrl Pts',(-36.8682806608543,36.1751892903995,40.0800676834957));
#27584=CARTESIAN_POINT('Ctrl Pts',(-36.9651682104947,36.2240667709959,40.1976784229463));
#27585=CARTESIAN_POINT('Ctrl Pts',(-37.0603617295996,36.2802533164657,40.3136431658551));
#27586=CARTESIAN_POINT('Ctrl Pts',(-37.153424289896,36.3434905688718,40.4274297664406));
#27587=CARTESIAN_POINT('Ctrl Pts',(-37.2464868501925,36.4067278212778,40.5412163670262));
#27588=CARTESIAN_POINT('Ctrl Pts',(-37.3374181906852,36.4770156027545,40.6528245063355));
#27589=CARTESIAN_POINT('Ctrl Pts',(-37.4258009324191,36.554030963938,40.7617420299664));
#27590=CARTESIAN_POINT('Ctrl Pts',(-37.5141836741531,36.6310463251215,40.8706595535973));
#27591=CARTESIAN_POINT('Ctrl Pts',(-37.6000175692298,36.7147890496724,40.9768861562323));
#27592=CARTESIAN_POINT('Ctrl Pts',(-37.6829086069535,36.8048745550757,41.0799343596235));
#27593=CARTESIAN_POINT('Ctrl Pts',(-37.7657996446773,36.894960060479,41.1829825630148));
#27594=CARTESIAN_POINT('Ctrl Pts',(-37.8457475925048,36.991388093894,41.2828520782612));
#27595=CARTESIAN_POINT('Ctrl Pts',(-37.9223854134262,37.0937159605723,41.3790845625229));
#27596=CARTESIAN_POINT('Ctrl Pts',(-33.1766930776214,37.7705087843601,36.1244244172113));
#27597=CARTESIAN_POINT('Ctrl Pts',(-33.2469057853303,37.6427433806131,36.2014333689329));
#27598=CARTESIAN_POINT('Ctrl Pts',(-33.3210512350507,37.5201296639953,36.2834032413025));
#27599=CARTESIAN_POINT('Ctrl Pts',(-33.3987671367845,37.4032666996501,36.3699335096646));
#27600=CARTESIAN_POINT('Ctrl Pts',(-33.4764140304055,37.2865075041919,36.4563869431656));
#27601=CARTESIAN_POINT('Ctrl Pts',(-33.5576247911777,37.1754892239836,36.5473924025272));
#27602=CARTESIAN_POINT('Ctrl Pts',(-33.6420033278953,37.0707533308666,36.6425060244189));
#27603=CARTESIAN_POINT('Ctrl Pts',(-33.7263818646128,36.9660174377497,36.7376196463106));
#27604=CARTESIAN_POINT('Ctrl Pts',(-33.8139279089859,36.8675642647401,36.836841128309));
#27605=CARTESIAN_POINT('Ctrl Pts',(-33.9042144706173,36.7758739995088,36.9396865349718));
#27606=CARTESIAN_POINT('Ctrl Pts',(-33.9945010322489,36.6841837342774,37.0425319416347));
#27607=CARTESIAN_POINT('Ctrl Pts',(-34.0875278240641,36.5992566683603,37.149000945955));
#27608=CARTESIAN_POINT('Ctrl Pts',(-34.1828411243289,36.5215070181751,37.2585742640763));
#27609=CARTESIAN_POINT('Ctrl Pts',(-34.2781544245936,36.4437573679901,37.3681475821975));
#27610=CARTESIAN_POINT('Ctrl Pts',(-34.3757539302503,36.3731853807473,37.4808248657209));
#27611=CARTESIAN_POINT('Ctrl Pts',(-34.4751636170032,36.3101352584734,37.5960565511047));
#27612=CARTESIAN_POINT('Ctrl Pts',(-34.5745733037561,36.2470851361995,37.7112882364884));
#27613=CARTESIAN_POINT('Ctrl Pts',(-34.675792855523,36.1915570793665,37.8290739573426));
#27614=CARTESIAN_POINT('Ctrl Pts',(-34.778328591915,36.1438219158808,37.9488392347248));
#27615=CARTESIAN_POINT('Ctrl Pts',(-34.8808643283069,36.0960867523952,38.068604512107));
#27616=CARTESIAN_POINT('Ctrl Pts',(-34.9847159233021,36.0561446340336,38.1903489652127));
#27617=CARTESIAN_POINT('Ctrl Pts',(-35.0893768592252,36.0241903710571,38.3134788071787));
#27618=CARTESIAN_POINT('Ctrl Pts',(-35.1940377951484,35.9922361080806,38.4366086491448));
#27619=CARTESIAN_POINT('Ctrl Pts',(-35.2995077392206,35.9682698020891,38.5611234884689));
#27620=CARTESIAN_POINT('Ctrl Pts',(-35.4052722805894,35.9524083441775,38.6864160263084));
#27621=CARTESIAN_POINT('Ctrl Pts',(-35.5110368219582,35.9365468862658,38.8117085641479));
#27622=CARTESIAN_POINT('Ctrl Pts',(-35.6170956243359,35.9287903268657,38.9377784021244));
#27623=CARTESIAN_POINT('Ctrl Pts',(-35.7229314048457,35.9291764969512,39.0640106572437));
#27624=CARTESIAN_POINT('Ctrl Pts',(-35.8287671853555,35.9295626670368,39.190242912363));
#27625=CARTESIAN_POINT('Ctrl Pts',(-35.9343796074835,35.9380915653791,39.316637183259));
#27626=CARTESIAN_POINT('Ctrl Pts',(-36.0392535655137,35.9547215935791,39.4425770046408));
#27627=CARTESIAN_POINT('Ctrl Pts',(-36.144127523544,35.971351621779,39.5685168260227));
#27628=CARTESIAN_POINT('Ctrl Pts',(-36.2482626840209,35.996082726959,39.6940017974544));
#27629=CARTESIAN_POINT('Ctrl Pts',(-36.3511511463227,36.0287942874002,39.8184198886456));
#27630=CARTESIAN_POINT('Ctrl Pts',(-36.4540396086244,36.0615058478414,39.9428379798368));
#27631=CARTESIAN_POINT('Ctrl Pts',(-36.5556810456084,36.1021977595337,40.0661887951901));
#27632=CARTESIAN_POINT('Ctrl Pts',(-36.6555797193503,36.1506715548338,40.1878707134216));
#27633=CARTESIAN_POINT('Ctrl Pts',(-36.7554783930923,36.1991453501339,40.3095526316531));
#27634=CARTESIAN_POINT('Ctrl Pts',(-36.853633985956,36.2554008749145,40.4295652658654));
#27635=CARTESIAN_POINT('Ctrl Pts',(-36.949567761598,36.3191637528529,40.5473232761837));
#27636=CARTESIAN_POINT('Ctrl Pts',(-37.04550153724,36.3829266307912,40.6650812865021));
#27637=CARTESIAN_POINT('Ctrl Pts',(-37.1392131906308,36.4541966591475,40.7805842985054));
#27638=CARTESIAN_POINT('Ctrl Pts',(-37.2302456599391,36.5326262311041,40.8932689672078));
#27639=CARTESIAN_POINT('Ctrl Pts',(-37.3212781292474,36.6110558030609,41.0059536359101));
#27640=CARTESIAN_POINT('Ctrl Pts',(-37.4096311250278,36.6966446692444,41.1158196030214));
#27641=CARTESIAN_POINT('Ctrl Pts',(-37.4948737213283,36.7889753853261,41.2223310172326));
#27642=CARTESIAN_POINT('Ctrl Pts',(-37.5801163176289,36.8813061014078,41.3288424314437));
#27643=CARTESIAN_POINT('Ctrl Pts',(-37.6622482434134,36.9803783738144,41.4319989540929));
#27644=CARTESIAN_POINT('Ctrl Pts',(-37.7408689148655,37.0857089953691,41.5312974579708));
#27645=CARTESIAN_POINT('',(-37.7834004681043,37.0875767698756,41.4956185460356));
#27646=CARTESIAN_POINT('Ctrl Pts',(-41.7981279794346,37.2631014686576,38.1264711628116));
#27647=CARTESIAN_POINT('Ctrl Pts',(-41.7952803682454,37.2626276178739,38.1282941998091));
#27648=CARTESIAN_POINT('Ctrl Pts',(-41.7924327570584,37.2621537670904,38.1301172368054));
#27649=CARTESIAN_POINT('Ctrl Pts',(-41.7895851458665,37.2616799163062,38.1319402738046));
#27650=CARTESIAN_POINT('Ctrl Pts',(-41.7888732430902,37.2615614536138,38.1323960330406));
#27651=CARTESIAN_POINT('Ctrl Pts',(-41.7881613402824,37.261442990916,38.1328517922966));
#27652=CARTESIAN_POINT('Ctrl Pts',(-41.7874494374748,37.2613245282183,38.1333075515525));
#27653=CARTESIAN_POINT('Ctrl Pts',(-41.7870934860748,37.2612652968701,38.133535431178));
#27654=CARTESIAN_POINT('Ctrl Pts',(-41.7867375346748,37.2612060655218,38.1337633108035));
#27655=CARTESIAN_POINT('Ctrl Pts',(-41.7863815832788,37.2611468341743,38.1339911904264));
#27656=CARTESIAN_POINT('Ctrl Pts',(-41.7860256318321,37.2610876028183,38.1342190700819));
#27657=CARTESIAN_POINT('Ctrl Pts',(-41.7856628656225,37.2610301617684,38.1344560559244));
#27658=CARTESIAN_POINT('Ctrl Pts',(-41.7853034269248,37.2609721218352,38.1346890419301));
#27659=CARTESIAN_POINT('Ctrl Pts',(-41.7838656722769,37.2607399621266,38.1356209858621));
#27660=CARTESIAN_POINT('Ctrl Pts',(-41.7824297932713,37.2605103116342,38.1365552928376));
#27661=CARTESIAN_POINT('Ctrl Pts',(-41.780995781495,37.2602831590315,38.1374919521413));
#27662=CARTESIAN_POINT('Ctrl Pts',(-41.7752597343898,37.259374548621,38.1412385893563));
#27663=CARTESIAN_POINT('Ctrl Pts',(-41.7695535667904,37.2585059112087,38.1450228712984));
#27664=CARTESIAN_POINT('Ctrl Pts',(-41.7638757728966,37.257675231489,38.1488428994769));
#27665=CARTESIAN_POINT('Ctrl Pts',(-41.7581979790448,37.2568445517755,38.1526629276272));
#27666=CARTESIAN_POINT('Ctrl Pts',(-41.7525485535461,37.2560518229013,38.1565186957688));
#27667=CARTESIAN_POINT('Ctrl Pts',(-41.7469251703319,37.2552939330802,38.1604072733946));
#27668=CARTESIAN_POINT('Ctrl Pts',(-41.7413017870347,37.254536043248,38.1642958510777));
#27669=CARTESIAN_POINT('Ctrl Pts',(-41.7357044238504,37.2538129628078,38.1682172103118));
#27670=CARTESIAN_POINT('Ctrl Pts',(-41.7301301522264,37.2531207739776,38.1721676615473));
#27671=CARTESIAN_POINT('Ctrl Pts',(-41.7245558806842,37.2524285851575,38.176118112725));
#27672=CARTESIAN_POINT('Ctrl Pts',(-41.7190046733824,37.251767251399,38.1800976214849));
#27673=CARTESIAN_POINT('Ctrl Pts',(-41.7134733845952,37.2511325643884,38.184102224671));
#27674=CARTESIAN_POINT('Ctrl Pts',(-41.7079420957676,37.2504978773732,38.1881068278865));
#27675=CARTESIAN_POINT('Ctrl Pts',(-41.7024307055449,37.2498898104708,38.1921365004449));
#27676=CARTESIAN_POINT('Ctrl Pts',(-41.6969362138226,37.2493043501777,38.1961874626515));
#27677=CARTESIAN_POINT('Ctrl Pts',(-41.6914417221003,37.2487188898845,38.200238424858));
#27678=CARTESIAN_POINT('Ctrl Pts',(-41.6859641201875,37.2481560245742,38.2043106657638));
#27679=CARTESIAN_POINT('Ctrl Pts',(-41.6805007672794,37.2476122214099,38.2084008583392));
#27680=CARTESIAN_POINT('Ctrl Pts',(-41.675037414332,37.2470684182417,38.2124910509441));
#27681=CARTESIAN_POINT('Ctrl Pts',(-41.6695883098069,37.2465436764404,38.2165991944852));
#27682=CARTESIAN_POINT('Ctrl Pts',(-41.6641512373951,37.2460350310546,38.2207224967357));
#27683=CARTESIAN_POINT('Ctrl Pts',(-41.6532770926885,37.2450177402938,38.2289691011478));
#27684=CARTESIAN_POINT('Ctrl Pts',(-41.6424507433835,37.2440643896428,38.2372759208019));
#27685=CARTESIAN_POINT('Ctrl Pts',(-41.6316590585708,37.24315741273,38.2456264126654));
#27686=CARTESIAN_POINT('Ctrl Pts',(-41.6208673736816,37.2422504358108,38.2539769045882));
#27687=CARTESIAN_POINT('Ctrl Pts',(-41.6101104832692,37.2413900065215,38.2623712324819));
#27688=CARTESIAN_POINT('Ctrl Pts',(-41.5993797204532,37.2405645304145,38.2707984773402));
#27689=CARTESIAN_POINT('Ctrl Pts',(-41.5886489577125,37.2397390543133,38.2792257221395));
#27690=CARTESIAN_POINT('Ctrl Pts',(-41.5779444113226,37.238948650129,38.287685995721));
#27691=CARTESIAN_POINT('Ctrl Pts',(-41.5672602276774,37.2381854869781,38.2961719233939));
#27692=CARTESIAN_POINT('Ctrl Pts',(-41.5565760439582,37.2374223238219,38.3046578511256));
#27693=CARTESIAN_POINT('Ctrl Pts',(-41.5459122765069,37.2366864733018,38.31316950038));
#27694=CARTESIAN_POINT('Ctrl Pts',(-41.5352648323389,37.2359724598726,38.3217017145931));
#27695=CARTESIAN_POINT('Ctrl Pts',(-41.524617388244,37.2352584464482,38.3302339287476));
#27696=CARTESIAN_POINT('Ctrl Pts',(-41.5139862993864,37.2345663128625,38.3387867481182));
#27697=CARTESIAN_POINT('Ctrl Pts',(-41.5033686034439,37.2338920961565,38.3473564406103));
#27698=CARTESIAN_POINT('Ctrl Pts',(-41.492750907465,37.2332178794481,38.3559261331318));
#27699=CARTESIAN_POINT('Ctrl Pts',(-41.4821466239335,37.2325616057495,38.3645127233828));
#27700=CARTESIAN_POINT('Ctrl Pts',(-41.4715535415973,37.2319203168746,38.3731134255079));
#27701=CARTESIAN_POINT('Ctrl Pts',(-41.4503673768902,37.2306377391226,38.3903148297865));
#27702=CARTESIAN_POINT('Ctrl Pts',(-41.4292256929265,37.2294146671707,38.4075722733206));
#27703=CARTESIAN_POINT('Ctrl Pts',(-41.4081164361093,37.228234975863,38.4248705703345));
#27704=CARTESIAN_POINT('Ctrl Pts',(-41.3870071793618,37.2270552845593,38.4421688672915));
#27705=CARTESIAN_POINT('Ctrl Pts',(-41.3659305268728,37.2259192108381,38.4595082408637));
#27706=CARTESIAN_POINT('Ctrl Pts',(-41.3448787787704,37.2248164539037,38.4768789903342));
#27707=CARTESIAN_POINT('Ctrl Pts',(-41.3238270305998,37.2237136969658,38.4942497398608));
#27708=CARTESIAN_POINT('Ctrl Pts',(-41.3028002730303,37.2226443721514,38.5116519739034));
#27709=CARTESIAN_POINT('Ctrl Pts',(-41.2817932595768,37.2216014607763,38.5290790826552));
#27710=CARTESIAN_POINT('Ctrl Pts',(-41.2607862461898,37.2205585494046,38.5465061913519));
#27711=CARTESIAN_POINT('Ctrl Pts',(-41.2397990228863,37.2195421129669,38.5639582326701));
#27712=CARTESIAN_POINT('Ctrl Pts',(-41.2188278343381,37.2185471276308,38.5814304754436));
#27713=CARTESIAN_POINT('Ctrl Pts',(-41.1978566457246,37.2175521422917,38.5989027182715));
#27714=CARTESIAN_POINT('Ctrl Pts',(-41.1769015182199,37.2165786433093,38.6163951957561));
#27715=CARTESIAN_POINT('Ctrl Pts',(-41.1559596578763,37.2156228929745,38.6339043879306));
#27716=CARTESIAN_POINT('Ctrl Pts',(-41.1350177975965,37.2146671426426,38.6514135800517));
#27717=CARTESIAN_POINT('Ctrl Pts',(-41.1140892204956,37.2137291623866,38.6689395070428));
#27718=CARTESIAN_POINT('Ctrl Pts',(-41.0931717822014,37.2128060834914,38.6864794673073));
#27719=CARTESIAN_POINT('Ctrl Pts',(-41.0722543438446,37.2118830045934,38.7040194276243));
#27720=CARTESIAN_POINT('Ctrl Pts',(-41.0513480545069,37.2109748407181,38.7215734340807));
#27721=CARTESIAN_POINT('Ctrl Pts',(-41.0304512257111,37.2100793330414,38.7391393594415));
#27722=CARTESIAN_POINT('Ctrl Pts',(-40.9886575682115,37.2082883176918,38.774271210086));
#27723=CARTESIAN_POINT('Ctrl Pts',(-40.9469015299109,37.2065476288515,38.8094504554401));
#27724=CARTESIAN_POINT('Ctrl Pts',(-40.905173253682,37.2048440797747,38.8446646769593));
#27725=CARTESIAN_POINT('Ctrl Pts',(-40.8634449773944,37.2031405306954,38.879878898528));
#27726=CARTESIAN_POINT('Ctrl Pts',(-40.8217445702088,37.2014742645636,38.9151282311048));
#27727=CARTESIAN_POINT('Ctrl Pts',(-40.7800652132294,37.1998361591428,38.9504040838741));
#27728=CARTESIAN_POINT('Ctrl Pts',(-40.7383858563063,37.1981980537242,38.9856799365958));
#27729=CARTESIAN_POINT('Ctrl Pts',(-40.6967276065313,37.1965881851929,39.0209823812487));
#27730=CARTESIAN_POINT('Ctrl Pts',(-40.6550854902778,37.1949998998914,39.056305151788));
#27731=CARTESIAN_POINT('Ctrl Pts',(-40.6134433739704,37.1934116145878,39.0916279223729));
#27732=CARTESIAN_POINT('Ctrl Pts',(-40.5718174239146,37.1918449562999,39.1269710600792));
#27733=CARTESIAN_POINT('Ctrl Pts',(-40.5302038548951,37.1902948612125,39.1623297960873));
#27734=CARTESIAN_POINT('Ctrl Pts',(-40.488590285927,37.188744766127,39.1976885320517));
#27735=CARTESIAN_POINT('Ctrl Pts',(-40.4469891179915,37.1872112609928,39.2330628915102));
#27736=CARTESIAN_POINT('Ctrl Pts',(-40.4053973662081,37.1856903526728,39.2684491139483));
#27737=CARTESIAN_POINT('Ctrl Pts',(-40.3638056143756,37.1841694443511,39.3038353364282));
#27738=CARTESIAN_POINT('Ctrl Pts',(-40.3222232915335,37.1826611500186,39.3392334380622));
#27739=CARTESIAN_POINT('Ctrl Pts',(-40.2806479706236,37.1811622227862,39.3746403611105));
#27740=CARTESIAN_POINT('Ctrl Pts',(-40.1974973288739,37.178164368324,39.4454542071473));
#27741=CARTESIAN_POINT('Ctrl Pts',(-40.1143744321379,37.1752036308053,39.5163030078588));
#27742=CARTESIAN_POINT('Ctrl Pts',(-40.0312642571702,37.1722599123143,39.5871678361448));
#27743=CARTESIAN_POINT('Ctrl Pts',(-39.9481540821605,37.1693161938219,39.6580326644667));
#27744=CARTESIAN_POINT('Ctrl Pts',(-39.8650567681428,37.1663896806089,39.7289136957646));
#27745=CARTESIAN_POINT('Ctrl Pts',(-39.78196079965,37.1634649674229,39.799796422228));
#27746=CARTESIAN_POINT('Ctrl Pts',(-39.6988648311948,37.1605402542383,39.8706791486594));
#27747=CARTESIAN_POINT('Ctrl Pts',(-39.6157702857781,37.1576174447775,39.941563667912));
#27748=CARTESIAN_POINT('Ctrl Pts',(-39.5326675761395,37.1546837133193,40.0124379014345));
#27749=CARTESIAN_POINT('Ctrl Pts',(-39.4495648664821,37.1517499818605,40.0833121349731));
#27750=CARTESIAN_POINT('Ctrl Pts',(-39.3664540409006,37.1488053930167,40.1541761436298));
#27751=CARTESIAN_POINT('Ctrl Pts',(-39.2833265166636,37.1458384649135,40.2250191144136));
#27752=CARTESIAN_POINT('Ctrl Pts',(-39.2001989924265,37.1428715368103,40.2958620851973));
#27753=CARTESIAN_POINT('Ctrl Pts',(-39.1170548033789,37.1398823147253,40.366684060748));
#27754=CARTESIAN_POINT('Ctrl Pts',(-39.0338857649331,37.1368598494162,40.4374747296777));
#27755=CARTESIAN_POINT('Ctrl Pts',(-38.9507167264778,37.1338373841067,40.5082653986154));
#27756=CARTESIAN_POINT('Ctrl Pts',(-38.8675228655626,37.1307817116108,40.5790247948705));
#27757=CARTESIAN_POINT('Ctrl Pts',(-38.7842959451795,37.127681812559,40.6497425410132));
#27758=CARTESIAN_POINT('Ctrl Pts',(-38.7010690248156,37.124581913508,40.7204602871396));
#27759=CARTESIAN_POINT('Ctrl Pts',(-38.6178090694157,37.1214378205856,40.791136413934));
#27760=CARTESIAN_POINT('Ctrl Pts',(-38.5345074076489,37.1182379333905,40.8617599967831));
#27761=CARTESIAN_POINT('Ctrl Pts',(-38.4512057458678,37.1150380461948,40.9323835796444));
#27762=CARTESIAN_POINT('Ctrl Pts',(-38.3678624026822,37.1117823981208,41.0029546500094));
#27763=CARTESIAN_POINT('Ctrl Pts',(-38.2844679045694,37.1084583156043,41.0734612726197));
#27764=CARTESIAN_POINT('Ctrl Pts',(-38.1176789083584,37.1018101505721,41.2144745178281));
#27765=CARTESIAN_POINT('Ctrl Pts',(-37.9506870299514,37.0948905721936,41.3552321610306));
#27766=CARTESIAN_POINT('Ctrl Pts',(-37.7834004681043,37.0875767698756,41.4956185460356));
#27767=CARTESIAN_POINT('Origin',(-35.6284929434833,40.9281765976896,39.1278840755075));
#27768=CARTESIAN_POINT('Ctrl Pts',(-38.0398886763086,37.4073630839359,41.7808966890464));
#27769=CARTESIAN_POINT('Ctrl Pts',(-37.9326177918203,37.4114807225354,41.8852044318755));
#27770=CARTESIAN_POINT('Ctrl Pts',(-37.8096166958413,37.3290227884235,41.8633979578226));
#27771=CARTESIAN_POINT('Ctrl Pts',(-37.6866155998624,37.2465648543116,41.8415914837696));
#27772=CARTESIAN_POINT('Ctrl Pts',(-37.6777121386978,37.1645658239806,41.7166875597931));
#27773=CARTESIAN_POINT('Ctrl Pts',(-37.6688086775333,37.0825667936495,41.5917836358167));
#27774=CARTESIAN_POINT('Ctrl Pts',(-37.7834004681593,37.087576769944,41.4956185461047));
#27775=CARTESIAN_POINT('Ctrl Pts',(-40.7814290969457,40.6059367497034,44.4740514613886));
#27776=CARTESIAN_POINT('Ctrl Pts',(-38.5287405218227,40.692407160327,46.6645140616453));
#27777=CARTESIAN_POINT('Ctrl Pts',(-35.9457175052688,38.960790543309,46.2065781063563));
#27778=CARTESIAN_POINT('Ctrl Pts',(-33.362694488715,37.229173926291,45.7486421510673));
#27779=CARTESIAN_POINT('Ctrl Pts',(-33.1757218041875,35.5071942886757,43.1256597465504));
#27780=CARTESIAN_POINT('Ctrl Pts',(-32.9887491196601,33.7852146510605,40.5026773420335));
#27781=CARTESIAN_POINT('Ctrl Pts',(-35.3951767237337,33.8904241532856,38.4832104573036));
#27782=CARTESIAN_POINT('Ctrl Pts',(-38.6265215723274,44.4465365775852,42.1063169907319));
#27783=CARTESIAN_POINT('Ctrl Pts',(-36.3738329972119,44.5330069882085,44.2967795909812));
#27784=CARTESIAN_POINT('Ctrl Pts',(-33.7908099806667,42.8013903711963,43.8388436356938));
#27785=CARTESIAN_POINT('Ctrl Pts',(-31.2077869641214,41.0697737541841,43.3809076804063));
#27786=CARTESIAN_POINT('Ctrl Pts',(-31.0208142795946,39.3477941165746,40.7579252758982));
#27787=CARTESIAN_POINT('Ctrl Pts',(-30.8338415950678,37.6258144789651,38.13494287139));
#27788=CARTESIAN_POINT('Ctrl Pts',(-33.2402691991333,37.7310239811898,36.1154759866669));
#27789=CARTESIAN_POINT('',(-38.0398886763558,37.4073630839945,41.7808966890927));
#27790=CARTESIAN_POINT('Origin',(-35.8849811517349,41.2479629118085,39.4131622185645));
#27791=CARTESIAN_POINT('Origin',(-37.9028116553955,37.2474344007039,41.6462389504159));
#27792=CARTESIAN_POINT('Ctrl Pts',(-41.7981279794346,37.2631014686576,38.1264711628116));
#27793=CARTESIAN_POINT('Ctrl Pts',(-41.7981279794346,37.2631014686576,38.1264711628116));
#27794=CARTESIAN_POINT('Ctrl Pts',(-41.7981279794346,37.2631014686576,38.1264711628116));
#27795=CARTESIAN_POINT('Ctrl Pts',(-41.7981279794346,37.2631014686576,38.1264711628116));
#27796=CARTESIAN_POINT('Ctrl Pts',(-41.7981279794346,37.2631014686576,38.1264711628116));
#27797=CARTESIAN_POINT('Ctrl Pts',(-41.7981279794346,37.2631014686576,38.1264711628116));
#27798=CARTESIAN_POINT('Ctrl Pts',(-41.7981279794346,37.2631014686576,38.1264711628116));
#27799=CARTESIAN_POINT('Ctrl Pts',(-41.7981279794346,37.2631014686576,38.1264711628116));
#27800=CARTESIAN_POINT('Ctrl Pts',(-41.7981279794346,37.2631014686576,38.1264711628116));
#27801=CARTESIAN_POINT('Ctrl Pts',(-41.7981279794346,37.2631014686576,38.1264711628116));
#27802=CARTESIAN_POINT('Ctrl Pts',(-41.7981279794346,37.2631014686576,38.1264711628116));
#27803=CARTESIAN_POINT('Ctrl Pts',(-41.7981279794346,37.2631014686576,38.1264711628116));
#27804=CARTESIAN_POINT('Ctrl Pts',(-41.7981279794346,37.2631014686576,38.1264711628116));
#27805=CARTESIAN_POINT('Ctrl Pts',(-41.7981279794346,37.2631014686576,38.1264711628116));
#27806=CARTESIAN_POINT('Ctrl Pts',(-41.7981279794346,37.2631014686576,38.1264711628116));
#27807=CARTESIAN_POINT('Ctrl Pts',(-41.7981279794346,37.2631014686576,38.1264711628116));
#27808=CARTESIAN_POINT('Ctrl Pts',(-41.7981279794346,37.2631014686576,38.1264711628116));
#27809=CARTESIAN_POINT('Ctrl Pts',(-41.7981279794346,37.2631014686576,38.1264711628116));
#27810=CARTESIAN_POINT('Ctrl Pts',(-41.7981279794346,37.2631014686576,38.1264711628116));
#27811=CARTESIAN_POINT('Ctrl Pts',(-41.7981279794346,37.2631014686576,38.1264711628116));
#27812=CARTESIAN_POINT('Ctrl Pts',(-41.7981279794346,37.2631014686576,38.1264711628116));
#27813=CARTESIAN_POINT('Ctrl Pts',(-41.7981279794346,37.2631014686576,38.1264711628116));
#27814=CARTESIAN_POINT('Ctrl Pts',(-41.7981279794346,37.2631014686576,38.1264711628116));
#27815=CARTESIAN_POINT('Ctrl Pts',(-41.7981279794346,37.2631014686576,38.1264711628116));
#27816=CARTESIAN_POINT('Ctrl Pts',(-41.7981279794346,37.2631014686576,38.1264711628116));
#27817=CARTESIAN_POINT('Ctrl Pts',(-41.7981279794346,37.2631014686576,38.1264711628116));
#27818=CARTESIAN_POINT('Ctrl Pts',(-41.7981279794346,37.2631014686576,38.1264711628116));
#27819=CARTESIAN_POINT('Ctrl Pts',(-41.7981279794346,37.2631014686576,38.1264711628116));
#27820=CARTESIAN_POINT('Ctrl Pts',(-41.7981279794346,37.2631014686576,38.1264711628116));
#27821=CARTESIAN_POINT('Ctrl Pts',(-41.7981279794346,37.2631014686576,38.1264711628116));
#27822=CARTESIAN_POINT('Ctrl Pts',(-41.7981279794346,37.2631014686576,38.1264711628116));
#27823=CARTESIAN_POINT('Ctrl Pts',(-41.7981279794346,37.2631014686576,38.1264711628116));
#27824=CARTESIAN_POINT('Ctrl Pts',(-41.7981279794346,37.2631014686576,38.1264711628116));
#27825=CARTESIAN_POINT('Ctrl Pts',(-41.7981279794346,37.2631014686576,38.1264711628116));
#27826=CARTESIAN_POINT('Ctrl Pts',(-41.7981279794346,37.2631014686576,38.1264711628116));
#27827=CARTESIAN_POINT('Ctrl Pts',(-41.7981279794346,37.2631014686576,38.1264711628116));
#27828=CARTESIAN_POINT('Ctrl Pts',(-41.7981279794346,37.2631014686576,38.1264711628116));
#27829=CARTESIAN_POINT('Ctrl Pts',(-41.7981279794346,37.2631014686576,38.1264711628116));
#27830=CARTESIAN_POINT('Ctrl Pts',(-41.7981279794346,37.2631014686576,38.1264711628116));
#27831=CARTESIAN_POINT('Ctrl Pts',(-41.7981279794346,37.2631014686576,38.1264711628116));
#27832=CARTESIAN_POINT('Ctrl Pts',(-41.7981279794346,37.2631014686576,38.1264711628116));
#27833=CARTESIAN_POINT('Ctrl Pts',(-41.7981279794346,37.2631014686576,38.1264711628116));
#27834=CARTESIAN_POINT('Ctrl Pts',(-41.7981279794346,37.2631014686576,38.1264711628116));
#27835=CARTESIAN_POINT('Ctrl Pts',(-41.7981279794346,37.2631014686576,38.1264711628116));
#27836=CARTESIAN_POINT('Ctrl Pts',(-41.7981279794346,37.2631014686576,38.1264711628116));
#27837=CARTESIAN_POINT('Ctrl Pts',(-41.7981279794346,37.2631014686576,38.1264711628116));
#27838=CARTESIAN_POINT('Ctrl Pts',(-41.7981279794346,37.2631014686576,38.1264711628116));
#27839=CARTESIAN_POINT('Ctrl Pts',(-41.7981279794346,37.2631014686576,38.1264711628116));
#27840=CARTESIAN_POINT('Ctrl Pts',(-41.7981279794346,37.2631014686576,38.1264711628116));
#27841=CARTESIAN_POINT('Ctrl Pts',(-41.7960245110197,37.2635554058993,38.1291218701799));
#27842=CARTESIAN_POINT('Ctrl Pts',(-41.7962311144902,37.2637489024678,38.1292476999627));
#27843=CARTESIAN_POINT('Ctrl Pts',(-41.7964377179608,37.2639423990362,38.1293735297455));
#27844=CARTESIAN_POINT('Ctrl Pts',(-41.7966443214313,37.2641358956046,38.1294993595282));
#27845=CARTESIAN_POINT('Ctrl Pts',(-41.7968509249018,37.264329392173,38.129625189311));
#27846=CARTESIAN_POINT('Ctrl Pts',(-41.7970575283723,37.2645228887414,38.1297510190938));
#27847=CARTESIAN_POINT('Ctrl Pts',(-41.7972641318428,37.2647163853098,38.1298768488765));
#27848=CARTESIAN_POINT('Ctrl Pts',(-41.7974707353134,37.2649098818782,38.1300026786593));
#27849=CARTESIAN_POINT('Ctrl Pts',(-41.7976773387839,37.2651033784466,38.1301285084421));
#27850=CARTESIAN_POINT('Ctrl Pts',(-41.7978839422544,37.265296875015,38.1302543382248));
#27851=CARTESIAN_POINT('Ctrl Pts',(-41.7980905457249,37.2654903715834,38.1303801680076));
#27852=CARTESIAN_POINT('Ctrl Pts',(-41.7982971491955,37.2656838681519,38.1305059977904));
#27853=CARTESIAN_POINT('Ctrl Pts',(-41.798503752666,37.2658773647203,38.1306318275731));
#27854=CARTESIAN_POINT('Ctrl Pts',(-41.7987103561365,37.2660708612887,38.1307576573559));
#27855=CARTESIAN_POINT('Ctrl Pts',(-41.798916959607,37.2662643578571,38.1308834871387));
#27856=CARTESIAN_POINT('Ctrl Pts',(-41.7991235630775,37.2664578544255,38.1310093169214));
#27857=CARTESIAN_POINT('Ctrl Pts',(-41.7993301665481,37.2666513509939,38.1311351467042));
#27858=CARTESIAN_POINT('Ctrl Pts',(-41.7995367700186,37.2668448475623,38.131260976487));
#27859=CARTESIAN_POINT('Ctrl Pts',(-41.7997433734891,37.2670383441307,38.1313868062697));
#27860=CARTESIAN_POINT('Ctrl Pts',(-41.7999499769596,37.2672318406991,38.1315126360525));
#27861=CARTESIAN_POINT('Ctrl Pts',(-41.8001565804302,37.2674253372675,38.1316384658353));
#27862=CARTESIAN_POINT('Ctrl Pts',(-41.8003631839007,37.2676188338359,38.131764295618));
#27863=CARTESIAN_POINT('Ctrl Pts',(-41.8005697873712,37.2678123304043,38.1318901254008));
#27864=CARTESIAN_POINT('Ctrl Pts',(-41.8007763908417,37.2680058269728,38.1320159551836));
#27865=CARTESIAN_POINT('Ctrl Pts',(-41.8009829943122,37.2681993235412,38.1321417849663));
#27866=CARTESIAN_POINT('Ctrl Pts',(-41.8011895977828,37.2683928201096,38.1322676147491));
#27867=CARTESIAN_POINT('Ctrl Pts',(-41.8013962012533,37.268586316678,38.1323934445319));
#27868=CARTESIAN_POINT('Ctrl Pts',(-41.8016028047238,37.2687798132464,38.1325192743146));
#27869=CARTESIAN_POINT('Ctrl Pts',(-41.8018094081943,37.2689733098148,38.1326451040974));
#27870=CARTESIAN_POINT('Ctrl Pts',(-41.8020160116648,37.2691668063832,38.1327709338802));
#27871=CARTESIAN_POINT('Ctrl Pts',(-41.8022226151354,37.2693603029516,38.1328967636629));
#27872=CARTESIAN_POINT('Ctrl Pts',(-41.8024292186059,37.26955379952,38.1330225934457));
#27873=CARTESIAN_POINT('Ctrl Pts',(-41.8026358220764,37.2697472960884,38.1331484232285));
#27874=CARTESIAN_POINT('Ctrl Pts',(-41.8028424255469,37.2699407926569,38.1332742530112));
#27875=CARTESIAN_POINT('Ctrl Pts',(-41.8030490290175,37.2701342892253,38.133400082794));
#27876=CARTESIAN_POINT('Ctrl Pts',(-41.803255632488,37.2703277857937,38.1335259125768));
#27877=CARTESIAN_POINT('Ctrl Pts',(-41.8034622359585,37.2705212823621,38.1336517423595));
#27878=CARTESIAN_POINT('Ctrl Pts',(-41.803668839429,37.2707147789305,38.1337775721423));
#27879=CARTESIAN_POINT('Ctrl Pts',(-41.8038754428995,37.2709082754989,38.1339034019251));
#27880=CARTESIAN_POINT('Ctrl Pts',(-41.8040820463701,37.2711017720673,38.1340292317078));
#27881=CARTESIAN_POINT('Ctrl Pts',(-41.8042886498406,37.2712952686357,38.1341550614906));
#27882=CARTESIAN_POINT('Ctrl Pts',(-41.8044952533111,37.2714887652041,38.1342808912734));
#27883=CARTESIAN_POINT('Ctrl Pts',(-41.8047018567816,37.2716822617725,38.1344067210561));
#27884=CARTESIAN_POINT('Ctrl Pts',(-41.8049084602521,37.2718757583409,38.1345325508389));
#27885=CARTESIAN_POINT('Ctrl Pts',(-41.8051150637227,37.2720692549094,38.1346583806217));
#27886=CARTESIAN_POINT('Ctrl Pts',(-41.8053216671932,37.2722627514778,38.1347842104044));
#27887=CARTESIAN_POINT('Ctrl Pts',(-41.805528454281,37.2724564200148,38.1349101520175));
#27888=CARTESIAN_POINT('Ctrl Pts',(-41.8057352413689,37.2726500885519,38.1350360936305));
#27889=CARTESIAN_POINT('Ctrl Pts',(-41.8059420284567,37.272843757089,38.1351620352436));
#27890=CARTESIAN_POINT('Ctrl Pts',(-41.7939210565382,37.2640093183082,38.1317725928578));
#27891=CARTESIAN_POINT('Ctrl Pts',(-41.7943397763188,37.2644044471742,38.1320324388456));
#27892=CARTESIAN_POINT('Ctrl Pts',(-41.7947584589863,37.2647996421852,38.1322922440548));
#27893=CARTESIAN_POINT('Ctrl Pts',(-41.7951771045444,37.2651949033453,38.1325520084888));
#27894=CARTESIAN_POINT('Ctrl Pts',(-41.7955957501026,37.2655901645054,38.1328117729228));
#27895=CARTESIAN_POINT('Ctrl Pts',(-41.7960143585513,37.2659854918146,38.1330714965815));
#27896=CARTESIAN_POINT('Ctrl Pts',(-41.7964329298944,37.2663808852769,38.1333311794681));
#27897=CARTESIAN_POINT('Ctrl Pts',(-41.7968515012375,37.2667762787392,38.1335908623546));
#27898=CARTESIAN_POINT('Ctrl Pts',(-41.7972700354749,37.2671717383546,38.133850504469));
#27899=CARTESIAN_POINT('Ctrl Pts',(-41.7976885326102,37.2675672641272,38.1341101058145));
#27900=CARTESIAN_POINT('Ctrl Pts',(-41.7981070297456,37.2679627898998,38.1343697071599));
#27901=CARTESIAN_POINT('Ctrl Pts',(-41.7985254897789,37.2683583818297,38.1346292677364));
#27902=CARTESIAN_POINT('Ctrl Pts',(-41.7989439127138,37.2687540399209,38.134888787547));
#27903=CARTESIAN_POINT('Ctrl Pts',(-41.7993623356487,37.2691496980122,38.1351483073576));
#27904=CARTESIAN_POINT('Ctrl Pts',(-41.7997807214852,37.2695454222648,38.1354077864023));
#27905=CARTESIAN_POINT('Ctrl Pts',(-41.800199070227,37.269941212683,38.1356672246842));
#27906=CARTESIAN_POINT('Ctrl Pts',(-41.8006174189687,37.2703370031012,38.1359266629662));
#27907=CARTESIAN_POINT('Ctrl Pts',(-41.8010357306157,37.2707328596848,38.1361860604855));
#27908=CARTESIAN_POINT('Ctrl Pts',(-41.8014540051714,37.2711287824383,38.136445417245));
#27909=CARTESIAN_POINT('Ctrl Pts',(-41.8018722797272,37.2715247051917,38.1367047740046));
#27910=CARTESIAN_POINT('Ctrl Pts',(-41.8022905171918,37.2719206941149,38.1369640900045));
#27911=CARTESIAN_POINT('Ctrl Pts',(-41.8027087175689,37.2723167492119,38.1372233652478));
#27912=CARTESIAN_POINT('Ctrl Pts',(-41.8031269179459,37.272712804309,38.1374826404911));
#27913=CARTESIAN_POINT('Ctrl Pts',(-41.8035450812354,37.2731089255801,38.1377418749778));
#27914=CARTESIAN_POINT('Ctrl Pts',(-41.8039632074408,37.2735051130292,38.1380010687111));
#27915=CARTESIAN_POINT('Ctrl Pts',(-41.8043813336463,37.2739013004784,38.1382602624443));
#27916=CARTESIAN_POINT('Ctrl Pts',(-41.8047994227677,37.2742975541059,38.138519415424));
#27917=CARTESIAN_POINT('Ctrl Pts',(-41.8052174748088,37.2746938739157,38.1387785276532));
#27918=CARTESIAN_POINT('Ctrl Pts',(-41.8056355268498,37.2750901937255,38.1390376398824));
#27919=CARTESIAN_POINT('Ctrl Pts',(-41.8060535418103,37.2754865797179,38.1392967113611));
#27920=CARTESIAN_POINT('Ctrl Pts',(-41.8064715196939,37.275883031897,38.1395557420923));
#27921=CARTESIAN_POINT('Ctrl Pts',(-41.8068894975776,37.276279484076,38.1398147728236));
#27922=CARTESIAN_POINT('Ctrl Pts',(-41.8073074383844,37.2766760024418,38.1400737628074));
#27923=CARTESIAN_POINT('Ctrl Pts',(-41.8077253421178,37.2770725869988,38.1403327120467));
#27924=CARTESIAN_POINT('Ctrl Pts',(-41.8081432458511,37.2774691715558,38.140591661286));
#27925=CARTESIAN_POINT('Ctrl Pts',(-41.8085611125111,37.2778658223038,38.1408505697809));
#27926=CARTESIAN_POINT('Ctrl Pts',(-41.8089789421013,37.2782625392472,38.1411094375343));
#27927=CARTESIAN_POINT('Ctrl Pts',(-41.8093967716914,37.2786592561906,38.1413683052878));
#27928=CARTESIAN_POINT('Ctrl Pts',(-41.8098145642117,37.2790560393296,38.1416271322997));
#27929=CARTESIAN_POINT('Ctrl Pts',(-41.8102323196656,37.2794528886683,38.1418859185732));
#27930=CARTESIAN_POINT('Ctrl Pts',(-41.8106500751195,37.2798497380071,38.1421447048466));
#27931=CARTESIAN_POINT('Ctrl Pts',(-41.8110677935071,37.2802466535456,38.1424034503816));
#27932=CARTESIAN_POINT('Ctrl Pts',(-41.8114854748317,37.2806436352884,38.142662155181));
#27933=CARTESIAN_POINT('Ctrl Pts',(-41.8119031561564,37.2810406170312,38.1429208599804));
#27934=CARTESIAN_POINT('Ctrl Pts',(-41.8123208004182,37.2814376649782,38.1431795240443));
#27935=CARTESIAN_POINT('Ctrl Pts',(-41.8127384076205,37.2818347791339,38.1434381473755));
#27936=CARTESIAN_POINT('Ctrl Pts',(-41.8131563859682,37.2822322462219,38.1436970005564));
#27937=CARTESIAN_POINT('Ctrl Pts',(-41.8135743271905,37.2826297796363,38.1439558129322));
#27938=CARTESIAN_POINT('Ctrl Pts',(-41.813992231291,37.2830273793816,38.1442145845059));
#27939=CARTESIAN_POINT('Ctrl Pts',(-41.79181757419,37.2644632803828,38.1344232849166));
#27940=CARTESIAN_POINT('Ctrl Pts',(-41.7924539645127,37.2650685630173,38.1348259073185));
#27941=CARTESIAN_POINT('Ctrl Pts',(-41.7930902341437,37.2656740607558,38.1352283971087));
#27942=CARTESIAN_POINT('Ctrl Pts',(-41.7937263829759,37.2662797734963,38.1356307542194));
#27943=CARTESIAN_POINT('Ctrl Pts',(-41.7943625318081,37.2668854862368,38.1360331113302));
#27944=CARTESIAN_POINT('Ctrl Pts',(-41.7949985598417,37.2674914139794,38.1364353357616));
#27945=CARTESIAN_POINT('Ctrl Pts',(-41.7956344669696,37.2680975566223,38.1368374274459));
#27946=CARTESIAN_POINT('Ctrl Pts',(-41.7962703740977,37.2687036992651,38.1372395191303));
#27947=CARTESIAN_POINT('Ctrl Pts',(-41.7969061603201,37.2693100568083,38.1376414780677));
#27948=CARTESIAN_POINT('Ctrl Pts',(-41.7975418255301,37.2699166291498,38.1380433041906));
#27949=CARTESIAN_POINT('Ctrl Pts',(-41.7981774907402,37.2705232014914,38.1384451303135));
#27950=CARTESIAN_POINT('Ctrl Pts',(-41.7988130349378,37.2711299886313,38.1388468236219));
#27951=CARTESIAN_POINT('Ctrl Pts',(-41.7994484580163,37.2717369904676,38.1392483840483));
#27952=CARTESIAN_POINT('Ctrl Pts',(-41.8000838810948,37.2723439923039,38.1396499444747));
#27953=CARTESIAN_POINT('Ctrl Pts',(-41.8007191830542,37.2729512088367,38.140051372019));
#27954=CARTESIAN_POINT('Ctrl Pts',(-41.8013543637875,37.2735586399639,38.1404526666139));
#27955=CARTESIAN_POINT('Ctrl Pts',(-41.8019895445209,37.2741660710911,38.1408539612088));
#27956=CARTESIAN_POINT('Ctrl Pts',(-41.8026246040285,37.2747737168126,38.1412551228543));
#27957=CARTESIAN_POINT('Ctrl Pts',(-41.8032595422033,37.2753815770265,38.1416561514829));
#27958=CARTESIAN_POINT('Ctrl Pts',(-41.8038944803782,37.2759894372404,38.1420571801114));
#27959=CARTESIAN_POINT('Ctrl Pts',(-41.8045292972204,37.2765975119466,38.1424580757232));
#27960=CARTESIAN_POINT('Ctrl Pts',(-41.8051639926234,37.2772058010429,38.1428588382507));
#27961=CARTESIAN_POINT('Ctrl Pts',(-41.8057986880264,37.2778140901392,38.1432596007782));
#27962=CARTESIAN_POINT('Ctrl Pts',(-41.80643326199,37.2784225936257,38.1436602302214));
#27963=CARTESIAN_POINT('Ctrl Pts',(-41.8070677144078,37.2790313114001,38.1440607265132));
#27964=CARTESIAN_POINT('Ctrl Pts',(-41.8077021668256,37.2796400291744,38.1444612228049));
#27965=CARTESIAN_POINT('Ctrl Pts',(-41.8083364976974,37.2802489612367,38.1448615859451));
#27966=CARTESIAN_POINT('Ctrl Pts',(-41.8089707069168,37.2808581074845,38.1452618158665));
#27967=CARTESIAN_POINT('Ctrl Pts',(-41.8096049161361,37.2814672537324,38.1456620457879));
#27968=CARTESIAN_POINT('Ctrl Pts',(-41.810239003703,37.2820766141657,38.1460621424905));
#27969=CARTESIAN_POINT('Ctrl Pts',(-41.8108729695109,37.2826861886823,38.1464621059071));
#27970=CARTESIAN_POINT('Ctrl Pts',(-41.8115069353187,37.2832957631989,38.1468620693236));
#27971=CARTESIAN_POINT('Ctrl Pts',(-41.8121407793675,37.2839055517988,38.1472618994541));
#27972=CARTESIAN_POINT('Ctrl Pts',(-41.8127745015508,37.2845155543793,38.1476615962314));
#27973=CARTESIAN_POINT('Ctrl Pts',(-41.8134082237341,37.2851255569598,38.1480612930087));
#27974=CARTESIAN_POINT('Ctrl Pts',(-41.8140418240518,37.285735773521,38.1484608564328));
#27975=CARTESIAN_POINT('Ctrl Pts',(-41.8146753023975,37.2863462039604,38.1488602864366));
#27976=CARTESIAN_POINT('Ctrl Pts',(-41.8153087807433,37.2869566343999,38.1492597164403));
#27977=CARTESIAN_POINT('Ctrl Pts',(-41.815942137117,37.2875672787175,38.1496590130237));
#27978=CARTESIAN_POINT('Ctrl Pts',(-41.8165753714124,37.2881781368108,38.1500581761196));
#27979=CARTESIAN_POINT('Ctrl Pts',(-41.8172086057077,37.288788994904,38.1504573392156));
#27980=CARTESIAN_POINT('Ctrl Pts',(-41.8178417179246,37.2894000667729,38.1508563688241));
#27981=CARTESIAN_POINT('Ctrl Pts',(-41.8184747079568,37.2900113523147,38.1512552648781));
#27982=CARTESIAN_POINT('Ctrl Pts',(-41.8191076979889,37.2906226378565,38.1516541609321));
#27983=CARTESIAN_POINT('Ctrl Pts',(-41.8197405658363,37.2912341370712,38.1520529234316));
#27984=CARTESIAN_POINT('Ctrl Pts',(-41.8203733113925,37.291845849856,38.1524515523097));
#27985=CARTESIAN_POINT('Ctrl Pts',(-41.8210066192967,37.2924581062961,38.1528505354662));
#27986=CARTESIAN_POINT('Ctrl Pts',(-41.8216398046923,37.2930705766862,38.1532493847636));
#27987=CARTESIAN_POINT('Ctrl Pts',(-41.8222728674726,37.2936832609232,38.1536481001348));
#27988=CARTESIAN_POINT('Ctrl Pts',(-41.7912917036029,37.2645767709014,38.1350859579313));
#27989=CARTESIAN_POINT('Ctrl Pts',(-41.7919825115612,37.2652345919781,38.1355242744368));
#27990=CARTESIAN_POINT('Ctrl Pts',(-41.792673177933,37.2658926653985,38.1359624353721));
#27991=CARTESIAN_POINT('Ctrl Pts',(-41.7933637025837,37.2665509910341,38.1364004406521));
#27992=CARTESIAN_POINT('Ctrl Pts',(-41.7940542272345,37.2672093166697,38.1368384459321));
#27993=CARTESIAN_POINT('Ctrl Pts',(-41.7947446101643,37.2678678945206,38.1372762955566));
#27994=CARTESIAN_POINT('Ctrl Pts',(-41.7954348512385,37.2685267244587,38.1377139894404));
#27995=CARTESIAN_POINT('Ctrl Pts',(-41.7961250923127,37.2691855543967,38.1381516833243));
#27996=CARTESIAN_POINT('Ctrl Pts',(-41.7968151915314,37.2698446364218,38.1385892214674));
#27997=CARTESIAN_POINT('Ctrl Pts',(-41.7975051487601,37.2705039704055,38.1390266037847));
#27998=CARTESIAN_POINT('Ctrl Pts',(-41.7981951059888,37.2711633043892,38.139463986102));
#27999=CARTESIAN_POINT('Ctrl Pts',(-41.7988849212276,37.2718228903316,38.1399012125933));
#28000=CARTESIAN_POINT('Ctrl Pts',(-41.799574594342,37.2724827281042,38.1403382831736));
#28001=CARTESIAN_POINT('Ctrl Pts',(-41.8002642674564,37.2731425658768,38.1407753537539));
#28002=CARTESIAN_POINT('Ctrl Pts',(-41.8009537984464,37.2738026554797,38.1412122684232));
#28003=CARTESIAN_POINT('Ctrl Pts',(-41.8016431871777,37.2744629967841,38.1416490270963));
#28004=CARTESIAN_POINT('Ctrl Pts',(-41.802332575909,37.2751233380886,38.1420857857694));
#28005=CARTESIAN_POINT('Ctrl Pts',(-41.8030218223817,37.2757839310946,38.1425223884465));
#28006=CARTESIAN_POINT('Ctrl Pts',(-41.8037109264613,37.2764447756736,38.1429588350423));
#28007=CARTESIAN_POINT('Ctrl Pts',(-41.8044000305409,37.2771056202526,38.1433952816381));
#28008=CARTESIAN_POINT('Ctrl Pts',(-41.8050889922276,37.2777667164045,38.1438315721529));
#28009=CARTESIAN_POINT('Ctrl Pts',(-41.805777811387,37.2784280640007,38.1442677065014));
#28010=CARTESIAN_POINT('Ctrl Pts',(-41.8064666305465,37.2790894115968,38.1447038408499));
#28011=CARTESIAN_POINT('Ctrl Pts',(-41.8071553071787,37.2797510106372,38.1451398190323));
#28012=CARTESIAN_POINT('Ctrl Pts',(-41.8078438411495,37.2804128609928,38.1455756409637));
#28013=CARTESIAN_POINT('Ctrl Pts',(-41.8085323751204,37.2810747113485,38.1460114628951));
#28014=CARTESIAN_POINT('Ctrl Pts',(-41.8092207664298,37.2817368130194,38.1464471285754));
#28015=CARTESIAN_POINT('Ctrl Pts',(-41.8099090149438,37.2823991658767,38.1468826379199));
#28016=CARTESIAN_POINT('Ctrl Pts',(-41.8105972634578,37.283061518734,38.1473181472643));
#28017=CARTESIAN_POINT('Ctrl Pts',(-41.8112853691762,37.2837241227777,38.1477535002729));
#28018=CARTESIAN_POINT('Ctrl Pts',(-41.8119733319651,37.2843869778787,38.1481886968607));
#28019=CARTESIAN_POINT('Ctrl Pts',(-41.812661294754,37.2850498329797,38.1486238934486));
#28020=CARTESIAN_POINT('Ctrl Pts',(-41.8133491146133,37.285712939138,38.1490589336158));
#28021=CARTESIAN_POINT('Ctrl Pts',(-41.814036791409,37.2863762962244,38.1494938172776));
#28022=CARTESIAN_POINT('Ctrl Pts',(-41.8147244682048,37.2870396533108,38.1499287009394));
#28023=CARTESIAN_POINT('Ctrl Pts',(-41.815412001937,37.2877032613253,38.1503634280958));
#28024=CARTESIAN_POINT('Ctrl Pts',(-41.8160993924716,37.2883671201388,38.1507979986621));
#28025=CARTESIAN_POINT('Ctrl Pts',(-41.8167867830062,37.2890309789523,38.1512325692284));
#28026=CARTESIAN_POINT('Ctrl Pts',(-41.8174740303434,37.2896950885646,38.1516669832047));
#28027=CARTESIAN_POINT('Ctrl Pts',(-41.8181611343491,37.2903594488464,38.1521012405063));
#28028=CARTESIAN_POINT('Ctrl Pts',(-41.8188482383547,37.2910238091284,38.1525354978078));
#28029=CARTESIAN_POINT('Ctrl Pts',(-41.819535199029,37.2916884200798,38.1529695984347));
#28030=CARTESIAN_POINT('Ctrl Pts',(-41.820222016238,37.2923532815713,38.1534035423024));
#28031=CARTESIAN_POINT('Ctrl Pts',(-41.820908833447,37.2930181430628,38.15383748617));
#28032=CARTESIAN_POINT('Ctrl Pts',(-41.8215955071908,37.2936832550944,38.1542712732784));
#28033=CARTESIAN_POINT('Ctrl Pts',(-41.8222820373355,37.2943486175366,38.1547049035432));
#28034=CARTESIAN_POINT('Ctrl Pts',(-41.8229691776288,37.2950145713147,38.1551389191936));
#28035=CARTESIAN_POINT('Ctrl Pts',(-41.8236561740677,37.2956807759487,38.1555727777215));
#28036=CARTESIAN_POINT('Ctrl Pts',(-41.8243430265181,37.2963472313086,38.156006479042));
#28037=CARTESIAN_POINT('Ctrl Pts',(-41.7907658588839,37.2646902153166,38.1357486593688));
#28038=CARTESIAN_POINT('Ctrl Pts',(-41.7915114300167,37.2654011073895,38.1362232160579));
#28039=CARTESIAN_POINT('Ctrl Pts',(-41.7922568357581,37.2661122942323,38.136697591021));
#28040=CARTESIAN_POINT('Ctrl Pts',(-41.7930020759386,37.2668237756833,38.1371717841502));
#28041=CARTESIAN_POINT('Ctrl Pts',(-41.7937473161191,37.2675352571344,38.1376459772793));
#28042=CARTESIAN_POINT('Ctrl Pts',(-41.7944923907387,37.2682470331936,38.1381199885747));
#28043=CARTESIAN_POINT('Ctrl Pts',(-41.7952372996279,37.2689591036991,38.1385938179283));
#28044=CARTESIAN_POINT('Ctrl Pts',(-41.7959822085171,37.2696711742047,38.1390676472819));
#28045=CARTESIAN_POINT('Ctrl Pts',(-41.7967269516758,37.2703835391565,38.1395412946939));
#28046=CARTESIAN_POINT('Ctrl Pts',(-41.7974715289348,37.2710961983927,38.1400147600566));
#28047=CARTESIAN_POINT('Ctrl Pts',(-41.7982161061936,37.2718088576289,38.1404882254192));
#28048=CARTESIAN_POINT('Ctrl Pts',(-41.7989605175528,37.2725218111494,38.1409615087326));
#28049=CARTESIAN_POINT('Ctrl Pts',(-41.7997047628426,37.2732350587921,38.1414346098889));
#28050=CARTESIAN_POINT('Ctrl Pts',(-41.8004490081325,37.2739483064348,38.1419077110453));
#28051=CARTESIAN_POINT('Ctrl Pts',(-41.8011930873532,37.2746618481997,38.1423806300447));
#28052=CARTESIAN_POINT('Ctrl Pts',(-41.8019370003355,37.2753756839244,38.1428533667796));
#28053=CARTESIAN_POINT('Ctrl Pts',(-41.8026809133178,37.2760895196491,38.1433261035146));
#28054=CARTESIAN_POINT('Ctrl Pts',(-41.8034246600615,37.2768036493338,38.143798657985));
#28055=CARTESIAN_POINT('Ctrl Pts',(-41.8041682403976,37.277518072816,38.1442710300836));
#28056=CARTESIAN_POINT('Ctrl Pts',(-41.8049118207338,37.2782324962982,38.1447434021821));
#28057=CARTESIAN_POINT('Ctrl Pts',(-41.8056552346622,37.2789472135778,38.1452155919088));
#28058=CARTESIAN_POINT('Ctrl Pts',(-41.8063984820139,37.2796622244925,38.1456875991561));
#28059=CARTESIAN_POINT('Ctrl Pts',(-41.8071417293656,37.280377235407,38.1461596064035));
#28060=CARTESIAN_POINT('Ctrl Pts',(-41.8078848101404,37.2810925399566,38.1466314311716));
#28061=CARTESIAN_POINT('Ctrl Pts',(-41.8086277241695,37.2818081379785,38.1471030733532));
#28062=CARTESIAN_POINT('Ctrl Pts',(-41.8093706381985,37.2825237360004,38.1475747155347));
#28063=CARTESIAN_POINT('Ctrl Pts',(-41.8101133854818,37.2832396274945,38.1480461751297));
#28064=CARTESIAN_POINT('Ctrl Pts',(-41.8108559658502,37.2839558122982,38.1485174520309));
#28065=CARTESIAN_POINT('Ctrl Pts',(-41.8115985462185,37.2846719971018,38.1489887289321));
#28066=CARTESIAN_POINT('Ctrl Pts',(-41.8123409596722,37.2853884752149,38.1494598231396));
#28067=CARTESIAN_POINT('Ctrl Pts',(-41.8130832060421,37.2861052464746,38.1499307345462));
#28068=CARTESIAN_POINT('Ctrl Pts',(-41.8138254524119,37.2868220177343,38.1504016459528));
#28069=CARTESIAN_POINT('Ctrl Pts',(-41.8145675316981,37.2875390821405,38.1508723745586));
#28070=CARTESIAN_POINT('Ctrl Pts',(-41.8153094437317,37.2882564395303,38.1513429202564));
#28071=CARTESIAN_POINT('Ctrl Pts',(-41.8160513557654,37.28897379692,38.1518134659542));
#28072=CARTESIAN_POINT('Ctrl Pts',(-41.8167931005464,37.2896914472933,38.1522838287441));
#28073=CARTESIAN_POINT('Ctrl Pts',(-41.8175346779063,37.2904093904868,38.1527540085193));
#28074=CARTESIAN_POINT('Ctrl Pts',(-41.8182762552661,37.2911273336803,38.1532241882944));
#28075=CARTESIAN_POINT('Ctrl Pts',(-41.8190176652046,37.2918455696942,38.1536941850546));
#28076=CARTESIAN_POINT('Ctrl Pts',(-41.8197589075531,37.292564098365,38.1541639986931));
#28077=CARTESIAN_POINT('Ctrl Pts',(-41.8205001499017,37.2932826270358,38.1546338123316));
#28078=CARTESIAN_POINT('Ctrl Pts',(-41.8212412246603,37.2940014483635,38.1551034428484));
#28079=CARTESIAN_POINT('Ctrl Pts',(-41.8219821316603,37.2947205621849,38.1555728901367));
#28080=CARTESIAN_POINT('Ctrl Pts',(-41.8227230386603,37.2954396760062,38.1560423374249));
#28081=CARTESIAN_POINT('Ctrl Pts',(-41.8234637779018,37.2961590823209,38.1565116014848));
#28082=CARTESIAN_POINT('Ctrl Pts',(-41.8242043492162,37.2968787809657,38.1569806822093));
#28083=CARTESIAN_POINT('Ctrl Pts',(-41.8249455787079,37.2975991192373,38.1574501798259));
#28084=CARTESIAN_POINT('Ctrl Pts',(-41.8256866399739,37.2983197503587,38.1579194937813));
#28085=CARTESIAN_POINT('Ctrl Pts',(-41.8264275328452,37.2990406741657,38.1583886239685));
#28086=CARTESIAN_POINT('Ctrl Pts',(-41.7902399728789,37.264803733314,38.1364113154429));
#28087=CARTESIAN_POINT('Ctrl Pts',(-41.791040652538,37.2655682301309,38.1369226670485));
#28088=CARTESIAN_POINT('Ctrl Pts',(-41.7918411399332,37.2663330696116,38.1374338074015));
#28089=CARTESIAN_POINT('Ctrl Pts',(-41.7926414348502,37.2670982515513,38.1379447363651));
#28090=CARTESIAN_POINT('Ctrl Pts',(-41.7934417297672,37.2678634334911,38.1384556653286));
#28091=CARTESIAN_POINT('Ctrl Pts',(-41.794241832206,37.2686289578899,38.1389663829027));
#28092=CARTESIAN_POINT('Ctrl Pts',(-41.7950417419526,37.2693948245428,38.1394768889507));
#28093=CARTESIAN_POINT('Ctrl Pts',(-41.795841651699,37.2701606911958,38.1399873949986));
#28094=CARTESIAN_POINT('Ctrl Pts',(-41.7966413687531,37.2709269001031,38.1404976895203));
#28095=CARTESIAN_POINT('Ctrl Pts',(-41.7974408929009,37.2716934510593,38.1410077723793));
#28096=CARTESIAN_POINT('Ctrl Pts',(-41.7982404170486,37.2724600020156,38.1415178552383));
#28097=CARTESIAN_POINT('Ctrl Pts',(-41.7990397482899,37.2732268950209,38.1420277264346));
#28098=CARTESIAN_POINT('Ctrl Pts',(-41.7998388864109,37.2739941298702,38.1425373858316));
#28099=CARTESIAN_POINT('Ctrl Pts',(-41.8006380245318,37.2747613647194,38.1430470452286));
#28100=CARTESIAN_POINT('Ctrl Pts',(-41.8014369695325,37.2755289414123,38.1435564928264));
#28101=CARTESIAN_POINT('Ctrl Pts',(-41.8022357211989,37.2762968597437,38.1440657284886));
#28102=CARTESIAN_POINT('Ctrl Pts',(-41.8030344728653,37.2770647780751,38.1445749641509));
#28103=CARTESIAN_POINT('Ctrl Pts',(-41.8038330311975,37.2778330380449,38.1450839878774));
#28104=CARTESIAN_POINT('Ctrl Pts',(-41.8046313959817,37.2786016394473,38.1455927995322));
#28105=CARTESIAN_POINT('Ctrl Pts',(-41.8054297607659,37.2793702408498,38.146101611187));
#28106=CARTESIAN_POINT('Ctrl Pts',(-41.8062279320023,37.280139183685,38.14661021077));
#28107=CARTESIAN_POINT('Ctrl Pts',(-41.8070259094769,37.2809084677471,38.1471185981449));
#28108=CARTESIAN_POINT('Ctrl Pts',(-41.8078238869517,37.2816777518092,38.1476269855199));
#28109=CARTESIAN_POINT('Ctrl Pts',(-41.8086216706648,37.2824473770983,38.1481351606869));
#28110=CARTESIAN_POINT('Ctrl Pts',(-41.8094192604028,37.2832173434083,38.1486431235099));
#28111=CARTESIAN_POINT('Ctrl Pts',(-41.8102168501408,37.2839873097182,38.1491510863329));
#28112=CARTESIAN_POINT('Ctrl Pts',(-41.8110142459036,37.2847576170491,38.1496588368119));
#28113=CARTESIAN_POINT('Ctrl Pts',(-41.8118114474779,37.2855282651947,38.1501663748111));
#28114=CARTESIAN_POINT('Ctrl Pts',(-41.8126086490522,37.2862989133403,38.1506739128102));
#28115=CARTESIAN_POINT('Ctrl Pts',(-41.8134056564379,37.2870699023006,38.1511812383294));
#28116=CARTESIAN_POINT('Ctrl Pts',(-41.8142024694217,37.2878412318693,38.1516883512329));
#28117=CARTESIAN_POINT('Ctrl Pts',(-41.8149992824055,37.288612561438,38.1521954641365));
#28118=CARTESIAN_POINT('Ctrl Pts',(-41.8157959009875,37.289384231615,38.1527023644243));
#28119=CARTESIAN_POINT('Ctrl Pts',(-41.8165923249543,37.2901562421939,38.1532090519608));
#28120=CARTESIAN_POINT('Ctrl Pts',(-41.8173887489211,37.2909282527728,38.1537157394973));
#28121=CARTESIAN_POINT('Ctrl Pts',(-41.8181849782728,37.2917006037534,38.1542222142824));
#28122=CARTESIAN_POINT('Ctrl Pts',(-41.8189810127963,37.2924732949292,38.1547284761806));
#28123=CARTESIAN_POINT('Ctrl Pts',(-41.8197770473197,37.293245986105,38.1552347380787));
#28124=CARTESIAN_POINT('Ctrl Pts',(-41.8205728870149,37.2940190174758,38.15574078709));
#28125=CARTESIAN_POINT('Ctrl Pts',(-41.8213685316688,37.2947923888349,38.1562466230788));
#28126=CARTESIAN_POINT('Ctrl Pts',(-41.8221641763227,37.2955657601939,38.1567524590677));
#28127=CARTESIAN_POINT('Ctrl Pts',(-41.8229596259354,37.2963394715411,38.1572580820341));
#28128=CARTESIAN_POINT('Ctrl Pts',(-41.8237548802939,37.2971135226694,38.1577634918429));
#28129=CARTESIAN_POINT('Ctrl Pts',(-41.8245501346524,37.2978875737977,38.1582689016516));
#28130=CARTESIAN_POINT('Ctrl Pts',(-41.8253451937568,37.298661964707,38.1587740983027));
#28131=CARTESIAN_POINT('Ctrl Pts',(-41.8261400573941,37.2994366951901,38.1592790816607));
#28132=CARTESIAN_POINT('Ctrl Pts',(-41.8269356274607,37.3002121142093,38.1597845138191));
#28133=CARTESIAN_POINT('Ctrl Pts',(-41.8277310017127,37.3009878734061,38.1602897323052));
#28134=CARTESIAN_POINT('Ctrl Pts',(-41.8285261799368,37.3017639725726,38.1607947369835));
#28135=CARTESIAN_POINT('Ctrl Pts',(-41.7899770298764,37.2648604923127,38.1367426434799));
#28136=CARTESIAN_POINT('Ctrl Pts',(-41.7908052637987,37.2656517915016,38.1372723925438));
#28137=CARTESIAN_POINT('Ctrl Pts',(-41.7916332920208,37.2664434573011,38.1378019155918));
#28138=CARTESIAN_POINT('Ctrl Pts',(-41.792461114306,37.2672354894853,38.1383312124726));
#28139=CARTESIAN_POINT('Ctrl Pts',(-41.7932889365913,37.2680275216694,38.1388605093533));
#28140=CARTESIAN_POINT('Ctrl Pts',(-41.7941165529397,37.268819920238,38.1393895800668));
#28141=CARTESIAN_POINT('Ctrl Pts',(-41.7949439631148,37.2696126849648,38.1399184244618));
#28142=CARTESIAN_POINT('Ctrl Pts',(-41.79577137329,37.2704054496914,38.1404472688569));
#28143=CARTESIAN_POINT('Ctrl Pts',(-41.7965985772918,37.2711985805763,38.1409758869336));
#28144=CARTESIAN_POINT('Ctrl Pts',(-41.7974255748839,37.2719920773926,38.1415042785407));
#28145=CARTESIAN_POINT('Ctrl Pts',(-41.7982525724761,37.2727855742089,38.1420326701479));
#28146=CARTESIAN_POINT('Ctrl Pts',(-41.7990793636585,37.2735794369567,38.1425608352856));
#28147=CARTESIAN_POINT('Ctrl Pts',(-41.799905948195,37.2743736654092,38.143088773803));
#28148=CARTESIAN_POINT('Ctrl Pts',(-41.8007325327315,37.2751678938616,38.1436167123203));
#28149=CARTESIAN_POINT('Ctrl Pts',(-41.8015589106221,37.2759624880186,38.1441444242173));
#28150=CARTESIAN_POINT('Ctrl Pts',(-41.8023850816305,37.2767574476534,38.1446719093431));
#28151=CARTESIAN_POINT('Ctrl Pts',(-41.803211252639,37.277552407288,38.145199394469));
#28152=CARTESIAN_POINT('Ctrl Pts',(-41.8040372167654,37.2783477324003,38.1457266528237));
#28153=CARTESIAN_POINT('Ctrl Pts',(-41.8048629737738,37.2791434227629,38.1462536842566));
#28154=CARTESIAN_POINT('Ctrl Pts',(-41.8056887307821,37.2799391131256,38.1467807156895));
#28155=CARTESIAN_POINT('Ctrl Pts',(-41.8065142806723,37.2807351687386,38.1473075202006));
#28156=CARTESIAN_POINT('Ctrl Pts',(-41.8073396232085,37.2815315893745,38.1478340976393));
#28157=CARTESIAN_POINT('Ctrl Pts',(-41.8081649657447,37.2823280100104,38.1483606750781));
#28158=CARTESIAN_POINT('Ctrl Pts',(-41.8089901009269,37.2831247956691,38.1488870254446));
#28159=CARTESIAN_POINT('Ctrl Pts',(-41.8098150285194,37.2839219461231,38.1494131485883));
#28160=CARTESIAN_POINT('Ctrl Pts',(-41.8106399561118,37.2847190965771,38.1499392717321));
#28161=CARTESIAN_POINT('Ctrl Pts',(-41.8114646761145,37.2855166118263,38.1504651676531));
#28162=CARTESIAN_POINT('Ctrl Pts',(-41.8122891882918,37.2863144916429,38.1509908362012));
#28163=CARTESIAN_POINT('Ctrl Pts',(-41.813113700469,37.2871123714595,38.1515165047493));
#28164=CARTESIAN_POINT('Ctrl Pts',(-41.8139380048207,37.2879106158435,38.1520419459243));
#28165=CARTESIAN_POINT('Ctrl Pts',(-41.8147621011115,37.2887092245666,38.1525671595763));
#28166=CARTESIAN_POINT('Ctrl Pts',(-41.8155861974023,37.2895078332898,38.1530923732283));
#28167=CARTESIAN_POINT('Ctrl Pts',(-41.8164100856322,37.2903068063522,38.1536173593573));
#28168=CARTESIAN_POINT('Ctrl Pts',(-41.8172337655656,37.2911061435257,38.154142117813));
#28169=CARTESIAN_POINT('Ctrl Pts',(-41.818057445499,37.2919054806991,38.1546668762689));
#28170=CARTESIAN_POINT('Ctrl Pts',(-41.818880917136,37.2927051819835,38.1551914070515));
#28171=CARTESIAN_POINT('Ctrl Pts',(-41.8197041802412,37.2935052471505,38.1557157100112));
#28172=CARTESIAN_POINT('Ctrl Pts',(-41.8205274433465,37.2943053123173,38.156240012971));
#28173=CARTESIAN_POINT('Ctrl Pts',(-41.82135049792,37.2951057413667,38.1567640881077));
#28174=CARTESIAN_POINT('Ctrl Pts',(-41.8221733437266,37.2959065340698,38.1572879352717));
#28175=CARTESIAN_POINT('Ctrl Pts',(-41.8229961895333,37.296707326773,38.1578117824357));
#28176=CARTESIAN_POINT('Ctrl Pts',(-41.823818826573,37.2975084831298,38.158335401627));
#28177=CARTESIAN_POINT('Ctrl Pts',(-41.8246412546107,37.2983100029116,38.158858792696));
#28178=CARTESIAN_POINT('Ctrl Pts',(-41.8254636826485,37.2991115226933,38.159382183765));
#28179=CARTESIAN_POINT('Ctrl Pts',(-41.8262859016842,37.2999134059,38.1599053467116));
#28180=CARTESIAN_POINT('Ctrl Pts',(-41.8271079114831,37.3007156523024,38.1604282813864));
#28181=CARTESIAN_POINT('Ctrl Pts',(-41.8279306518371,37.3015186116953,38.1609516808156));
#28182=CARTESIAN_POINT('Ctrl Pts',(-41.828753182582,37.3023219349298,38.1614748515671));
#28183=CARTESIAN_POINT('Ctrl Pts',(-41.8295755034826,37.303125621776,38.161997793491));
#28184=CARTESIAN_POINT('Ctrl Pts',(-41.7897141202235,37.2649171918739,38.1370740081602));
#28185=CARTESIAN_POINT('Ctrl Pts',(-41.7905699938216,37.2657354284759,38.1376222923523));
#28186=CARTESIAN_POINT('Ctrl Pts',(-41.7914256475163,37.2665540570026,38.1381703349224));
#28187=CARTESIAN_POINT('Ctrl Pts',(-41.7922810810461,37.267373077204,38.1387181357031));
#28188=CARTESIAN_POINT('Ctrl Pts',(-41.7931365145759,37.2681920974053,38.1392659364838));
#28189=CARTESIAN_POINT('Ctrl Pts',(-41.7939917279408,37.2690115092812,38.139813495475));
#28190=CARTESIAN_POINT('Ctrl Pts',(-41.7948467208796,37.2698313125814,38.1403608125096));
#28191=CARTESIAN_POINT('Ctrl Pts',(-41.7957017138184,37.2706511158816,38.1409081295443));
#28192=CARTESIAN_POINT('Ctrl Pts',(-41.7965564863311,37.271471310606,38.1414552046223));
#28193=CARTESIAN_POINT('Ctrl Pts',(-41.7974110381565,37.2722918965043,38.1420020375765));
#28194=CARTESIAN_POINT('Ctrl Pts',(-41.798265589982,37.2731124824025,38.1425488705307));
#28195=CARTESIAN_POINT('Ctrl Pts',(-41.7991199211203,37.2739334594745,38.1430954613612));
#28196=CARTESIAN_POINT('Ctrl Pts',(-41.7999740313103,37.2747548274695,38.143641809901));
#28197=CARTESIAN_POINT('Ctrl Pts',(-41.8008281415004,37.2755761954645,38.1441881584408));
#28198=CARTESIAN_POINT('Ctrl Pts',(-41.8016820307423,37.2763979543824,38.14473426469));
#28199=CARTESIAN_POINT('Ctrl Pts',(-41.8025356987751,37.2772201039724,38.1452801284816));
#28200=CARTESIAN_POINT('Ctrl Pts',(-41.803389366808,37.2780422535623,38.1458259922732));
#28201=CARTESIAN_POINT('Ctrl Pts',(-41.8042428136318,37.2788647938243,38.1463716136074));
#28202=CARTESIAN_POINT('Ctrl Pts',(-41.8050960389859,37.279687724507,38.1469169923174));
#28203=CARTESIAN_POINT('Ctrl Pts',(-41.80594926434,37.2805106551896,38.1474623710274));
#28204=CARTESIAN_POINT('Ctrl Pts',(-41.8068022682244,37.2813339762931,38.1480075071133));
#28205=CARTESIAN_POINT('Ctrl Pts',(-41.8076550503785,37.2821576875657,38.1485524004085));
#28206=CARTESIAN_POINT('Ctrl Pts',(-41.8085078325325,37.2829813988384,38.1490972937037));
#28207=CARTESIAN_POINT('Ctrl Pts',(-41.8093603929563,37.2838055002803,38.1496419442083));
#28208=CARTESIAN_POINT('Ctrl Pts',(-41.8102127313893,37.2846299916398,38.1501863517559));
#28209=CARTESIAN_POINT('Ctrl Pts',(-41.8110650698224,37.2854544829992,38.1507307593035));
#28210=CARTESIAN_POINT('Ctrl Pts',(-41.8119171862648,37.2862793642763,38.151274923894));
#28211=CARTESIAN_POINT('Ctrl Pts',(-41.8127690804561,37.2871046352189,38.1518188453614));
#28212=CARTESIAN_POINT('Ctrl Pts',(-41.8136209746473,37.2879299061615,38.1523627668288));
#28213=CARTESIAN_POINT('Ctrl Pts',(-41.8144726465877,37.2887555667696,38.1529064451729));
#28214=CARTESIAN_POINT('Ctrl Pts',(-41.8153240960168,37.2895816167912,38.1534498802278));
#28215=CARTESIAN_POINT('Ctrl Pts',(-41.8161755454458,37.2904076668127,38.1539933152827));
#28216=CARTESIAN_POINT('Ctrl Pts',(-41.8170267723638,37.2912341062476,38.1545365070483));
#28217=CARTESIAN_POINT('Ctrl Pts',(-41.8178777765105,37.2920609348435,38.1550794553588));
#28218=CARTESIAN_POINT('Ctrl Pts',(-41.8187287806572,37.2928877634394,38.1556224036692));
#28219=CARTESIAN_POINT('Ctrl Pts',(-41.8195795620327,37.2937149811963,38.1561651085245));
#28220=CARTESIAN_POINT('Ctrl Pts',(-41.8204301203771,37.2945425878614,38.1567075697588));
#28221=CARTESIAN_POINT('Ctrl Pts',(-41.8212806787215,37.2953701945265,38.1572500309931));
#28222=CARTESIAN_POINT('Ctrl Pts',(-41.8221310140348,37.2961981901,38.1577922486064));
#28223=CARTESIAN_POINT('Ctrl Pts',(-41.8229811260573,37.2970265743287,38.1583342224332));
#28224=CARTESIAN_POINT('Ctrl Pts',(-41.8238312380797,37.2978549585575,38.1588761962601));
#28225=CARTESIAN_POINT('Ctrl Pts',(-41.8246811268113,37.2986837314417,38.1594179263003));
#28226=CARTESIAN_POINT('Ctrl Pts',(-41.8255307919925,37.299512892728,38.1599594123885));
#28227=CARTESIAN_POINT('Ctrl Pts',(-41.8263804571736,37.3003420540145,38.1605008984767));
#28228=CARTESIAN_POINT('Ctrl Pts',(-41.8272298988042,37.3011716037031,38.1610421406129));
#28229=CARTESIAN_POINT('Ctrl Pts',(-41.8280791166249,37.3020015415406,38.1615831386317));
#28230=CARTESIAN_POINT('Ctrl Pts',(-41.8289290891818,37.3028322169792,38.1621246174586));
#28231=CARTESIAN_POINT('Ctrl Pts',(-41.8297788375306,37.303663281257,38.162665851734));
#28232=CARTESIAN_POINT('Ctrl Pts',(-41.8306283614115,37.3044947341195,38.1632068412924));
#28233=CARTESIAN_POINT('Ctrl Pts',(-41.7894511722233,37.2649739597797,38.137405330706));
#28234=CARTESIAN_POINT('Ctrl Pts',(-41.7903347721088,37.2658192665273,38.1379722901388));
#28235=CARTESIAN_POINT('Ctrl Pts',(-41.7912181371005,37.2666649919163,38.1385389914788));
#28236=CARTESIAN_POINT('Ctrl Pts',(-41.7921012669095,37.2675111356698,38.1391054345407));
#28237=CARTESIAN_POINT('Ctrl Pts',(-41.7929843967185,37.2683572794234,38.1396718776026));
#28238=CARTESIAN_POINT('Ctrl Pts',(-41.7938672913449,37.2692038415416,38.1402380623863));
#28239=CARTESIAN_POINT('Ctrl Pts',(-41.7947499504998,37.2700508217476,38.1408039887068));
#28240=CARTESIAN_POINT('Ctrl Pts',(-41.7956326096548,37.2708978019536,38.1413699150272));
#28241=CARTESIAN_POINT('Ctrl Pts',(-41.7965150333384,37.2717452002474,38.1419355828845));
#28242=CARTESIAN_POINT('Ctrl Pts',(-41.797397221262,37.2725930163519,38.1425009920934));
#28243=CARTESIAN_POINT('Ctrl Pts',(-41.7982794091856,37.2734408324565,38.1430664013023));
#28244=CARTESIAN_POINT('Ctrl Pts',(-41.7991613613493,37.2742890663717,38.1436315518629));
#28245=CARTESIAN_POINT('Ctrl Pts',(-41.8000430774646,37.2751377178202,38.1441964435905));
#28246=CARTESIAN_POINT('Ctrl Pts',(-41.8009247935799,37.2759863692687,38.1447613353181));
#28247=CARTESIAN_POINT('Ctrl Pts',(-41.8018062736468,37.2768354382506,38.1453259682126));
#28248=CARTESIAN_POINT('Ctrl Pts',(-41.8026875173771,37.2776849244881,38.1458903420894));
#28249=CARTESIAN_POINT('Ctrl Pts',(-41.8035687611075,37.2785344107256,38.1464547159662));
#28250=CARTESIAN_POINT('Ctrl Pts',(-41.8044497685012,37.2793843142188,38.1470188308252));
#28251=CARTESIAN_POINT('Ctrl Pts',(-41.8053305392701,37.2802346346897,38.1475826864821));
#28252=CARTESIAN_POINT('Ctrl Pts',(-41.8062113100392,37.2810849551606,38.148146542139));
#28253=CARTESIAN_POINT('Ctrl Pts',(-41.8070918441834,37.2819356926093,38.1487101385937));
#28254=CARTESIAN_POINT('Ctrl Pts',(-41.8079721414151,37.2827868467574,38.1492734756619));
#28255=CARTESIAN_POINT('Ctrl Pts',(-41.8088524386466,37.2836380009056,38.1498368127301));
#28256=CARTESIAN_POINT('Ctrl Pts',(-41.8097324989656,37.2844895717533,38.1503998904118));
#28257=CARTESIAN_POINT('Ctrl Pts',(-41.8106123220841,37.2853415590221,38.1509627085229));
#28258=CARTESIAN_POINT('Ctrl Pts',(-41.8114921452026,37.2861935462908,38.151525526634));
#28259=CARTESIAN_POINT('Ctrl Pts',(-41.8123717311206,37.2870459499806,38.1520880851745));
#28260=CARTESIAN_POINT('Ctrl Pts',(-41.8132510795506,37.2878987698127,38.1526503839604));
#28261=CARTESIAN_POINT('Ctrl Pts',(-41.8141304279805,37.2887515896449,38.1532126827462));
#28262=CARTESIAN_POINT('Ctrl Pts',(-41.8150095389224,37.2896048256193,38.1537747217775));
#28263=CARTESIAN_POINT('Ctrl Pts',(-41.8158884120887,37.2904584774571,38.1543365008704));
#28264=CARTESIAN_POINT('Ctrl Pts',(-41.816767285255,37.2913121292948,38.1548982799633));
#28265=CARTESIAN_POINT('Ctrl Pts',(-41.8176459206457,37.2921661969958,38.1554597991178));
#28266=CARTESIAN_POINT('Ctrl Pts',(-41.8185243179736,37.2930206802807,38.1560210581504));
#28267=CARTESIAN_POINT('Ctrl Pts',(-41.8194027153014,37.2938751635658,38.1565823171829));
#28268=CARTESIAN_POINT('Ctrl Pts',(-41.8202808745663,37.2947300624348,38.1571433160934));
#28269=CARTESIAN_POINT('Ctrl Pts',(-41.8211587954812,37.2955853766083,38.1577040546985));
#28270=CARTESIAN_POINT('Ctrl Pts',(-41.822036716396,37.2964406907818,38.1582647933035));
#28271=CARTESIAN_POINT('Ctrl Pts',(-41.8229143989609,37.2972964202596,38.1588252716031));
#28272=CARTESIAN_POINT('Ctrl Pts',(-41.8237918428886,37.2981525647621,38.1593854894139));
#28273=CARTESIAN_POINT('Ctrl Pts',(-41.8246692868163,37.2990087092646,38.1599457072248));
#28274=CARTESIAN_POINT('Ctrl Pts',(-41.825546492107,37.2998652687917,38.1605056645469));
#28275=CARTESIAN_POINT('Ctrl Pts',(-41.8264234584738,37.3007222430633,38.1610653611971));
#28276=CARTESIAN_POINT('Ctrl Pts',(-41.8273004248405,37.3015792173349,38.1616250578474));
#28277=CARTESIAN_POINT('Ctrl Pts',(-41.8281771522833,37.302436606351,38.1621844938258));
#28278=CARTESIAN_POINT('Ctrl Pts',(-41.8290536405155,37.3032944098312,38.1627436689494));
#28279=CARTESIAN_POINT('Ctrl Pts',(-41.8299309077201,37.304152975678,38.1633033410358));
#28280=CARTESIAN_POINT('Ctrl Pts',(-41.8308079352887,37.3050119567259,38.1638627518035));
#28281=CARTESIAN_POINT('Ctrl Pts',(-41.831684722934,37.3058713526935,38.1644219010693));
#28282=CARTESIAN_POINT('Ctrl Pts',(-41.7891882242231,37.2650307276855,38.1377366532517));
#28283=CARTESIAN_POINT('Ctrl Pts',(-41.790099550396,37.2659031045788,38.1383222879253));
#28284=CARTESIAN_POINT('Ctrl Pts',(-41.7910106266847,37.2667759268299,38.1389076480353));
#28285=CARTESIAN_POINT('Ctrl Pts',(-41.7919214527729,37.2676491941357,38.1394927333783));
#28286=CARTESIAN_POINT('Ctrl Pts',(-41.7928322788612,37.2685224614414,38.1400778187214));
#28287=CARTESIAN_POINT('Ctrl Pts',(-41.793742854749,37.269396173802,38.1406626292976));
#28288=CARTESIAN_POINT('Ctrl Pts',(-41.7946531801201,37.2702703309138,38.141247164904));
#28289=CARTESIAN_POINT('Ctrl Pts',(-41.7955635054912,37.2711444880256,38.1418317005103));
#28290=CARTESIAN_POINT('Ctrl Pts',(-41.7964735803457,37.2720190898887,38.1424159611466));
#28291=CARTESIAN_POINT('Ctrl Pts',(-41.7973834043674,37.2728941361996,38.1429999466102));
#28292=CARTESIAN_POINT('Ctrl Pts',(-41.7982932283892,37.2737691825104,38.1435839320738));
#28293=CARTESIAN_POINT('Ctrl Pts',(-41.7992028015783,37.2746446732689,38.1441676423646));
#28294=CARTESIAN_POINT('Ctrl Pts',(-41.8001121236188,37.2755206081709,38.14475107728));
#28295=CARTESIAN_POINT('Ctrl Pts',(-41.8010214456594,37.276396543073,38.1453345121953));
#28296=CARTESIAN_POINT('Ctrl Pts',(-41.8019305165514,37.2772729221187,38.1459176717352));
#28297=CARTESIAN_POINT('Ctrl Pts',(-41.8028393359792,37.2781497450038,38.1465005556972));
#28298=CARTESIAN_POINT('Ctrl Pts',(-41.803748155407,37.2790265678889,38.1470834396591));
#28299=CARTESIAN_POINT('Ctrl Pts',(-41.8046567233705,37.2799038346134,38.1476660480431));
#28300=CARTESIAN_POINT('Ctrl Pts',(-41.8055650395544,37.2807815448725,38.1482483806468));
#28301=CARTESIAN_POINT('Ctrl Pts',(-41.8064733557383,37.2816592551316,38.1488307132506));
#28302=CARTESIAN_POINT('Ctrl Pts',(-41.8073814201425,37.2825374089255,38.1494127700742));
#28303=CARTESIAN_POINT('Ctrl Pts',(-41.8082892324516,37.2834160059491,38.1499945509153));
#28304=CARTESIAN_POINT('Ctrl Pts',(-41.8091970447608,37.2842946029728,38.1505763317565));
#28305=CARTESIAN_POINT('Ctrl Pts',(-41.8101046049749,37.2851736432263,38.1511578366154));
#28306=CARTESIAN_POINT('Ctrl Pts',(-41.8110119127788,37.2860531264044,38.1517390652899));
#28307=CARTESIAN_POINT('Ctrl Pts',(-41.8119192205827,37.2869326095824,38.1523202939646));
#28308=CARTESIAN_POINT('Ctrl Pts',(-41.8128262759765,37.287812535685,38.1529012464549));
#28309=CARTESIAN_POINT('Ctrl Pts',(-41.8137330786451,37.2886929044066,38.1534819225593));
#28310=CARTESIAN_POINT('Ctrl Pts',(-41.8146398813137,37.2895732731283,38.1540625986637));
#28311=CARTESIAN_POINT('Ctrl Pts',(-41.8155464312571,37.290454084469,38.1546429983821));
#28312=CARTESIAN_POINT('Ctrl Pts',(-41.8164527281606,37.2913353381229,38.155223121513));
#28313=CARTESIAN_POINT('Ctrl Pts',(-41.8173590250641,37.2922165917768,38.1558032446439));
#28314=CARTESIAN_POINT('Ctrl Pts',(-41.8182650689276,37.2930982877439,38.1563830911873));
#28315=CARTESIAN_POINT('Ctrl Pts',(-41.8191708594366,37.293980425718,38.156962660942));
#28316=CARTESIAN_POINT('Ctrl Pts',(-41.8200766499455,37.2948625636922,38.1575422306965));
#28317=CARTESIAN_POINT('Ctrl Pts',(-41.8209821870999,37.2957451436734,38.1581215236623));
#28318=CARTESIAN_POINT('Ctrl Pts',(-41.8218874705853,37.2966281653551,38.1587005396381));
#28319=CARTESIAN_POINT('Ctrl Pts',(-41.8227927540706,37.2975111870369,38.1592795556139));
#28320=CARTESIAN_POINT('Ctrl Pts',(-41.8236977838869,37.2983946504193,38.1598582945997));
#28321=CARTESIAN_POINT('Ctrl Pts',(-41.82460255972,37.2992785551955,38.1604367563946));
#28322=CARTESIAN_POINT('Ctrl Pts',(-41.825507335553,37.3001624599717,38.1610152181895));
#28323=CARTESIAN_POINT('Ctrl Pts',(-41.8264118574027,37.3010468061417,38.1615934027935));
#28324=CARTESIAN_POINT('Ctrl Pts',(-41.827316124955,37.3019315933985,38.1621713100058));
#28325=CARTESIAN_POINT('Ctrl Pts',(-41.8282203925074,37.3028163806553,38.1627492172181));
#28326=CARTESIAN_POINT('Ctrl Pts',(-41.8291244057623,37.3037016089989,38.1633268470387));
#28327=CARTESIAN_POINT('Ctrl Pts',(-41.8300281644059,37.3045872781219,38.163904199267));
#28328=CARTESIAN_POINT('Ctrl Pts',(-41.8309327262584,37.3054737343768,38.1644820646129));
#28329=CARTESIAN_POINT('Ctrl Pts',(-41.8318370330468,37.3063606321949,38.1650596518729));
#28330=CARTESIAN_POINT('Ctrl Pts',(-41.8327410844565,37.3072479712676,38.1656369608462));
#28331=CARTESIAN_POINT('Ctrl Pts',(-41.7889155657315,37.2650855879526,38.1380738607379));
#28332=CARTESIAN_POINT('Ctrl Pts',(-41.7898542793006,37.2659844101691,38.1386774653796));
#28333=CARTESIAN_POINT('Ctrl Pts',(-41.7907927276113,37.2668837051443,38.1392807785649));
#28334=CARTESIAN_POINT('Ctrl Pts',(-41.7917309103178,37.2677834725466,38.1398838000717));
#28335=CARTESIAN_POINT('Ctrl Pts',(-41.7926690930243,37.2686832399489,38.1404868215784));
#28336=CARTESIAN_POINT('Ctrl Pts',(-41.7936070101265,37.2695834797784,38.1410895514065));
#28337=CARTESIAN_POINT('Ctrl Pts',(-41.7945446612787,37.2704841917031,38.1416919893337));
#28338=CARTESIAN_POINT('Ctrl Pts',(-41.795482312431,37.2713849036278,38.1422944272611));
#28339=CARTESIAN_POINT('Ctrl Pts',(-41.7964196976332,37.2722860876479,38.1428965732875));
#28340=CARTESIAN_POINT('Ctrl Pts',(-41.7973568165398,37.273187743431,38.1434984271912));
#28341=CARTESIAN_POINT('Ctrl Pts',(-41.7982939354465,37.2740893992142,38.1441002810949));
#28342=CARTESIAN_POINT('Ctrl Pts',(-41.7992307880576,37.2749915267605,38.1447018428759));
#28343=CARTESIAN_POINT('Ctrl Pts',(-41.8001673740279,37.2758941257373,38.1453031123123));
#28344=CARTESIAN_POINT('Ctrl Pts',(-41.8011039599982,37.2767967247142,38.1459043817488));
#28345=CARTESIAN_POINT('Ctrl Pts',(-41.8020402793276,37.2776997951217,38.1465053588408));
#28346=CARTESIAN_POINT('Ctrl Pts',(-41.8029763316709,37.2786033366268,38.1471060433667));
#28347=CARTESIAN_POINT('Ctrl Pts',(-41.8039123840142,37.2795068781321,38.1477067278927));
#28348=CARTESIAN_POINT('Ctrl Pts',(-41.8048481693716,37.2804108907349,38.1483071198526));
#28349=CARTESIAN_POINT('Ctrl Pts',(-41.8057836873979,37.2813153741023,38.1489072190253));
#28350=CARTESIAN_POINT('Ctrl Pts',(-41.8067192054243,37.2822198574697,38.1495073181979));
#28351=CARTESIAN_POINT('Ctrl Pts',(-41.8076544561196,37.2831248116015,38.1501071245833));
#28352=CARTESIAN_POINT('Ctrl Pts',(-41.8085894391392,37.2840302361643,38.1507066379602));
#28353=CARTESIAN_POINT('Ctrl Pts',(-41.8095244221589,37.2849356607271,38.1513061513371));
#28354=CARTESIAN_POINT('Ctrl Pts',(-41.8104591375028,37.2858415557209,38.1519053717056));
#28355=CARTESIAN_POINT('Ctrl Pts',(-41.8113935848264,37.2867479208116,38.1525042988449));
#28356=CARTESIAN_POINT('Ctrl Pts',(-41.81232803215,37.2876542859023,38.1531032259841));
#28357=CARTESIAN_POINT('Ctrl Pts',(-41.8132622114533,37.28856112109,38.1537018598942));
#28358=CARTESIAN_POINT('Ctrl Pts',(-41.814196122392,37.2894684260405,38.1543002003542));
#28359=CARTESIAN_POINT('Ctrl Pts',(-41.8151300333306,37.290375730991,38.1548985408142));
#28360=CARTESIAN_POINT('Ctrl Pts',(-41.8160636759047,37.2912835057042,38.1554965878244));
#28361=CARTESIAN_POINT('Ctrl Pts',(-41.8169970497698,37.2921917498456,38.1560943411641));
#28362=CARTESIAN_POINT('Ctrl Pts',(-41.8179304236351,37.2930999939869,38.1566920945039));
#28363=CARTESIAN_POINT('Ctrl Pts',(-41.8188635287915,37.2940087075564,38.1572895541733));
#28364=CARTESIAN_POINT('Ctrl Pts',(-41.8197963648951,37.2949178902191,38.1578867199521));
#28365=CARTESIAN_POINT('Ctrl Pts',(-41.8207292009987,37.2958270728817,38.1584838857309));
#28366=CARTESIAN_POINT('Ctrl Pts',(-41.8216617680496,37.2967367246376,38.1590807576191));
#28367=CARTESIAN_POINT('Ctrl Pts',(-41.8225940657039,37.2976468451513,38.1596773353967));
#28368=CARTESIAN_POINT('Ctrl Pts',(-41.8235263633582,37.2985569656651,38.1602739131743));
#28369=CARTESIAN_POINT('Ctrl Pts',(-41.824458391616,37.2994675549367,38.1608701968413));
#28370=CARTESIAN_POINT('Ctrl Pts',(-41.8253901501336,37.3003786126306,38.161466186178));
#28371=CARTESIAN_POINT('Ctrl Pts',(-41.8263219086513,37.3012896703245,38.1620621755146));
#28372=CARTESIAN_POINT('Ctrl Pts',(-41.8272533974288,37.3022011964406,38.1626578705208));
#28373=CARTESIAN_POINT('Ctrl Pts',(-41.8281846161229,37.303113190643,38.163253270977));
#28374=CARTESIAN_POINT('Ctrl Pts',(-41.829115834817,37.3040251848454,38.1638486714333));
#28375=CARTESIAN_POINT('Ctrl Pts',(-41.8300467834275,37.304937647134,38.1644437773396));
#28376=CARTESIAN_POINT('Ctrl Pts',(-41.8309774616115,37.3058505771725,38.1650385884766));
#28377=CARTESIAN_POINT('Ctrl Pts',(-41.8319089669289,37.306764318571,38.1656339282475));
#28378=CARTESIAN_POINT('Ctrl Pts',(-41.8328402013387,37.3076785285511,38.166228972725));
#28379=CARTESIAN_POINT('Ctrl Pts',(-41.833771164497,37.3085932067754,38.1668237216893));
#28380=CARTESIAN_POINT('Ctrl Pts',(-41.7886472049959,37.2651411028535,38.1384081478369));
#28381=CARTESIAN_POINT('Ctrl Pts',(-41.7896135096978,37.266066754582,38.1390301604039));
#28382=CARTESIAN_POINT('Ctrl Pts',(-41.7905795328642,37.2669929080792,38.1396518636297));
#28383=CARTESIAN_POINT('Ctrl Pts',(-41.7915452741163,37.2679195629823,38.1402732572709));
#28384=CARTESIAN_POINT('Ctrl Pts',(-41.7925110153685,37.2688462178852,38.1408946509121));
#28385=CARTESIAN_POINT('Ctrl Pts',(-41.7934764747066,37.269773374194,38.1415157349685));
#28386=CARTESIAN_POINT('Ctrl Pts',(-41.7944416517521,37.2707010315451,38.1421365091968));
#28387=CARTESIAN_POINT('Ctrl Pts',(-41.7954068287976,37.2716286888962,38.1427572834251));
#28388=CARTESIAN_POINT('Ctrl Pts',(-41.7963717235505,37.2725568472897,38.1433777478252));
#28389=CARTESIAN_POINT('Ctrl Pts',(-41.7973363356327,37.2734855063617,38.143997902154));
#28390=CARTESIAN_POINT('Ctrl Pts',(-41.7983009477148,37.2744141654338,38.1446180564827));
#28391=CARTESIAN_POINT('Ctrl Pts',(-41.7992652771263,37.2753433251844,38.1452379007402));
#28392=CARTESIAN_POINT('Ctrl Pts',(-41.800229323489,37.2762729852495,38.1458574346833));
#28393=CARTESIAN_POINT('Ctrl Pts',(-41.8011933698517,37.2772026453146,38.1464769686264));
#28394=CARTESIAN_POINT('Ctrl Pts',(-41.8021571331657,37.278132805694,38.1470961922553));
#28395=CARTESIAN_POINT('Ctrl Pts',(-41.8031206130533,37.2790634660233,38.1477151053271));
#28396=CARTESIAN_POINT('Ctrl Pts',(-41.8040840929409,37.2799941263525,38.148334018399));
#28397=CARTESIAN_POINT('Ctrl Pts',(-41.805047289402,37.2809252866316,38.1489526209138));
#28398=CARTESIAN_POINT('Ctrl Pts',(-41.8060102020591,37.2818569464955,38.1495709126293));
#28399=CARTESIAN_POINT('Ctrl Pts',(-41.8069731147162,37.2827886063595,38.1501892043446));
#28400=CARTESIAN_POINT('Ctrl Pts',(-41.8079357435694,37.2837207658083,38.1508071852606));
#28401=CARTESIAN_POINT('Ctrl Pts',(-41.8088980882413,37.2846534244766,38.1514248551349));
#28402=CARTESIAN_POINT('Ctrl Pts',(-41.8098604329132,37.2855860831449,38.1520425250092));
#28403=CARTESIAN_POINT('Ctrl Pts',(-41.8108224934038,37.2865192410328,38.1526598838418));
#28404=CARTESIAN_POINT('Ctrl Pts',(-41.8117842693361,37.2874528977743,38.1532769313908));
#28405=CARTESIAN_POINT('Ctrl Pts',(-41.8127460452683,37.2883865545159,38.1538939789397));
#28406=CARTESIAN_POINT('Ctrl Pts',(-41.8137075366422,37.2893207101113,38.1545107152051));
#28407=CARTESIAN_POINT('Ctrl Pts',(-41.814668743081,37.2902553641942,38.1551271399451));
#28408=CARTESIAN_POINT('Ctrl Pts',(-41.8156299495197,37.2911900182772,38.155743564685));
#28409=CARTESIAN_POINT('Ctrl Pts',(-41.8165908710233,37.2921251708477,38.1563596778997));
#28410=CARTESIAN_POINT('Ctrl Pts',(-41.8175515072149,37.2930608215395,38.1569754793474));
#28411=CARTESIAN_POINT('Ctrl Pts',(-41.8185121434066,37.2939964722311,38.1575912807952));
#28412=CARTESIAN_POINT('Ctrl Pts',(-41.8194724942865,37.2949326210439,38.1582067704761));
#28413=CARTESIAN_POINT('Ctrl Pts',(-41.8204325594782,37.2958692676108,38.158821948149));
#28414=CARTESIAN_POINT('Ctrl Pts',(-41.8213926246698,37.2968059141777,38.1594371258218));
#28415=CARTESIAN_POINT('Ctrl Pts',(-41.8223524041732,37.2977430584989,38.1600519914865));
#28416=CARTESIAN_POINT('Ctrl Pts',(-41.8233118976122,37.2986807002069,38.1606665449022));
#28417=CARTESIAN_POINT('Ctrl Pts',(-41.8242713910512,37.2996183419148,38.1612810983179));
#28418=CARTESIAN_POINT('Ctrl Pts',(-41.8252305984258,37.3005564810097,38.1618953394845));
#28419=CARTESIAN_POINT('Ctrl Pts',(-41.82618951936,37.3014951171236,38.1625092681612));
#28420=CARTESIAN_POINT('Ctrl Pts',(-41.8271484402942,37.3024337532377,38.163123196838));
#28421=CARTESIAN_POINT('Ctrl Pts',(-41.828107074788,37.3033728863708,38.1637368130249));
#28422=CARTESIAN_POINT('Ctrl Pts',(-41.8290654224657,37.3043125161551,38.1643501164815));
#28423=CARTESIAN_POINT('Ctrl Pts',(-41.8300237701435,37.3052521459393,38.1649634199381));
#28424=CARTESIAN_POINT('Ctrl Pts',(-41.8309818310051,37.3061922723746,38.1655764106644));
#28425=CARTESIAN_POINT('Ctrl Pts',(-41.8319396046751,37.3071328950925,38.1661890884201));
#28426=CARTESIAN_POINT('Ctrl Pts',(-41.8328982295595,37.3080743537819,38.1668023106886));
#28427=CARTESIAN_POINT('Ctrl Pts',(-41.8338565667415,37.3090163096364,38.16741521943));
#28428=CARTESIAN_POINT('Ctrl Pts',(-41.8348146158448,37.3099587622863,38.1680278144036));
#28429=CARTESIAN_POINT('Ctrl Pts',(-41.7875737620538,37.2653631624573,38.1397452962328));
#28430=CARTESIAN_POINT('Ctrl Pts',(-41.7886504312868,37.2663961322335,38.140440940501));
#28431=CARTESIAN_POINT('Ctrl Pts',(-41.7897267538755,37.267429719819,38.1411362038889));
#28432=CARTESIAN_POINT('Ctrl Pts',(-41.7908027293106,37.2684639247247,38.1418310860678));
#28433=CARTESIAN_POINT('Ctrl Pts',(-41.7918787047456,37.2694981296305,38.1425259682467));
#28434=CARTESIAN_POINT('Ctrl Pts',(-41.7929543330269,37.2705329518566,38.1432204692165));
#28435=CARTESIAN_POINT('Ctrl Pts',(-41.7940296136454,37.2715683909132,38.1439145886488));
#28436=CARTESIAN_POINT('Ctrl Pts',(-41.795104894264,37.2726038299698,38.1446087080811));
#28437=CARTESIAN_POINT('Ctrl Pts',(-41.7961798272198,37.2736398858571,38.1453024459759));
#28438=CARTESIAN_POINT('Ctrl Pts',(-41.7972544120039,37.2746765580847,38.1459958020049));
#28439=CARTESIAN_POINT('Ctrl Pts',(-41.7983289967881,37.2757132303124,38.1466891580339));
#28440=CARTESIAN_POINT('Ctrl Pts',(-41.7994032334007,37.2767505188804,38.1473821321973));
#28441=CARTESIAN_POINT('Ctrl Pts',(-41.8004771213333,37.2777884232982,38.1480747241671));
#28442=CARTESIAN_POINT('Ctrl Pts',(-41.8015510092659,37.2788263277159,38.1487673161369));
#28443=CARTESIAN_POINT('Ctrl Pts',(-41.8026245485185,37.2798648479832,38.1494595259133));
#28444=CARTESIAN_POINT('Ctrl Pts',(-41.8036977385828,37.2809039836088,38.1501513531687));
#28445=CARTESIAN_POINT('Ctrl Pts',(-41.8047709286472,37.2819431192344,38.1508431804241));
#28446=CARTESIAN_POINT('Ctrl Pts',(-41.8058437695235,37.2829828702182,38.1515346251586));
#28447=CARTESIAN_POINT('Ctrl Pts',(-41.8069162607038,37.2840232360685,38.152225687045));
#28448=CARTESIAN_POINT('Ctrl Pts',(-41.8079887518841,37.2850636019188,38.1529167489315));
#28449=CARTESIAN_POINT('Ctrl Pts',(-41.8090608933685,37.2861045826353,38.15360742797));
#28450=CARTESIAN_POINT('Ctrl Pts',(-41.8101326846494,37.2871461777257,38.1542977238337));
#28451=CARTESIAN_POINT('Ctrl Pts',(-41.8112044759304,37.2881877728161,38.1549880196974));
#28452=CARTESIAN_POINT('Ctrl Pts',(-41.8122759170079,37.2892299822803,38.1556779323864));
#28453=CARTESIAN_POINT('Ctrl Pts',(-41.8133470073749,37.2902728056253,38.1563674615743));
#28454=CARTESIAN_POINT('Ctrl Pts',(-41.8144180977418,37.2913156289704,38.1570569907622));
#28455=CARTESIAN_POINT('Ctrl Pts',(-41.8154888373982,37.2923590661962,38.157746136449));
#28456=CARTESIAN_POINT('Ctrl Pts',(-41.8165592258371,37.2934031168091,38.1584348983086));
#28457=CARTESIAN_POINT('Ctrl Pts',(-41.8176296142761,37.294447167422,38.1591236601683));
#28458=CARTESIAN_POINT('Ctrl Pts',(-41.8186996514976,37.2954918314221,38.1598120382009));
#28459=CARTESIAN_POINT('Ctrl Pts',(-41.8197693369953,37.296537108315,38.1605000320806));
#28460=CARTESIAN_POINT('Ctrl Pts',(-41.8208390224929,37.297582385208,38.1611880259604));
#28461=CARTESIAN_POINT('Ctrl Pts',(-41.8219083562667,37.2986282749938,38.1618756356875));
#28462=CARTESIAN_POINT('Ctrl Pts',(-41.8229773378104,37.2996747771778,38.1625628609364));
#28463=CARTESIAN_POINT('Ctrl Pts',(-41.8240463193541,37.3007212793618,38.1632500861854));
#28464=CARTESIAN_POINT('Ctrl Pts',(-41.8251149486677,37.3017683939439,38.1639369269563));
#28465=CARTESIAN_POINT('Ctrl Pts',(-41.8261832252455,37.3028161204288,38.1646233829242));
#28466=CARTESIAN_POINT('Ctrl Pts',(-41.8272515018232,37.3038638469136,38.1653098388921));
#28467=CARTESIAN_POINT('Ctrl Pts',(-41.828319425665,37.3049121853013,38.165995910057));
#28468=CARTESIAN_POINT('Ctrl Pts',(-41.8293869962654,37.3059611350958,38.1666815960944));
#28469=CARTESIAN_POINT('Ctrl Pts',(-41.8304545668658,37.3070100848902,38.1673672821317));
#28470=CARTESIAN_POINT('Ctrl Pts',(-41.8315217842248,37.3080596460915,38.1680525830415));
#28471=CARTESIAN_POINT('Ctrl Pts',(-41.8325886478371,37.3091098182032,38.1687374984995));
#28472=CARTESIAN_POINT('Ctrl Pts',(-41.8336555114495,37.3101599903149,38.1694224139574));
#28473=CARTESIAN_POINT('Ctrl Pts',(-41.8347220213153,37.3112107733369,38.1701069439635));
#28474=CARTESIAN_POINT('Ctrl Pts',(-41.8357881769296,37.3122621667721,38.1707910881941));
#28475=CARTESIAN_POINT('Ctrl Pts',(-41.8368552800818,37.3133144946256,38.1714758404528));
#28476=CARTESIAN_POINT('Ctrl Pts',(-41.8379220283527,37.3143674339778,38.1721602062498));
#28477=CARTESIAN_POINT('Ctrl Pts',(-41.8389884212363,37.3154209843298,38.1728441852607));
#28478=CARTESIAN_POINT('Ctrl Pts',(-41.7864981650237,37.2655827073535,38.1410803260952));
#28479=CARTESIAN_POINT('Ctrl Pts',(-41.7876857100844,37.2667240342716,38.1418508221963));
#28480=CARTESIAN_POINT('Ctrl Pts',(-41.7888728315231,37.2678661161931,38.1426208528369));
#28481=CARTESIAN_POINT('Ctrl Pts',(-41.7900595286536,37.269008952458,38.1433904175723));
#28482=CARTESIAN_POINT('Ctrl Pts',(-41.7912462257841,37.270151788723,38.1441599823077));
#28483=CARTESIAN_POINT('Ctrl Pts',(-41.7924324986064,37.2712953793314,38.144929081138));
#28484=CARTESIAN_POINT('Ctrl Pts',(-41.7936183464348,37.2724397236224,38.1456977136189));
#28485=CARTESIAN_POINT('Ctrl Pts',(-41.794804194263,37.2735840679135,38.1464663460999));
#28486=CARTESIAN_POINT('Ctrl Pts',(-41.7959896170973,37.2747291658873,38.1472345122315));
#28487=CARTESIAN_POINT('Ctrl Pts',(-41.7971746142523,37.2758750168822,38.1480022115702));
#28488=CARTESIAN_POINT('Ctrl Pts',(-41.7983596114072,37.2770208678771,38.1487699109088));
#28489=CARTESIAN_POINT('Ctrl Pts',(-41.7995441828828,37.2781674718931,38.1495371434545));
#28490=CARTESIAN_POINT('Ctrl Pts',(-41.8007283279944,37.2793148282676,38.1503039087642));
#28491=CARTESIAN_POINT('Ctrl Pts',(-41.8019124731059,37.2804621846422,38.1510706740739));
#28492=CARTESIAN_POINT('Ctrl Pts',(-41.8030961918533,37.2816102933754,38.1518369721475));
#28493=CARTESIAN_POINT('Ctrl Pts',(-41.8042794835522,37.2827591538039,38.1526028025426));
#28494=CARTESIAN_POINT('Ctrl Pts',(-41.8054627752511,37.2839080142324,38.1533686329376));
#28495=CARTESIAN_POINT('Ctrl Pts',(-41.8066456399015,37.2850576263563,38.154133995654));
#28496=CARTESIAN_POINT('Ctrl Pts',(-41.8078280768195,37.2862079895112,38.1548988902498));
#28497=CARTESIAN_POINT('Ctrl Pts',(-41.8090105137376,37.2873583526662,38.1556637848456));
#28498=CARTESIAN_POINT('Ctrl Pts',(-41.8101925229233,37.2885094668524,38.1564282113207));
#28499=CARTESIAN_POINT('Ctrl Pts',(-41.8113741036934,37.2896613314046,38.1571921692336));
#28500=CARTESIAN_POINT('Ctrl Pts',(-41.8125556844634,37.2908131959569,38.1579561271466));
#28501=CARTESIAN_POINT('Ctrl Pts',(-41.8137368368177,37.2919658108753,38.1587196164974));
#28502=CARTESIAN_POINT('Ctrl Pts',(-41.8149175600733,37.2931191754941,38.159482636845));
#28503=CARTESIAN_POINT('Ctrl Pts',(-41.816098283329,37.2942725401128,38.1602456571926));
#28504=CARTESIAN_POINT('Ctrl Pts',(-41.8172785774861,37.2954266544319,38.161008208537));
#28505=CARTESIAN_POINT('Ctrl Pts',(-41.8184584418621,37.2965815177845,38.1617702904379));
#28506=CARTESIAN_POINT('Ctrl Pts',(-41.8196383062381,37.2977363811371,38.1625323723387));
#28507=CARTESIAN_POINT('Ctrl Pts',(-41.8208177408331,37.2988919935233,38.1632939847959));
#28508=CARTESIAN_POINT('Ctrl Pts',(-41.8219967449651,37.3000483542757,38.1640551273696));
#28509=CARTESIAN_POINT('Ctrl Pts',(-41.8231757490971,37.301204715028,38.1648162699433));
#28510=CARTESIAN_POINT('Ctrl Pts',(-41.8243543227662,37.3023618241463,38.1655769426334));
#28511=CARTESIAN_POINT('Ctrl Pts',(-41.8255324652909,37.3035196809625,38.1663371450006));
#28512=CARTESIAN_POINT('Ctrl Pts',(-41.8267106078155,37.3046775377785,38.1670973473678));
#28513=CARTESIAN_POINT('Ctrl Pts',(-41.8278883191958,37.3058361422923,38.167857079412));
#28514=CARTESIAN_POINT('Ctrl Pts',(-41.8290655987506,37.3069954938345,38.1686163406944));
#28515=CARTESIAN_POINT('Ctrl Pts',(-41.8302428783055,37.3081548453767,38.1693756019768));
#28516=CARTESIAN_POINT('Ctrl Pts',(-41.831419726035,37.3093149439473,38.1701343924974));
#28517=CARTESIAN_POINT('Ctrl Pts',(-41.8325961412587,37.3104757888764,38.1708927118178));
#28518=CARTESIAN_POINT('Ctrl Pts',(-41.8337725564824,37.3116366338054,38.1716510311383));
#28519=CARTESIAN_POINT('Ctrl Pts',(-41.8349485392002,37.3127982250929,38.1724088792586));
#28520=CARTESIAN_POINT('Ctrl Pts',(-41.8361240887322,37.3139605620678,38.1731662557409));
#28521=CARTESIAN_POINT('Ctrl Pts',(-41.8372996382642,37.3151228990428,38.1739236322232));
#28522=CARTESIAN_POINT('Ctrl Pts',(-41.8384747546104,37.3162859817051,38.1746805370675));
#28523=CARTESIAN_POINT('Ctrl Pts',(-41.8396494370912,37.3174498093833,38.1754369698366));
#28524=CARTESIAN_POINT('Ctrl Pts',(-41.8408251635625,37.3186146714048,38.1761940748797));
#28525=CARTESIAN_POINT('Ctrl Pts',(-41.8420004553969,37.3197802797668,38.1769507070081));
#28526=CARTESIAN_POINT('Ctrl Pts',(-41.8431753119136,37.320946633795,38.1777068657839));
#28527=CARTESIAN_POINT('Ctrl Pts',(-41.785420431661,37.26579975827,38.1424132548863));
#28528=CARTESIAN_POINT('Ctrl Pts',(-41.786719321559,37.2670504478503,38.1432598069792));
#28529=CARTESIAN_POINT('Ctrl Pts',(-41.7880176984179,37.2683020517983,38.1441057953634));
#28530=CARTESIAN_POINT('Ctrl Pts',(-41.7893155613103,37.2695545692201,38.1449512194344));
#28531=CARTESIAN_POINT('Ctrl Pts',(-41.7906134242027,37.270807086642,38.1457966435054));
#28532=CARTESIAN_POINT('Ctrl Pts',(-41.7919107731286,37.2720605175377,38.1466415032634));
#28533=CARTESIAN_POINT('Ctrl Pts',(-41.7932076071614,37.2733148610119,38.1474857981048));
#28534=CARTESIAN_POINT('Ctrl Pts',(-41.7945044411943,37.2745692044862,38.1483300929463));
#28535=CARTESIAN_POINT('Ctrl Pts',(-41.795800760334,37.275824460539,38.1491738228712));
#28536=CARTESIAN_POINT('Ctrl Pts',(-41.7970965636547,37.2770806282739,38.150016987277));
#28537=CARTESIAN_POINT('Ctrl Pts',(-41.7983923669755,37.2783367960088,38.1508601516828));
#28538=CARTESIAN_POINT('Ctrl Pts',(-41.7996876544773,37.2795938754256,38.1517027505694));
#28539=CARTESIAN_POINT('Ctrl Pts',(-41.8009824252349,37.2808518656268,38.1525447833351));
#28540=CARTESIAN_POINT('Ctrl Pts',(-41.8022771959926,37.2821098558278,38.1533868161008));
#28541=CARTESIAN_POINT('Ctrl Pts',(-41.8035714500061,37.283368756813,38.1542282827456));
#28542=CARTESIAN_POINT('Ctrl Pts',(-41.8048651863511,37.2846285676834,38.1550691826683));
#28543=CARTESIAN_POINT('Ctrl Pts',(-41.8061589226961,37.2858883785537,38.1559100825911));
#28544=CARTESIAN_POINT('Ctrl Pts',(-41.8074521413726,37.287149099309,38.1567504157919));
#28545=CARTESIAN_POINT('Ctrl Pts',(-41.8087448414569,37.2884107290488,38.1575901816705));
#28546=CARTESIAN_POINT('Ctrl Pts',(-41.8100375415412,37.2896723587887,38.1584299475492));
#28547=CARTESIAN_POINT('Ctrl Pts',(-41.8113297230333,37.2909348975131,38.1592691461057));
#28548=CARTESIAN_POINT('Ctrl Pts',(-41.8126213850103,37.2921983443204,38.1601077767407));
#28549=CARTESIAN_POINT('Ctrl Pts',(-41.8139130469873,37.2934617911276,38.1609464073756));
#28550=CARTESIAN_POINT('Ctrl Pts',(-41.8152041894491,37.2947261460177,38.161784470089));
#28551=CARTESIAN_POINT('Ctrl Pts',(-41.8164948114736,37.2959914080875,38.1626219642823));
#28552=CARTESIAN_POINT('Ctrl Pts',(-41.8177854334982,37.2972566701574,38.1634594584755));
#28553=CARTESIAN_POINT('Ctrl Pts',(-41.8190755350855,37.298522839407,38.1642963841487));
#28554=CARTESIAN_POINT('Ctrl Pts',(-41.820365115314,37.299789914932,38.165132740704));
#28555=CARTESIAN_POINT('Ctrl Pts',(-41.8216546955425,37.301056990457,38.1659690972592));
#28556=CARTESIAN_POINT('Ctrl Pts',(-41.8229437544123,37.3023249722574,38.1668048846966));
#28557=CARTESIAN_POINT('Ctrl Pts',(-41.8242322910026,37.3035938594276,38.1676401024191));
#28558=CARTESIAN_POINT('Ctrl Pts',(-41.8255208275929,37.3048627465979,38.1684753201416));
#28559=CARTESIAN_POINT('Ctrl Pts',(-41.8268088419038,37.3061325391379,38.1693099681493));
#28560=CARTESIAN_POINT('Ctrl Pts',(-41.8280963330153,37.3074032361407,38.1701440458461));
#28561=CARTESIAN_POINT('Ctrl Pts',(-41.8293838241269,37.3086739331435,38.1709781235428));
#28562=CARTESIAN_POINT('Ctrl Pts',(-41.830670792039,37.3099455346092,38.1718116309285));
#28563=CARTESIAN_POINT('Ctrl Pts',(-41.8319572358326,37.3112180396295,38.172644567408));
#28564=CARTESIAN_POINT('Ctrl Pts',(-41.8332436796261,37.3124905446497,38.1734775038874));
#28565=CARTESIAN_POINT('Ctrl Pts',(-41.8345295993011,37.3137639532247,38.1743098694605));
#28566=CARTESIAN_POINT('Ctrl Pts',(-41.835814993939,37.3150382644446,38.1751416635329));
#28567=CARTESIAN_POINT('Ctrl Pts',(-41.8371003885769,37.3163125756647,38.1759734576052));
#28568=CARTESIAN_POINT('Ctrl Pts',(-41.8383852581778,37.3175877895298,38.1768046801767));
#28569=CARTESIAN_POINT('Ctrl Pts',(-41.8396696018239,37.3188639051292,38.1776353306538));
#28570=CARTESIAN_POINT('Ctrl Pts',(-41.8409539454701,37.3201400207286,38.1784659811308));
#28571=CARTESIAN_POINT('Ctrl Pts',(-41.8422377631615,37.3214170380623,38.1792960595133));
#28572=CARTESIAN_POINT('Ctrl Pts',(-41.8435210539812,37.3226949562182,38.1801255652085));
#28573=CARTESIAN_POINT('Ctrl Pts',(-41.8448054853162,37.3239740101144,38.1809558081207));
#28574=CARTESIAN_POINT('Ctrl Pts',(-41.8460893888426,37.3252539664348,38.1817854773272));
#28575=CARTESIAN_POINT('Ctrl Pts',(-41.8473727636417,37.3265348242634,38.1826145722343));
#28576=CARTESIAN_POINT('Ctrl Pts',(-41.7811094982102,37.2666679619361,38.1477449700507));
#28577=CARTESIAN_POINT('Ctrl Pts',(-41.7828537674574,37.2683561021649,38.1488957461111));
#28578=CARTESIAN_POINT('Ctrl Pts',(-41.7845971659969,37.2700457942191,38.1500455654693));
#28579=CARTESIAN_POINT('Ctrl Pts',(-41.7863396919368,37.2717370362685,38.1511944268828));
#28580=CARTESIAN_POINT('Ctrl Pts',(-41.7880822178768,37.273428278318,38.1523432882963));
#28581=CARTESIAN_POINT('Ctrl Pts',(-41.7898238712172,37.2751210703628,38.153491191765));
#28582=CARTESIAN_POINT('Ctrl Pts',(-41.7915646500682,37.2768154105697,38.1546381360485));
#28583=CARTESIAN_POINT('Ctrl Pts',(-41.7933054289192,37.2785097507767,38.1557850803319));
#28584=CARTESIAN_POINT('Ctrl Pts',(-41.7950453332808,37.2802056391457,38.1569310654301));
#28585=CARTESIAN_POINT('Ctrl Pts',(-41.7967843612647,37.2819030738406,38.1580760901044));
#28586=CARTESIAN_POINT('Ctrl Pts',(-41.7985233892487,37.2836005085354,38.1592211147786));
#28587=CARTESIAN_POINT('Ctrl Pts',(-41.8002615408549,37.2852994895561,38.160365179029));
#28588=CARTESIAN_POINT('Ctrl Pts',(-41.8019988141972,37.2870000150632,38.1615082816187));
#28589=CARTESIAN_POINT('Ctrl Pts',(-41.8037360875394,37.2887005405702,38.1626513842085));
#28590=CARTESIAN_POINT('Ctrl Pts',(-41.8054724826176,37.2904026105638,38.1637935251375));
#28591=CARTESIAN_POINT('Ctrl Pts',(-41.807207997547,37.2921062232011,38.1649347031713));
#28592=CARTESIAN_POINT('Ctrl Pts',(-41.8089435124765,37.2938098358385,38.1660758812051));
#28593=CARTESIAN_POINT('Ctrl Pts',(-41.8106781472572,37.2955149911197,38.1672160963434));
#28594=CARTESIAN_POINT('Ctrl Pts',(-41.8124119000063,37.2972216871992,38.1683553473536));
#28595=CARTESIAN_POINT('Ctrl Pts',(-41.8141456527554,37.2989283832786,38.1694945983638));
#28596=CARTESIAN_POINT('Ctrl Pts',(-41.8158785234729,37.3006366201563,38.1706328852458));
#28597=CARTESIAN_POINT('Ctrl Pts',(-41.8176105102778,37.3023463959835,38.1717702067688));
#28598=CARTESIAN_POINT('Ctrl Pts',(-41.8193424970826,37.3040561718106,38.1729075282917));
#28599=CARTESIAN_POINT('Ctrl Pts',(-41.8210735999748,37.3057674865872,38.1740438844557));
#28600=CARTESIAN_POINT('Ctrl Pts',(-41.8228038170748,37.3074803384615,38.1751792740315));
#28601=CARTESIAN_POINT('Ctrl Pts',(-41.824534034175,37.3091931903357,38.1763146636074));
#28602=CARTESIAN_POINT('Ctrl Pts',(-41.826263365483,37.3109075793076,38.1774490865953));
#28603=CARTESIAN_POINT('Ctrl Pts',(-41.8279918091215,37.3126235035221,38.1785825417683));
#28604=CARTESIAN_POINT('Ctrl Pts',(-41.82972025276,37.3143394277366,38.1797159969412));
#28605=CARTESIAN_POINT('Ctrl Pts',(-41.8314478087289,37.3160568871938,38.1808484842992));
#28606=CARTESIAN_POINT('Ctrl Pts',(-41.8331744751525,37.3177758800355,38.1819800026171));
#28607=CARTESIAN_POINT('Ctrl Pts',(-41.8349011415761,37.3194948728773,38.1831115209351));
#28608=CARTESIAN_POINT('Ctrl Pts',(-41.8366269184544,37.3212153991037,38.1842420702131));
#28609=CARTESIAN_POINT('Ctrl Pts',(-41.8383518039133,37.3229374568536,38.1853716492279));
#28610=CARTESIAN_POINT('Ctrl Pts',(-41.8400766893723,37.3246595146035,38.1865012282427));
#28611=CARTESIAN_POINT('Ctrl Pts',(-41.841800683412,37.326383103877,38.1876298369945));
#28612=CARTESIAN_POINT('Ctrl Pts',(-41.8435237841602,37.3281082228095,38.1887574742621));
#28613=CARTESIAN_POINT('Ctrl Pts',(-41.8452468849085,37.3298333417421,38.1898851115296));
#28614=CARTESIAN_POINT('Ctrl Pts',(-41.8469690923652,37.331559990334,38.1910117773129));
#28615=CARTESIAN_POINT('Ctrl Pts',(-41.8486904046602,37.3332881667178,38.1921374703929));
#28616=CARTESIAN_POINT('Ctrl Pts',(-41.8504117169551,37.3350163431016,38.1932631634728));
#28617=CARTESIAN_POINT('Ctrl Pts',(-41.8521321340882,37.3367460472773,38.1943878838494));
#28618=CARTESIAN_POINT('Ctrl Pts',(-41.8538516541909,37.3384772773746,38.1955116303053));
#28619=CARTESIAN_POINT('Ctrl Pts',(-41.8555711742936,37.3402085074719,38.1966353767613));
#28620=CARTESIAN_POINT('Ctrl Pts',(-41.8572897973659,37.3419412634907,38.1977581492966));
#28621=CARTESIAN_POINT('Ctrl Pts',(-41.859007521541,37.3436755435576,38.1988799466961));
#28622=CARTESIAN_POINT('Ctrl Pts',(-41.8607267723309,37.3454113649531,38.2000027410847));
#28623=CARTESIAN_POINT('Ctrl Pts',(-41.8624451226252,37.3471487131068,38.2011245586035));
#28624=CARTESIAN_POINT('Ctrl Pts',(-41.8641625705538,37.3488875861373,38.2022453980358));
#28625=CARTESIAN_POINT('Ctrl Pts',(-41.7767643079322,37.2674961737807,38.1530429938155));
#28626=CARTESIAN_POINT('Ctrl Pts',(-41.7789615970312,37.2696380573266,38.1545174677516));
#28627=CARTESIAN_POINT('Ctrl Pts',(-41.7811574577173,37.2717824866718,38.1559903721994));
#28628=CARTESIAN_POINT('Ctrl Pts',(-41.7833518861241,37.2739294580647,38.1574617046023));
#28629=CARTESIAN_POINT('Ctrl Pts',(-41.7855463145309,37.2760764294577,38.1589330370052));
#28630=CARTESIAN_POINT('Ctrl Pts',(-41.7877393106584,37.2782259428985,38.1604027973634));
#28631=CARTESIAN_POINT('Ctrl Pts',(-41.789930870644,37.2803779946286,38.1618709831246));
#28632=CARTESIAN_POINT('Ctrl Pts',(-41.7921224306297,37.2825300463587,38.1633391688858));
#28633=CARTESIAN_POINT('Ctrl Pts',(-41.7943125544735,37.2846846363782,38.1648057800501));
#28634=CARTESIAN_POINT('Ctrl Pts',(-41.796501238317,37.2868417609214,38.1662708140698));
#28635=CARTESIAN_POINT('Ctrl Pts',(-41.7986899221604,37.2889988854646,38.1677358480895));
#28636=CARTESIAN_POINT('Ctrl Pts',(-41.8008771660035,37.2911585445316,38.1691993049645));
#28637=CARTESIAN_POINT('Ctrl Pts',(-41.8030629659915,37.2933207343499,38.1706611821514));
#28638=CARTESIAN_POINT('Ctrl Pts',(-41.8052487659796,37.2954829241681,38.1721230593384));
#28639=CARTESIAN_POINT('Ctrl Pts',(-41.8074331221127,37.2976476447376,38.1735833568372));
#28640=CARTESIAN_POINT('Ctrl Pts',(-41.8096160305401,37.2998148922788,38.175042072109));
#28641=CARTESIAN_POINT('Ctrl Pts',(-41.8117989389676,37.3019821398199,38.1765007873808));
#28642=CARTESIAN_POINT('Ctrl Pts',(-41.8139803996895,37.3041519143327,38.1779579204255));
#28643=CARTESIAN_POINT('Ctrl Pts',(-41.8161604088591,37.3063242120306,38.1794134687084));
#28644=CARTESIAN_POINT('Ctrl Pts',(-41.8183404180287,37.3084965097284,38.1808690169913));
#28645=CARTESIAN_POINT('Ctrl Pts',(-41.820518975646,37.3106713306114,38.1823229805124));
#28646=CARTESIAN_POINT('Ctrl Pts',(-41.8226960778685,37.3128486708858,38.1837753567414));
#28647=CARTESIAN_POINT('Ctrl Pts',(-41.824873180091,37.3150260111601,38.1852277329705));
#28648=CARTESIAN_POINT('Ctrl Pts',(-41.8270488269186,37.3172058708259,38.1866785219074));
#28649=CARTESIAN_POINT('Ctrl Pts',(-41.8292230145128,37.3193882460825,38.1881277210263));
#28650=CARTESIAN_POINT('Ctrl Pts',(-41.8313972021068,37.3215706213391,38.1895769201452));
#28651=CARTESIAN_POINT('Ctrl Pts',(-41.8335699304674,37.3237555121865,38.191024529446));
#28652=CARTESIAN_POINT('Ctrl Pts',(-41.8357411957597,37.3259429148172,38.1924705464073));
#28653=CARTESIAN_POINT('Ctrl Pts',(-41.8379124610521,37.3281303174478,38.1939165633685));
#28654=CARTESIAN_POINT('Ctrl Pts',(-41.8400822632763,37.3303202318617,38.19536098799));
#28655=CARTESIAN_POINT('Ctrl Pts',(-41.8422505986016,37.3325126542441,38.1968038177549));
#28656=CARTESIAN_POINT('Ctrl Pts',(-41.844418933927,37.3347050766265,38.1982466475196));
#28657=CARTESIAN_POINT('Ctrl Pts',(-41.8465858023535,37.3369000069775,38.1996878824276));
#28658=CARTESIAN_POINT('Ctrl Pts',(-41.8487512000545,37.3390974414755,38.2011275199659));
#28659=CARTESIAN_POINT('Ctrl Pts',(-41.8509165977556,37.3412948759734,38.2025671575042));
#28660=CARTESIAN_POINT('Ctrl Pts',(-41.8530805247312,37.3434948146184,38.2040051976728));
#28661=CARTESIAN_POINT('Ctrl Pts',(-41.8552429771587,37.3456972535817,38.2054416379634));
#28662=CARTESIAN_POINT('Ctrl Pts',(-41.8574054295863,37.3478996925451,38.206878078254));
#28663=CARTESIAN_POINT('Ctrl Pts',(-41.8595664074657,37.3501046318268,38.2083129186665));
#28664=CARTESIAN_POINT('Ctrl Pts',(-41.8617259069785,37.3523120675913,38.2097461566969));
#28665=CARTESIAN_POINT('Ctrl Pts',(-41.8638854064913,37.3545195033558,38.2111793947272));
#28666=CARTESIAN_POINT('Ctrl Pts',(-41.8660434276374,37.3567294356032,38.2126110303754));
#28667=CARTESIAN_POINT('Ctrl Pts',(-41.8681999666023,37.3589418604908,38.2140410611418));
#28668=CARTESIAN_POINT('Ctrl Pts',(-41.8703565055672,37.3611542853783,38.2154710919082));
#28669=CARTESIAN_POINT('Ctrl Pts',(-41.8725115623508,37.3633692029062,38.2168995177928));
#28670=CARTESIAN_POINT('Ctrl Pts',(-41.8746651331427,37.3655866092248,38.2183263363003));
#28671=CARTESIAN_POINT('Ctrl Pts',(-41.8768206179049,37.367805986247,38.2197544228823));
#28672=CARTESIAN_POINT('Ctrl Pts',(-41.8789746140328,37.3700278564857,38.2211808992288));
#28673=CARTESIAN_POINT('Ctrl Pts',(-41.8811271177098,37.372252216074,38.2226057628425));
#28674=CARTESIAN_POINT('Ctrl Pts',(-41.7723865878497,37.2682864099502,38.1583090246979));
#28675=CARTESIAN_POINT('Ctrl Pts',(-41.77504070807,37.2708945608831,38.160124042574));
#28676=CARTESIAN_POINT('Ctrl Pts',(-41.7776926120407,37.2735066617433,38.1619366253151));
#28677=CARTESIAN_POINT('Ctrl Pts',(-41.7803422915794,37.2761227044715,38.1637467673286));
#28678=CARTESIAN_POINT('Ctrl Pts',(-41.7829919711183,37.2787387471996,38.1655569093422));
#28679=CARTESIAN_POINT('Ctrl Pts',(-41.7856394262253,37.2813587317957,38.1673646106282));
#28680=CARTESIAN_POINT('Ctrl Pts',(-41.788284648732,37.283982650176,38.1691698656093));
#28681=CARTESIAN_POINT('Ctrl Pts',(-41.7909298712387,37.2866065685563,38.1709751205904));
#28682=CARTESIAN_POINT('Ctrl Pts',(-41.7935728611452,37.2892344207208,38.1727779292665));
#28683=CARTESIAN_POINT('Ctrl Pts',(-41.7962136102967,37.2918661985616,38.1745782860751));
#28684=CARTESIAN_POINT('Ctrl Pts',(-41.7988543594482,37.2944979764025,38.1763786428838));
#28685=CARTESIAN_POINT('Ctrl Pts',(-41.8014928678447,37.2971336799196,38.1781765478251));
#28686=CARTESIAN_POINT('Ctrl Pts',(-41.8041291273455,37.2997733009808,38.1799719953518));
#28687=CARTESIAN_POINT('Ctrl Pts',(-41.8067653868463,37.302412922042,38.1817674428785));
#28688=CARTESIAN_POINT('Ctrl Pts',(-41.8093993974513,37.3050564606473,38.1835604329906));
#28689=CARTESIAN_POINT('Ctrl Pts',(-41.8120311510335,37.3077039086403,38.1853509601559));
#28690=CARTESIAN_POINT('Ctrl Pts',(-41.8146629046157,37.3103513566333,38.1871414873213));
#28691=CARTESIAN_POINT('Ctrl Pts',(-41.8172924011752,37.3130027140141,38.1889295515399));
#28692=CARTESIAN_POINT('Ctrl Pts',(-41.8199196325989,37.3156579726021,38.190715147295));
#28693=CARTESIAN_POINT('Ctrl Pts',(-41.8225468640225,37.3183132311901,38.19250074305));
#28694=CARTESIAN_POINT('Ctrl Pts',(-41.8251718303104,37.3209723909853,38.1942838703415));
#28695=CARTESIAN_POINT('Ctrl Pts',(-41.8277945233635,37.3236354437833,38.1960645236678));
#28696=CARTESIAN_POINT('Ctrl Pts',(-41.8304172164165,37.3262984965811,38.197845176994));
#28697=CARTESIAN_POINT('Ctrl Pts',(-41.8330376362347,37.3289654423818,38.199623356355));
#28698=CARTESIAN_POINT('Ctrl Pts',(-41.835655774733,37.3316362729565,38.2013990562643));
#28699=CARTESIAN_POINT('Ctrl Pts',(-41.8382739132314,37.3343071035311,38.2031747561737));
#28700=CARTESIAN_POINT('Ctrl Pts',(-41.8408897704098,37.33698181888,38.2049479766314));
#28701=CARTESIAN_POINT('Ctrl Pts',(-41.8435033381974,37.3396604107503,38.2067187121664));
#28702=CARTESIAN_POINT('Ctrl Pts',(-41.846116905985,37.3423390026207,38.2084894477014));
#28703=CARTESIAN_POINT('Ctrl Pts',(-41.8487281843818,37.3450214710125,38.2102576983137));
#28704=CARTESIAN_POINT('Ctrl Pts',(-41.8513371653309,37.3477078076495,38.2120234585475));
#28705=CARTESIAN_POINT('Ctrl Pts',(-41.85394614628,37.3503941442864,38.2137892187814));
#28706=CARTESIAN_POINT('Ctrl Pts',(-41.8565528297814,37.3530843491685,38.2155524886367));
#28707=CARTESIAN_POINT('Ctrl Pts',(-41.8591572077926,37.3557784139952,38.2173132626732));
#28708=CARTESIAN_POINT('Ctrl Pts',(-41.8617615858037,37.358472478822,38.2190740367097));
#28709=CARTESIAN_POINT('Ctrl Pts',(-41.8643636583245,37.3611704035935,38.2208323149273));
#28710=CARTESIAN_POINT('Ctrl Pts',(-41.8669634173266,37.3638721799855,38.2225880919011));
#28711=CARTESIAN_POINT('Ctrl Pts',(-41.8695631763287,37.3665739563775,38.224343868875));
#28712=CARTESIAN_POINT('Ctrl Pts',(-41.872160621812,37.3692795843902,38.2260971446049));
#28713=CARTESIAN_POINT('Ctrl Pts',(-41.8747557457625,37.3719890556753,38.2278479136815));
#28714=CARTESIAN_POINT('Ctrl Pts',(-41.877350869713,37.3746985269606,38.229598682758));
#28715=CARTESIAN_POINT('Ctrl Pts',(-41.8799436721306,37.3774118415184,38.2313469451812));
#28716=CARTESIAN_POINT('Ctrl Pts',(-41.8825341450154,37.3801289909773,38.2330926955569));
#28717=CARTESIAN_POINT('Ctrl Pts',(-41.8851246179004,37.3828461404361,38.2348384459327));
#28718=CARTESIAN_POINT('Ctrl Pts',(-41.8877127612526,37.3855671247958,38.2365816842609));
#28719=CARTESIAN_POINT('Ctrl Pts',(-41.8902985670866,37.3882919356613,38.2383224051631));
#28720=CARTESIAN_POINT('Ctrl Pts',(-41.8928866710366,37.3910191681824,38.2400646731182));
#28721=CARTESIAN_POINT('Ctrl Pts',(-41.8954724333117,37.3937502340137,38.2418044191706));
#28722=CARTESIAN_POINT('Ctrl Pts',(-41.8980558459195,37.3964851247139,38.2435416379429));
#28723=CARTESIAN_POINT('Ctrl Pts',(-41.7680088677671,37.2690766461197,38.1635750555802));
#28724=CARTESIAN_POINT('Ctrl Pts',(-41.7711198191088,37.2721510644396,38.1657306173963));
#28725=CARTESIAN_POINT('Ctrl Pts',(-41.774227766364,37.2752308368149,38.1678828784307));
#28726=CARTESIAN_POINT('Ctrl Pts',(-41.7773326970348,37.2783159508782,38.170031830055));
#28727=CARTESIAN_POINT('Ctrl Pts',(-41.7804376277057,37.2814010649415,38.1721807816792));
#28728=CARTESIAN_POINT('Ctrl Pts',(-41.7835395417922,37.2844915206928,38.1743264238931));
#28729=CARTESIAN_POINT('Ctrl Pts',(-41.7866384268199,37.2875873057234,38.176468748094));
#28730=CARTESIAN_POINT('Ctrl Pts',(-41.7897373118478,37.2906830907538,38.1786110722949));
#28731=CARTESIAN_POINT('Ctrl Pts',(-41.7928331678168,37.2937842050635,38.1807500784827));
#28732=CARTESIAN_POINT('Ctrl Pts',(-41.7959259822763,37.296890636202,38.1828857580804));
#28733=CARTESIAN_POINT('Ctrl Pts',(-41.7990187967359,37.2999970673404,38.1850214376781));
#28734=CARTESIAN_POINT('Ctrl Pts',(-41.802108569686,37.3031088153076,38.1871537906857));
#28735=CARTESIAN_POINT('Ctrl Pts',(-41.8051952886994,37.3062258676117,38.1892828085522));
#28736=CARTESIAN_POINT('Ctrl Pts',(-41.8082820077129,37.3093429199158,38.1914118264186));
#28737=CARTESIAN_POINT('Ctrl Pts',(-41.8113656727898,37.3124652765569,38.1935375091439));
#28738=CARTESIAN_POINT('Ctrl Pts',(-41.8144462715268,37.3155929250019,38.1956598482028));
#28739=CARTESIAN_POINT('Ctrl Pts',(-41.8175268702638,37.3187205734467,38.1977821872618));
#28740=CARTESIAN_POINT('Ctrl Pts',(-41.8206044026609,37.3218535136954,38.1999011826544));
#28741=CARTESIAN_POINT('Ctrl Pts',(-41.8236788563386,37.3249917331736,38.2020168258816));
#28742=CARTESIAN_POINT('Ctrl Pts',(-41.8267533100164,37.3281299526517,38.2041324691088));
#28743=CARTESIAN_POINT('Ctrl Pts',(-41.8298246849748,37.3312734513592,38.2062447601707));
#28744=CARTESIAN_POINT('Ctrl Pts',(-41.8328929688584,37.3344222166808,38.2083536905941));
#28745=CARTESIAN_POINT('Ctrl Pts',(-41.835961252742,37.3375709820023,38.2104626210175));
#28746=CARTESIAN_POINT('Ctrl Pts',(-41.8390264455507,37.3407250139377,38.2125681908025));
#28747=CARTESIAN_POINT('Ctrl Pts',(-41.8420885349533,37.3438842998304,38.2146703915024));
#28748=CARTESIAN_POINT('Ctrl Pts',(-41.8451506243559,37.3470435857233,38.2167725922022));
#28749=CARTESIAN_POINT('Ctrl Pts',(-41.8482096103522,37.3502081255734,38.2188714238168));
#28750=CARTESIAN_POINT('Ctrl Pts',(-41.851265480635,37.3533779066835,38.2209668779256));
#28751=CARTESIAN_POINT('Ctrl Pts',(-41.8543213509179,37.3565476877935,38.2230623320344));
#28752=CARTESIAN_POINT('Ctrl Pts',(-41.8573741054873,37.3597227101635,38.2251544086374));
#28753=CARTESIAN_POINT('Ctrl Pts',(-41.8604237320601,37.362902961055,38.2272430993402));
#28754=CARTESIAN_POINT('Ctrl Pts',(-41.863473358633,37.3660832119465,38.2293317900431));
#28755=CARTESIAN_POINT('Ctrl Pts',(-41.8665198572093,37.3692686913596,38.2314170948458));
#28756=CARTESIAN_POINT('Ctrl Pts',(-41.8695632155305,37.3724593865151,38.2334990053805));
#28757=CARTESIAN_POINT('Ctrl Pts',(-41.8726065738518,37.3756500816706,38.2355809159152));
#28758=CARTESIAN_POINT('Ctrl Pts',(-41.8756467919178,37.3788459925686,38.2376594321818));
#28759=CARTESIAN_POINT('Ctrl Pts',(-41.8786838574945,37.3820471063893,38.2397345458388));
#28760=CARTESIAN_POINT('Ctrl Pts',(-41.8817209230711,37.3852482202101,38.2418096594958));
#28761=CARTESIAN_POINT('Ctrl Pts',(-41.8847548361584,37.3884545369535,38.2438813705433));
#28762=CARTESIAN_POINT('Ctrl Pts',(-41.8877855845465,37.3916660437595,38.2459496706661));
#28763=CARTESIAN_POINT('Ctrl Pts',(-41.8908163329347,37.3948775505653,38.2480179707889));
#28764=CARTESIAN_POINT('Ctrl Pts',(-41.8938439166238,37.3980942474337,38.250082859987));
#28765=CARTESIAN_POINT('Ctrl Pts',(-41.8968683234287,37.4013161214637,38.2521443299721));
#28766=CARTESIAN_POINT('Ctrl Pts',(-41.8998927302336,37.4045379954937,38.2542057999571));
#28767=CARTESIAN_POINT('Ctrl Pts',(-41.9029139601543,37.4077650466855,38.256263850729));
#28768=CARTESIAN_POINT('Ctrl Pts',(-41.9059320010304,37.4109972620978,38.2583184740259));
#28769=CARTESIAN_POINT('Ctrl Pts',(-41.9089527241683,37.4142323501178,38.2603749233541));
#28770=CARTESIAN_POINT('Ctrl Pts',(-41.9119702525905,37.4174726115418,38.2624279391123));
#28771=CARTESIAN_POINT('Ctrl Pts',(-41.9149845741293,37.4207180333538,38.2644775130434));
#28772=CARTESIAN_POINT('Ctrl Pts',(-41.7635986248403,37.2698289147397,38.1688091004257));
#28773=CARTESIAN_POINT('Ctrl Pts',(-41.767170149167,37.2733820604892,38.1713220115573));
#28774=CARTESIAN_POINT('Ctrl Pts',(-41.7707376507708,37.2769423757664,38.1738305026664));
#28775=CARTESIAN_POINT('Ctrl Pts',(-41.774301110476,37.2805098414877,38.1763345603498));
#28776=CARTESIAN_POINT('Ctrl Pts',(-41.7778645701812,37.284077307209,38.1788386180331));
#28777=CARTESIAN_POINT('Ctrl Pts',(-41.7814239879878,37.2876519233744,38.1813382422907));
#28778=CARTESIAN_POINT('Ctrl Pts',(-41.7849793447612,37.2912336708281,38.1838334197642));
#28779=CARTESIAN_POINT('Ctrl Pts',(-41.7885347015346,37.2948154182817,38.1863285972376));
#28780=CARTESIAN_POINT('Ctrl Pts',(-41.7920859972746,37.2984042970236,38.1888193279269));
#28781=CARTESIAN_POINT('Ctrl Pts',(-41.7956332128876,37.3020002878258,38.1913055985184));
#28782=CARTESIAN_POINT('Ctrl Pts',(-41.7991804285007,37.305596278628,38.19379186911));
#28783=CARTESIAN_POINT('Ctrl Pts',(-41.8027235639866,37.3091993814906,38.1962736796039));
#28784=CARTESIAN_POINT('Ctrl Pts',(-41.806262600293,37.3128095771137,38.1987510167316));
#28785=CARTESIAN_POINT('Ctrl Pts',(-41.8098016365993,37.3164197727369,38.2012283538592));
#28786=CARTESIAN_POINT('Ctrl Pts',(-41.813336573726,37.3200370611205,38.2037012176207));
#28787=CARTESIAN_POINT('Ctrl Pts',(-41.8168673926618,37.3236614228931,38.2061695947926));
#28788=CARTESIAN_POINT('Ctrl Pts',(-41.8203982115976,37.3272857846658,38.2086379719645));
#28789=CARTESIAN_POINT('Ctrl Pts',(-41.8239249123425,37.3309172198275,38.2111018625468));
#28790=CARTESIAN_POINT('Ctrl Pts',(-41.8274474759268,37.3345557089351,38.2135612533614));
#28791=CARTESIAN_POINT('Ctrl Pts',(-41.8309700395111,37.3381941980428,38.216020644176));
#28792=CARTESIAN_POINT('Ctrl Pts',(-41.8344884659347,37.3418397410965,38.2184755352229));
#28793=CARTESIAN_POINT('Ctrl Pts',(-41.8380027362697,37.3454923185817,38.2209259133694));
#28794=CARTESIAN_POINT('Ctrl Pts',(-41.8415170066047,37.349144896067,38.2233762915158));
#28795=CARTESIAN_POINT('Ctrl Pts',(-41.8450271208511,37.3528045079838,38.2258221567618));
#28796=CARTESIAN_POINT('Ctrl Pts',(-41.8485330601227,37.3564711347466,38.2282634960202));
#28797=CARTESIAN_POINT('Ctrl Pts',(-41.8520389993942,37.3601377615094,38.2307048352785));
#28798=CARTESIAN_POINT('Ctrl Pts',(-41.855540763691,37.3638114031182,38.2331416485492));
#28799=CARTESIAN_POINT('Ctrl Pts',(-41.8590383341689,37.3674920399165,38.2355739227905));
#28800=CARTESIAN_POINT('Ctrl Pts',(-41.8625359046468,37.3711726767147,38.2380061970319));
#28801=CARTESIAN_POINT('Ctrl Pts',(-41.8660292813057,37.3748603087024,38.240433932244));
#28802=CARTESIAN_POINT('Ctrl Pts',(-41.8695184453439,37.3785549161521,38.2428571154308));
#28803=CARTESIAN_POINT('Ctrl Pts',(-41.873007609382,37.3822495236018,38.2452802986178));
#28804=CARTESIAN_POINT('Ctrl Pts',(-41.8764925607994,37.3859511065137,38.2476989297795));
#28805=CARTESIAN_POINT('Ctrl Pts',(-41.8799732808366,37.3896596450895,38.250112995966));
#28806=CARTESIAN_POINT('Ctrl Pts',(-41.8834540008737,37.3933681836653,38.2525270621525));
#28807=CARTESIAN_POINT('Ctrl Pts',(-41.8869304895305,37.3970836779052,38.2549365633638));
#28808=CARTESIAN_POINT('Ctrl Pts',(-41.8904027280903,37.4008061079406,38.257341486696));
#28809=CARTESIAN_POINT('Ctrl Pts',(-41.89387496665,37.404528537976,38.2597464100281));
#28810=CARTESIAN_POINT('Ctrl Pts',(-41.8973429551125,37.4082579038071,38.2621467554809));
#28811=CARTESIAN_POINT('Ctrl Pts',(-41.9008066748037,37.4119941854949,38.2645425101966));
#28812=CARTESIAN_POINT('Ctrl Pts',(-41.904270394495,37.4157304671828,38.2669382649123));
#28813=CARTESIAN_POINT('Ctrl Pts',(-41.9077298454149,37.4194736647275,38.2693294288908));
#28814=CARTESIAN_POINT('Ctrl Pts',(-41.9111850089323,37.4232237581202,38.2717159893205));
#28815=CARTESIAN_POINT('Ctrl Pts',(-41.9146401724497,37.4269738515128,38.2741025497502));
#28816=CARTESIAN_POINT('Ctrl Pts',(-41.9180910485645,37.4307308407536,38.2764845066309));
#28817=CARTESIAN_POINT('Ctrl Pts',(-41.9215376186886,37.4344947057637,38.2788618471974));
#28818=CARTESIAN_POINT('Ctrl Pts',(-41.9249872519267,37.438261915881,38.2812413006078));
#28819=CARTESIAN_POINT('Ctrl Pts',(-41.9284325715169,37.4420360139948,38.2836161294949));
#28820=CARTESIAN_POINT('Ctrl Pts',(-41.9318735588647,37.4458169799027,38.2859863211058));
#28821=CARTESIAN_POINT('Ctrl Pts',(-41.7591585257862,37.2705463289668,38.1740137819355));
#28822=CARTESIAN_POINT('Ctrl Pts',(-41.7631892704991,37.2745846634979,38.1768957540815));
#28823=CARTESIAN_POINT('Ctrl Pts',(-41.7672147321291,37.2786324138423,38.1797719213672));
#28824=CARTESIAN_POINT('Ctrl Pts',(-41.7712348810694,37.2826895502289,38.1826422626386));
#28825=CARTESIAN_POINT('Ctrl Pts',(-41.7752550300097,37.2867466866155,38.1855126039099));
#28826=CARTESIAN_POINT('Ctrl Pts',(-41.7792698662602,37.2908132090444,38.1883771191669));
#28827=CARTESIAN_POINT('Ctrl Pts',(-41.783279360292,37.2948890876066,38.1912357873412));
#28828=CARTESIAN_POINT('Ctrl Pts',(-41.7872888543238,37.2989649661687,38.1940944555156));
#28829=CARTESIAN_POINT('Ctrl Pts',(-41.791293006137,37.3030502008641,38.1969472766072));
#28830=CARTESIAN_POINT('Ctrl Pts',(-41.7952917862812,37.3071447616462,38.1997942296338));
#28831=CARTESIAN_POINT('Ctrl Pts',(-41.7992905664254,37.3112393224283,38.2026411826604));
#28832=CARTESIAN_POINT('Ctrl Pts',(-41.8032839749007,37.315343209297,38.2054822676221));
#28833=CARTESIAN_POINT('Ctrl Pts',(-41.8072719823357,37.3194563920684,38.2083174636227));
#28834=CARTESIAN_POINT('Ctrl Pts',(-41.8112599897708,37.3235695748399,38.2111526596233));
#28835=CARTESIAN_POINT('Ctrl Pts',(-41.8152425961656,37.3276920535142,38.2139819666629));
#28836=CARTESIAN_POINT('Ctrl Pts',(-41.8192197722285,37.3318237977707,38.2168053639321));
#28837=CARTESIAN_POINT('Ctrl Pts',(-41.8231969482913,37.3359555420272,38.2196287612014));
#28838=CARTESIAN_POINT('Ctrl Pts',(-41.8271686940221,37.3400965518658,38.2224462487002));
#28839=CARTESIAN_POINT('Ctrl Pts',(-41.8311349802089,37.34424679683,38.2252578057062));
#28840=CARTESIAN_POINT('Ctrl Pts',(-41.8351012663957,37.348397041794,38.2280693627123));
#28841=CARTESIAN_POINT('Ctrl Pts',(-41.8390620930385,37.3525565218834,38.2308749892255));
#28842=CARTESIAN_POINT('Ctrl Pts',(-41.8430174310058,37.3567252065055,38.2336746646106));
#28843=CARTESIAN_POINT('Ctrl Pts',(-41.846972768973,37.3608938911276,38.2364743399958));
#28844=CARTESIAN_POINT('Ctrl Pts',(-41.8509226182647,37.3650717802822,38.2392680642529));
#28845=CARTESIAN_POINT('Ctrl Pts',(-41.8548669498298,37.3692588432415,38.2420558168344));
#28846=CARTESIAN_POINT('Ctrl Pts',(-41.8588112813949,37.3734459062008,38.2448435694158));
#28847=CARTESIAN_POINT('Ctrl Pts',(-41.8627500952336,37.3776421429644,38.2476253503216));
#28848=CARTESIAN_POINT('Ctrl Pts',(-41.866683362376,37.3818475226697,38.2504011390917));
#28849=CARTESIAN_POINT('Ctrl Pts',(-41.8706166295184,37.3860529023749,38.253176927862));
#28850=CARTESIAN_POINT('Ctrl Pts',(-41.8745443499646,37.3902674250216,38.2559467244967));
#28851=CARTESIAN_POINT('Ctrl Pts',(-41.8784664948264,37.3944910596122,38.2587105086242));
#28852=CARTESIAN_POINT('Ctrl Pts',(-41.8823886396882,37.3987146942029,38.2614742927517));
#28853=CARTESIAN_POINT('Ctrl Pts',(-41.8863052089657,37.4029474407374,38.264232064372));
#28854=CARTESIAN_POINT('Ctrl Pts',(-41.8902161738527,37.4071892680843,38.2669838032018));
#28855=CARTESIAN_POINT('Ctrl Pts',(-41.8941271387397,37.4114310954311,38.2697355420317));
#28856=CARTESIAN_POINT('Ctrl Pts',(-41.8980324992362,37.4156820035903,38.2724812480711));
#28857=CARTESIAN_POINT('Ctrl Pts',(-41.9019322266185,37.4199419612967,38.2752209011256));
#28858=CARTESIAN_POINT('Ctrl Pts',(-41.9058319540008,37.4242019190032,38.27796055418));
#28859=CARTESIAN_POINT('Ctrl Pts',(-41.909726048269,37.4284709262567,38.2806941542496));
#28860=CARTESIAN_POINT('Ctrl Pts',(-41.9136144807821,37.4327489516591,38.2834216812288));
#28861=CARTESIAN_POINT('Ctrl Pts',(-41.9175029132953,37.4370269770616,38.2861492082079));
#28862=CARTESIAN_POINT('Ctrl Pts',(-41.9213856840535,37.4413140206129,38.2888706620967));
#28863=CARTESIAN_POINT('Ctrl Pts',(-41.9252627644992,37.4456100507822,38.2915860228789));
#28864=CARTESIAN_POINT('Ctrl Pts',(-41.9291398449449,37.4499060809515,38.2943013836612));
#28865=CARTESIAN_POINT('Ctrl Pts',(-41.933011235078,37.4542110977388,38.2970106513369));
#28866=CARTESIAN_POINT('Ctrl Pts',(-41.9368769064249,37.4585250694809,38.2997138059797));
#28867=CARTESIAN_POINT('Ctrl Pts',(-41.9407460133587,37.4628428752336,38.3024193630313));
#28868=CARTESIAN_POINT('Ctrl Pts',(-41.9446093913366,37.4671696518656,38.3051187961791));
#28869=CARTESIAN_POINT('Ctrl Pts',(-41.9484670118931,37.4715053674971,38.3078120855339));
#28870=CARTESIAN_POINT('Ctrl Pts',(-41.7547184267321,37.271263743194,38.1792184634453));
#28871=CARTESIAN_POINT('Ctrl Pts',(-41.7592083918311,37.2757872665067,38.1824694966057));
#28872=CARTESIAN_POINT('Ctrl Pts',(-41.7636918134875,37.2803224519181,38.1857133400681));
#28873=CARTESIAN_POINT('Ctrl Pts',(-41.7681686516628,37.28486925897,38.1889499649274));
#28874=CARTESIAN_POINT('Ctrl Pts',(-41.7726454898382,37.2894160660219,38.1921865897868));
#28875=CARTESIAN_POINT('Ctrl Pts',(-41.7771157445325,37.2939744947144,38.1954159960432));
#28876=CARTESIAN_POINT('Ctrl Pts',(-41.7815793758228,37.2985445043851,38.1986381549183));
#28877=CARTESIAN_POINT('Ctrl Pts',(-41.7860430071131,37.3031145140558,38.2018603137936));
#28878=CARTESIAN_POINT('Ctrl Pts',(-41.7905000149993,37.3076961047048,38.2050752252875));
#28879=CARTESIAN_POINT('Ctrl Pts',(-41.7949503596747,37.3122892354667,38.2082828607492));
#28880=CARTESIAN_POINT('Ctrl Pts',(-41.7994007043501,37.3168823662286,38.2114904962109));
#28881=CARTESIAN_POINT('Ctrl Pts',(-41.8038443858147,37.3214870371033,38.2146908556402));
#28882=CARTESIAN_POINT('Ctrl Pts',(-41.8082813643785,37.3261032070232,38.2178839105138));
#28883=CARTESIAN_POINT('Ctrl Pts',(-41.8127183429423,37.330719376943,38.2210769653874));
#28884=CARTESIAN_POINT('Ctrl Pts',(-41.8171486186053,37.3353470459079,38.2242627157051));
#28885=CARTESIAN_POINT('Ctrl Pts',(-41.8215721517952,37.3399861726482,38.2274411330717));
#28886=CARTESIAN_POINT('Ctrl Pts',(-41.825995684985,37.3446252993886,38.2306195504382));
#28887=CARTESIAN_POINT('Ctrl Pts',(-41.8304124757016,37.3492758839043,38.2337906348536));
#28888=CARTESIAN_POINT('Ctrl Pts',(-41.834822484491,37.3539378847247,38.2369543580511));
#28889=CARTESIAN_POINT('Ctrl Pts',(-41.8392324932803,37.3585998855452,38.2401180812485));
#28890=CARTESIAN_POINT('Ctrl Pts',(-41.8436357201424,37.3632733026704,38.243274443228));
#28891=CARTESIAN_POINT('Ctrl Pts',(-41.8480321257418,37.3679580944293,38.2464234158519));
#28892=CARTESIAN_POINT('Ctrl Pts',(-41.8524285313413,37.3726428861882,38.2495723884758));
#28893=CARTESIAN_POINT('Ctrl Pts',(-41.8568181156782,37.3773390525808,38.252713971744));
#28894=CARTESIAN_POINT('Ctrl Pts',(-41.8612008395369,37.3820465517364,38.2558481376486));
#28895=CARTESIAN_POINT('Ctrl Pts',(-41.8655835633956,37.3867540508921,38.2589823035531));
#28896=CARTESIAN_POINT('Ctrl Pts',(-41.8699594267761,37.3914728828107,38.2621090520939));
#28897=CARTESIAN_POINT('Ctrl Pts',(-41.8743283905831,37.396203005423,38.265228355393));
#28898=CARTESIAN_POINT('Ctrl Pts',(-41.8786973543901,37.4009331280351,38.2683476586921));
#28899=CARTESIAN_POINT('Ctrl Pts',(-41.8830594186235,37.4056745413409,38.2714595167494));
#28900=CARTESIAN_POINT('Ctrl Pts',(-41.887414544309,37.4104272030723,38.2745639018175));
#28901=CARTESIAN_POINT('Ctrl Pts',(-41.8917696699944,37.4151798648039,38.2776682868856));
#28902=CARTESIAN_POINT('Ctrl Pts',(-41.8961178571319,37.4199437749612,38.2807651989644));
#28903=CARTESIAN_POINT('Ctrl Pts',(-41.9004590668688,37.4247188910791,38.2838546104377));
#28904=CARTESIAN_POINT('Ctrl Pts',(-41.9048002766057,37.429494007197,38.2869440219109));
#28905=CARTESIAN_POINT('Ctrl Pts',(-41.9091345089417,37.4342803292756,38.2900259327783));
#28906=CARTESIAN_POINT('Ctrl Pts',(-41.9134617251467,37.4390778146529,38.2931003155552));
#28907=CARTESIAN_POINT('Ctrl Pts',(-41.9177889413516,37.4438753000302,38.2961746983321));
#28908=CARTESIAN_POINT('Ctrl Pts',(-41.9221091414255,37.4486839487062,38.2992415530183));
#28909=CARTESIAN_POINT('Ctrl Pts',(-41.9264222867606,37.4535037178233,38.3023008522609));
#28910=CARTESIAN_POINT('Ctrl Pts',(-41.9307354320957,37.4583234869404,38.3053601515035));
#28911=CARTESIAN_POINT('Ctrl Pts',(-41.9350415226922,37.4631543764984,38.3084118953025));
#28912=CARTESIAN_POINT('Ctrl Pts',(-41.9393405200661,37.4679963434443,38.3114560564374));
#28913=CARTESIAN_POINT('Ctrl Pts',(-41.9436395174402,37.4728383103901,38.3145002175723));
#28914=CARTESIAN_POINT('Ctrl Pts',(-41.9479314215916,37.4776913547239,38.317536796043));
#28915=CARTESIAN_POINT('Ctrl Pts',(-41.9522161941611,37.482555433198,38.320565764762));
#28916=CARTESIAN_POINT('Ctrl Pts',(-41.9565047747907,37.4874238345862,38.3235974254546));
#28917=CARTESIAN_POINT('Ctrl Pts',(-41.9607862111563,37.4923032897364,38.3266214628634));
#28918=CARTESIAN_POINT('Ctrl Pts',(-41.9650604649214,37.4971937550915,38.329637849962));
#28919=CARTESIAN_POINT('Ctrl Pts',(-41.7502484969702,37.2719463327032,38.1843938066194));
#28920=CARTESIAN_POINT('Ctrl Pts',(-41.7551962256523,37.276961374585,38.1880254939256));
#28921=CARTESIAN_POINT('Ctrl Pts',(-41.7601359088508,37.2819907555891,38.1916483411455));
#28922=CARTESIAN_POINT('Ctrl Pts',(-41.7650674923212,37.2870344205738,38.1952623086258));
#28923=CARTESIAN_POINT('Ctrl Pts',(-41.7699990757916,37.2920780855585,38.1988762761062));
#28924=CARTESIAN_POINT('Ctrl Pts',(-41.7749225595338,37.2971360345237,38.2024813638471));
#28925=CARTESIAN_POINT('Ctrl Pts',(-41.7798378894764,37.3022082120227,38.2060775323852));
#28926=CARTESIAN_POINT('Ctrl Pts',(-41.784753219419,37.3072803895216,38.2096737009232));
#28927=CARTESIAN_POINT('Ctrl Pts',(-41.7896603955619,37.3123667955542,38.2132609502583));
#28928=CARTESIAN_POINT('Ctrl Pts',(-41.7945593640076,37.3174673743695,38.2168392411177));
#28929=CARTESIAN_POINT('Ctrl Pts',(-41.7994583324533,37.3225679531848,38.2204175319771));
#28930=CARTESIAN_POINT('Ctrl Pts',(-41.8043490932019,37.3276827047826,38.2239868643607));
#28931=CARTESIAN_POINT('Ctrl Pts',(-41.8092315925311,37.3328115731093,38.2275471991868));
#28932=CARTESIAN_POINT('Ctrl Pts',(-41.8141140918603,37.3379404414361,38.231107534013));
#28933=CARTESIAN_POINT('Ctrl Pts',(-41.8189883297701,37.3430834264914,38.2346588712817));
#28934=CARTESIAN_POINT('Ctrl Pts',(-41.8238542527147,37.3482404719199,38.2382011721036));
#28935=CARTESIAN_POINT('Ctrl Pts',(-41.8287201756593,37.3533975173484,38.2417434729254));
#28936=CARTESIAN_POINT('Ctrl Pts',(-41.8335777836387,37.3585686231499,38.2452767373004));
#28937=CARTESIAN_POINT('Ctrl Pts',(-41.8384270232845,37.3637537326682,38.2488009265318));
#28938=CARTESIAN_POINT('Ctrl Pts',(-41.8432762629303,37.3689388421866,38.2523251157632));
#28939=CARTESIAN_POINT('Ctrl Pts',(-41.8481171342425,37.3741379554216,38.2558402298512));
#28940=CARTESIAN_POINT('Ctrl Pts',(-41.8529495840314,37.3793510154178,38.2593462302928));
#28941=CARTESIAN_POINT('Ctrl Pts',(-41.8577820338202,37.3845640754139,38.2628522307343));
#28942=CARTESIAN_POINT('Ctrl Pts',(-41.8626060620857,37.389791082171,38.2663491175296));
#28943=CARTESIAN_POINT('Ctrl Pts',(-41.8674216158177,37.3950319784353,38.2698368523701));
#28944=CARTESIAN_POINT('Ctrl Pts',(-41.8722371695496,37.4002728746996,38.2733245872106));
#28945=CARTESIAN_POINT('Ctrl Pts',(-41.8770442487481,37.4055276604708,38.2768031700963));
#28946=CARTESIAN_POINT('Ctrl Pts',(-41.8818428005838,37.4107962781982,38.2802725629143));
#28947=CARTESIAN_POINT('Ctrl Pts',(-41.8866413524195,37.4160648959255,38.2837419557322));
#28948=CARTESIAN_POINT('Ctrl Pts',(-41.8914313768924,37.4213473456087,38.2872021584824));
#28949=CARTESIAN_POINT('Ctrl Pts',(-41.8962128213549,37.4266435694012,38.2906531332478));
#28950=CARTESIAN_POINT('Ctrl Pts',(-41.9009942658176,37.4319397931935,38.2941041080132));
#28951=CARTESIAN_POINT('Ctrl Pts',(-41.9057671302699,37.4372497910949,38.2975458547937));
#28952=CARTESIAN_POINT('Ctrl Pts',(-41.9105313622474,37.4425735049638,38.3009783358694));
#28953=CARTESIAN_POINT('Ctrl Pts',(-41.915295594225,37.4478972188327,38.3044108169451));
#28954=CARTESIAN_POINT('Ctrl Pts',(-41.9200511937278,37.4532346486689,38.3078340323158));
#28955=CARTESIAN_POINT('Ctrl Pts',(-41.9247981084754,37.4585857360373,38.3112479444592));
#28956=CARTESIAN_POINT('Ctrl Pts',(-41.9295450232231,37.4639368234058,38.3146618566026));
#28957=CARTESIAN_POINT('Ctrl Pts',(-41.9342832532155,37.4693015683065,38.3180664655185));
#28958=CARTESIAN_POINT('Ctrl Pts',(-41.9390127463574,37.4746799120121,38.321461733883));
#28959=CARTESIAN_POINT('Ctrl Pts',(-41.9437422394994,37.4800582557176,38.3248570022476));
#28960=CARTESIAN_POINT('Ctrl Pts',(-41.9484629957909,37.4854501982279,38.3282429300606));
#28961=CARTESIAN_POINT('Ctrl Pts',(-41.9531749633228,37.4908556805245,38.3316194801973));
#28962=CARTESIAN_POINT('Ctrl Pts',(-41.9578869308548,37.4962611628211,38.3349960303341));
#28963=CARTESIAN_POINT('Ctrl Pts',(-41.9625901096271,37.5016801849039,38.3383632027944));
#28964=CARTESIAN_POINT('Ctrl Pts',(-41.9672844479182,37.5071126874645,38.3417209606536));
#28965=CARTESIAN_POINT('Ctrl Pts',(-41.9719829582679,37.512550018122,38.3450817026954));
#28966=CARTESIAN_POINT('Ctrl Pts',(-41.9766726124154,37.5180008532292,38.3484330133941));
#28967=CARTESIAN_POINT('Ctrl Pts',(-41.98135335869,37.5234651330302,38.3517748559277));
#28968=CARTESIAN_POINT('Ctrl Pts',(-41.7457520939339,37.2725980170017,38.1895431134749));
#28969=CARTESIAN_POINT('Ctrl Pts',(-41.7511511407049,37.278104218446,38.19356073873));
#28970=CARTESIAN_POINT('Ctrl Pts',(-41.7565404115942,37.2836278430274,38.1975676225998));
#28971=CARTESIAN_POINT('Ctrl Pts',(-41.7619198332558,37.2891688155715,38.2015637105522));
#28972=CARTESIAN_POINT('Ctrl Pts',(-41.7672992549175,37.2947097881156,38.2055597985045));
#28973=CARTESIAN_POINT('Ctrl Pts',(-41.7726688273513,37.3002681086224,38.2095450905392));
#28974=CARTESIAN_POINT('Ctrl Pts',(-41.7780284774797,37.3058437014451,38.2135195324181));
#28975=CARTESIAN_POINT('Ctrl Pts',(-41.783388127608,37.3114192942678,38.2174939742969));
#28976=CARTESIAN_POINT('Ctrl Pts',(-41.7887378554306,37.3170121594064,38.2214575660198));
#28977=CARTESIAN_POINT('Ctrl Pts',(-41.7940775881398,37.3226222207441,38.2254102536438));
#28978=CARTESIAN_POINT('Ctrl Pts',(-41.799417320849,37.3282322820818,38.2293629412678));
#28979=CARTESIAN_POINT('Ctrl Pts',(-41.8047470584447,37.3338595396184,38.2333047247928));
#28980=CARTESIAN_POINT('Ctrl Pts',(-41.8100667283911,37.3395039167693,38.2372355505726));
#28981=CARTESIAN_POINT('Ctrl Pts',(-41.8153863983375,37.3451482939202,38.2411663763523));
#28982=CARTESIAN_POINT('Ctrl Pts',(-41.8206960006346,37.3508097906851,38.2450862443869));
#28983=CARTESIAN_POINT('Ctrl Pts',(-41.8259954630207,37.3564883300132,38.2489951013283));
#28984=CARTESIAN_POINT('Ctrl Pts',(-41.8312949254068,37.3621668693414,38.2529039582697));
#28985=CARTESIAN_POINT('Ctrl Pts',(-41.8365842478817,37.3678624512327,38.2568018041178));
#28986=CARTESIAN_POINT('Ctrl Pts',(-41.8418633584599,37.3735749981724,38.2606885858245));
#28987=CARTESIAN_POINT('Ctrl Pts',(-41.8471424690381,37.3792875451122,38.2645753675312));
#28988=CARTESIAN_POINT('Ctrl Pts',(-41.8524113677194,37.3850170571003,38.2684510850964));
#28989=CARTESIAN_POINT('Ctrl Pts',(-41.8576699827962,37.3907634561602,38.2723156857731));
#28990=CARTESIAN_POINT('Ctrl Pts',(-41.8629285978729,37.3965098552201,38.2761802864498));
#28991=CARTESIAN_POINT('Ctrl Pts',(-41.868176929345,37.4022731413517,38.2800337702378));
#28992=CARTESIAN_POINT('Ctrl Pts',(-41.8734149057845,37.408053236119,38.2838760846927));
#28993=CARTESIAN_POINT('Ctrl Pts',(-41.8786528822242,37.4138333308862,38.2877183991477));
#28994=CARTESIAN_POINT('Ctrl Pts',(-41.8838805036312,37.419630234289,38.2915495442695));
#28995=CARTESIAN_POINT('Ctrl Pts',(-41.8890976988597,37.4254438674336,38.2953694679178));
#28996=CARTESIAN_POINT('Ctrl Pts',(-41.8943148940882,37.4312575005782,38.299189391566));
#28997=CARTESIAN_POINT('Ctrl Pts',(-41.8995216631381,37.4370878634646,38.3029980937406));
#28998=CARTESIAN_POINT('Ctrl Pts',(-41.9047179351473,37.4429348767437,38.3067955226066));
#28999=CARTESIAN_POINT('Ctrl Pts',(-41.9099142071565,37.4487818900228,38.3105929514726));
#29000=CARTESIAN_POINT('Ctrl Pts',(-41.9150999821248,37.4546455536944,38.3143791070299));
#29001=CARTESIAN_POINT('Ctrl Pts',(-41.9202751894758,37.4605257879565,38.3181539377503));
#29002=CARTESIAN_POINT('Ctrl Pts',(-41.9254503968269,37.4664060222185,38.3219287684708));
#29003=CARTESIAN_POINT('Ctrl Pts',(-41.9306150365605,37.4723028270709,38.3256922743543));
#29004=CARTESIAN_POINT('Ctrl Pts',(-41.935769038388,37.4782161222602,38.329444404181));
#29005=CARTESIAN_POINT('Ctrl Pts',(-41.9409230402155,37.4841294174496,38.3331965340078));
#29006=CARTESIAN_POINT('Ctrl Pts',(-41.9460664041368,37.4900592029758,38.3369372877777));
#29007=CARTESIAN_POINT('Ctrl Pts',(-41.9511990601526,37.4960053981369,38.3406666145804));
#29008=CARTESIAN_POINT('Ctrl Pts',(-41.9563317161684,37.5019515932978,38.3443959413833));
#29009=CARTESIAN_POINT('Ctrl Pts',(-41.9614536642786,37.5079141980935,38.3481138412189));
#29010=CARTESIAN_POINT('Ctrl Pts',(-41.9665648347755,37.513893131375,38.3518202634881));
#29011=CARTESIAN_POINT('Ctrl Pts',(-41.9716760052724,37.5198720646565,38.3555266857574));
#29012=CARTESIAN_POINT('Ctrl Pts',(-41.9767763981558,37.5258673264238,38.3592216304602));
#29013=CARTESIAN_POINT('Ctrl Pts',(-41.9818659440114,37.5318788350836,38.3629050473097));
#29014=CARTESIAN_POINT('Ctrl Pts',(-41.9869600131636,37.5378956864276,38.366591737769));
#29015=CARTESIAN_POINT('Ctrl Pts',(-41.9920432159987,37.5439288135554,38.3702668798752));
#29016=CARTESIAN_POINT('Ctrl Pts',(-41.9971154832133,37.5499781342127,38.3739304235221));
#29017=CARTESIAN_POINT('Ctrl Pts',(-41.7412556908976,37.2732497013001,38.1946924203304));
#29018=CARTESIAN_POINT('Ctrl Pts',(-41.7471060557576,37.2792470623069,38.1990959835345));
#29019=CARTESIAN_POINT('Ctrl Pts',(-41.7529449143376,37.2852649304657,38.2034869040542));
#29020=CARTESIAN_POINT('Ctrl Pts',(-41.7587721741905,37.2913032105692,38.2078651124785));
#29021=CARTESIAN_POINT('Ctrl Pts',(-41.7645994340434,37.2973414906728,38.2122433209027));
#29022=CARTESIAN_POINT('Ctrl Pts',(-41.7704150951689,37.303400182721,38.2166088172313));
#29023=CARTESIAN_POINT('Ctrl Pts',(-41.7762190654829,37.3094791908675,38.220961532451));
#29024=CARTESIAN_POINT('Ctrl Pts',(-41.782023035797,37.315558199014,38.2253142476706));
#29025=CARTESIAN_POINT('Ctrl Pts',(-41.7878153152994,37.3216575232586,38.2296541817813));
#29026=CARTESIAN_POINT('Ctrl Pts',(-41.793595812272,37.3277770671187,38.2339812661699));
#29027=CARTESIAN_POINT('Ctrl Pts',(-41.7993763092447,37.3338966109788,38.2383083505585));
#29028=CARTESIAN_POINT('Ctrl Pts',(-41.8051450236875,37.3400363744543,38.2426225852248));
#29029=CARTESIAN_POINT('Ctrl Pts',(-41.8109018642511,37.3461962604293,38.2469239019583));
#29030=CARTESIAN_POINT('Ctrl Pts',(-41.8166587048148,37.3523561464043,38.2512252186917));
#29031=CARTESIAN_POINT('Ctrl Pts',(-41.8224036714991,37.3585361548787,38.2555136174921));
#29032=CARTESIAN_POINT('Ctrl Pts',(-41.8281366733266,37.3647361881066,38.259789030553));
#29033=CARTESIAN_POINT('Ctrl Pts',(-41.8338696751542,37.3709362213344,38.2640644436139));
#29034=CARTESIAN_POINT('Ctrl Pts',(-41.8395907121247,37.3771562793155,38.2683268709353));
#29035=CARTESIAN_POINT('Ctrl Pts',(-41.8452996936353,37.3833962636767,38.2725762451173));
#29036=CARTESIAN_POINT('Ctrl Pts',(-41.8510086751459,37.3896362480378,38.2768256192993));
#29037=CARTESIAN_POINT('Ctrl Pts',(-41.8567056011963,37.3958961587788,38.2810619403417));
#29038=CARTESIAN_POINT('Ctrl Pts',(-41.8623903815609,37.4021758969026,38.2852851412534));
#29039=CARTESIAN_POINT('Ctrl Pts',(-41.8680751619256,37.4084556350262,38.2895083421652));
#29040=CARTESIAN_POINT('Ctrl Pts',(-41.8737477966043,37.4147552005324,38.293718422946));
#29041=CARTESIAN_POINT('Ctrl Pts',(-41.8794081957515,37.4210744938026,38.2979153170154));
#29042=CARTESIAN_POINT('Ctrl Pts',(-41.8850685948987,37.4273937870729,38.3021122110849));
#29043=CARTESIAN_POINT('Ctrl Pts',(-41.8907167585142,37.4337328081071,38.3062959184427));
#29044=CARTESIAN_POINT('Ctrl Pts',(-41.8963525971356,37.440091456669,38.3104663729213));
#29045=CARTESIAN_POINT('Ctrl Pts',(-41.901988435757,37.446450105231,38.3146368273998));
#29046=CARTESIAN_POINT('Ctrl Pts',(-41.9076119493839,37.4528283813204,38.3187940289989));
#29047=CARTESIAN_POINT('Ctrl Pts',(-41.9132230489397,37.4592261840861,38.3229379119655));
#29048=CARTESIAN_POINT('Ctrl Pts',(-41.9188341484954,37.4656239868519,38.3270817949321));
#29049=CARTESIAN_POINT('Ctrl Pts',(-41.9244328339797,37.4720413162939,38.331212359266));
#29050=CARTESIAN_POINT('Ctrl Pts',(-41.9300190167042,37.4784780709492,38.3353295396313));
#29051=CARTESIAN_POINT('Ctrl Pts',(-41.9356051994287,37.4849148256045,38.3394467199965));
#29052=CARTESIAN_POINT('Ctrl Pts',(-41.9411788793932,37.4913710054729,38.3435505163928));
#29053=CARTESIAN_POINT('Ctrl Pts',(-41.9467399683006,37.4978465084832,38.3476408639029));
#29054=CARTESIAN_POINT('Ctrl Pts',(-41.952301057208,37.5043220114934,38.351731211413));
#29055=CARTESIAN_POINT('Ctrl Pts',(-41.9578495550581,37.5108168376451,38.3558081100369));
#29056=CARTESIAN_POINT('Ctrl Pts',(-41.9633853739478,37.5173308842615,38.3598714952779));
#29057=CARTESIAN_POINT('Ctrl Pts',(-41.9689211928374,37.523844930878,38.3639348805189));
#29058=CARTESIAN_POINT('Ctrl Pts',(-41.9744443327663,37.530378197959,38.3679847523771));
#29059=CARTESIAN_POINT('Ctrl Pts',(-41.9799547062282,37.5369305822254,38.3720210467789));
#29060=CARTESIAN_POINT('Ctrl Pts',(-41.98546507969,37.5434829664919,38.3760573411807));
#29061=CARTESIAN_POINT('Ctrl Pts',(-41.9909626866845,37.5500544679437,38.3800800581259));
#29062=CARTESIAN_POINT('Ctrl Pts',(-41.9964474401047,37.5566449827026,38.3840891339659));
#29063=CARTESIAN_POINT('Ctrl Pts',(-42.0019370680592,37.5632413547331,38.3881017728427));
#29064=CARTESIAN_POINT('Ctrl Pts',(-42.007413819582,37.5698567738815,38.3921007463564));
#29065=CARTESIAN_POINT('Ctrl Pts',(-42.0128776077367,37.5764911353951,38.3960859911166));
#29066=CARTESIAN_POINT('Ctrl Pts',(-41.7367328459062,37.2738705169503,38.1998157216697));
#29067=CARTESIAN_POINT('Ctrl Pts',(-41.7430280210025,37.2803585765446,38.2046103979808));
#29068=CARTESIAN_POINT('Ctrl Pts',(-41.7493097317734,37.2868706330318,38.209390280178));
#29069=CARTESIAN_POINT('Ctrl Pts',(-41.7555778617687,37.293406565812,38.214155279829));
#29070=CARTESIAN_POINT('Ctrl Pts',(-41.761845991764,37.2999424985921,38.21892027948));
#29071=CARTESIAN_POINT('Ctrl Pts',(-41.7681005409835,37.3065023076648,38.2236703965848));
#29072=CARTESIAN_POINT('Ctrl Pts',(-41.7743413934729,37.3130858715579,38.2284055432544));
#29073=CARTESIAN_POINT('Ctrl Pts',(-41.7805822459624,37.319669435451,38.2331406899241));
#29074=CARTESIAN_POINT('Ctrl Pts',(-41.7868094017216,37.3262767541642,38.2378608661586));
#29075=CARTESIAN_POINT('Ctrl Pts',(-41.7930227452966,37.3329077053572,38.2425659846159));
#29076=CARTESIAN_POINT('Ctrl Pts',(-41.7992360888717,37.3395386565503,38.2472711030733));
#29077=CARTESIAN_POINT('Ctrl Pts',(-41.8054356202623,37.3461932402229,38.2519611637533));
#29078=CARTESIAN_POINT('Ctrl Pts',(-41.8116212245189,37.3528713331714,38.256636079864));
#29079=CARTESIAN_POINT('Ctrl Pts',(-41.8178068287755,37.35954942612,38.2613109959747));
#29080=CARTESIAN_POINT('Ctrl Pts',(-41.8239785058979,37.3662510283441,38.2659707675158));
#29081=CARTESIAN_POINT('Ctrl Pts',(-41.8301361414449,37.3729760157812,38.2706153082483));
#29082=CARTESIAN_POINT('Ctrl Pts',(-41.8362937769919,37.3797010032182,38.2752598489809));
#29083=CARTESIAN_POINT('Ctrl Pts',(-41.8424373709633,37.3864493758679,38.2798891589046));
#29084=CARTESIAN_POINT('Ctrl Pts',(-41.8485668094307,37.3932210088127,38.2845031523365));
#29085=CARTESIAN_POINT('Ctrl Pts',(-41.8546962478981,37.3999926417575,38.2891171457685));
#29086=CARTESIAN_POINT('Ctrl Pts',(-41.8608115308611,37.4067875349973,38.2937158227084));
#29087=CARTESIAN_POINT('Ctrl Pts',(-41.866912544908,37.4136055627644,38.2982990980327));
#29088=CARTESIAN_POINT('Ctrl Pts',(-41.873013558955,37.4204235905314,38.3028823733569));
#29089=CARTESIAN_POINT('Ctrl Pts',(-41.8791003040856,37.4272647528256,38.3074502470652));
#29090=CARTESIAN_POINT('Ctrl Pts',(-41.8851726674089,37.4341289230337,38.3120026345959));
#29091=CARTESIAN_POINT('Ctrl Pts',(-41.8912450307322,37.4409930932418,38.3165550221266));
#29092=CARTESIAN_POINT('Ctrl Pts',(-41.897303012248,37.4478802713635,38.3210919234796));
#29093=CARTESIAN_POINT('Ctrl Pts',(-41.90334649959,37.4547903299445,38.3256132546585));
#29094=CARTESIAN_POINT('Ctrl Pts',(-41.9093899869321,37.4617003885256,38.3301345858374));
#29095=CARTESIAN_POINT('Ctrl Pts',(-41.9154189801002,37.4686333275657,38.3346403468421));
#29096=CARTESIAN_POINT('Ctrl Pts',(-41.9214333672572,37.4755890187741,38.3391304542444));
#29097=CARTESIAN_POINT('Ctrl Pts',(-41.9274477544141,37.4825447099826,38.3436205616467));
#29098=CARTESIAN_POINT('Ctrl Pts',(-41.9334475355597,37.489523153359,38.3480950154465));
#29099=CARTESIAN_POINT('Ctrl Pts',(-41.9394325993895,37.4965242197808,38.352553732787));
#29100=CARTESIAN_POINT('Ctrl Pts',(-41.9454176632194,37.5035252862025,38.3570124501275));
#29101=CARTESIAN_POINT('Ctrl Pts',(-41.9513880097333,37.5105489756694,38.3614554310084));
#29102=CARTESIAN_POINT('Ctrl Pts',(-41.9573435281639,37.5175951582312,38.3658825931472));
#29103=CARTESIAN_POINT('Ctrl Pts',(-41.9632990465945,37.5246413407931,38.370309755286));
#29104=CARTESIAN_POINT('Ctrl Pts',(-41.9692397369415,37.5317100164498,38.3747210986826));
#29105=CARTESIAN_POINT('Ctrl Pts',(-41.9751654889785,37.5388010544286,38.3791165416315));
#29106=CARTESIAN_POINT('Ctrl Pts',(-41.9810912410156,37.5458920924075,38.3835119845804));
#29107=CARTESIAN_POINT('Ctrl Pts',(-41.9870020547423,37.5530054927082,38.3878915270814));
#29108=CARTESIAN_POINT('Ctrl Pts',(-41.9928978204773,37.5601411237404,38.3922550880094));
#29109=CARTESIAN_POINT('Ctrl Pts',(-41.9987935862122,37.5672767547726,38.3966186489373));
#29110=CARTESIAN_POINT('Ctrl Pts',(-42.0046743039551,37.5744346165359,38.400966228292));
#29111=CARTESIAN_POINT('Ctrl Pts',(-42.0105398645732,37.5816145766264,38.4052977455312));
#29112=CARTESIAN_POINT('Ctrl Pts',(-42.0164106381653,37.5888009178539,38.4096331123744));
#29113=CARTESIAN_POINT('Ctrl Pts',(-42.0222662276787,37.5960093967053,38.4139523885391));
#29114=CARTESIAN_POINT('Ctrl Pts',(-42.0281065242439,37.603239879613,38.4182554938557));
#29115=CARTESIAN_POINT('Ctrl Pts',(-41.7321871653721,37.2744646741203,38.2049165643793));
#29116=CARTESIAN_POINT('Ctrl Pts',(-41.7389170723941,37.2814374382853,38.21010180357));
#29117=CARTESIAN_POINT('Ctrl Pts',(-41.7456313608748,37.2884380387103,38.2152698816723));
#29118=CARTESIAN_POINT('Ctrl Pts',(-41.7523298848223,37.2954663231777,38.2204206863142));
#29119=CARTESIAN_POINT('Ctrl Pts',(-41.7590284087698,37.3024946076452,38.2255714909562));
#29120=CARTESIAN_POINT('Ctrl Pts',(-41.7657111681836,37.3095505761549,38.2307050221375));
#29121=CARTESIAN_POINT('Ctrl Pts',(-41.7723780177576,37.3166340752856,38.2358211682374));
#29122=CARTESIAN_POINT('Ctrl Pts',(-41.7790448673315,37.3237175744162,38.2409373143374));
#29123=CARTESIAN_POINT('Ctrl Pts',(-41.785695807065,37.3308286041674,38.2460360753556));
#29124=CARTESIAN_POINT('Ctrl Pts',(-41.7923306923437,37.3379670099207,38.2511173404274));
#29125=CARTESIAN_POINT('Ctrl Pts',(-41.7989655776225,37.345105415674,38.2561986054992));
#29126=CARTESIAN_POINT('Ctrl Pts',(-41.805584408446,37.352271197429,38.2612623746243));
#29127=CARTESIAN_POINT('Ctrl Pts',(-41.8121870408979,37.3594641993769,38.2663085376988));
#29128=CARTESIAN_POINT('Ctrl Pts',(-41.8187896733498,37.3666572013247,38.2713547007732));
#29129=CARTESIAN_POINT('Ctrl Pts',(-41.8253761074299,37.3738774234648,38.2763832577968));
#29130=CARTESIAN_POINT('Ctrl Pts',(-41.831946199926,37.3811247088047,38.2813940994311));
#29131=CARTESIAN_POINT('Ctrl Pts',(-41.8385162924222,37.3883719941445,38.2864049410656));
#29132=CARTESIAN_POINT('Ctrl Pts',(-41.8450700433342,37.3956463426837,38.2913980673105));
#29133=CARTESIAN_POINT('Ctrl Pts',(-41.8516073101607,37.4029475962526,38.2963733695981));
#29134=CARTESIAN_POINT('Ctrl Pts',(-41.8581445769872,37.4102488498215,38.3013486718857));
#29135=CARTESIAN_POINT('Ctrl Pts',(-41.8646653597278,37.4175770084196,38.3063061502157));
#29136=CARTESIAN_POINT('Ctrl Pts',(-41.8711695165982,37.4249319127075,38.3112456967953));
#29137=CARTESIAN_POINT('Ctrl Pts',(-41.8776736734685,37.4322868169954,38.3161852433749));
#29138=CARTESIAN_POINT('Ctrl Pts',(-41.8841612044682,37.4396684669727,38.3211068582038));
#29139=CARTESIAN_POINT('Ctrl Pts',(-41.8906319685359,37.4470767021365,38.3260104342692));
#29140=CARTESIAN_POINT('Ctrl Pts',(-41.8971027326035,37.4544849373004,38.3309140103344));
#29141=CARTESIAN_POINT('Ctrl Pts',(-41.9035567297387,37.4619197576506,38.3357995476358));
#29142=CARTESIAN_POINT('Ctrl Pts',(-41.9099938196092,37.4693810015281,38.3406669399448));
#29143=CARTESIAN_POINT('Ctrl Pts',(-41.9164309094797,37.4768422454057,38.3455343322538));
#29144=CARTESIAN_POINT('Ctrl Pts',(-41.9228510920851,37.4843299128102,38.35038357957));
#29145=CARTESIAN_POINT('Ctrl Pts',(-41.9292542278285,37.491843840934,38.3552145764541));
#29146=CARTESIAN_POINT('Ctrl Pts',(-41.9356573635717,37.4993577690579,38.3600455733381));
#29147=CARTESIAN_POINT('Ctrl Pts',(-41.9420434524526,37.5068979579004,38.3648583197898));
#29148=CARTESIAN_POINT('Ctrl Pts',(-41.9484123556152,37.5144642435118,38.3696527111632));
#29149=CARTESIAN_POINT('Ctrl Pts',(-41.9547812587779,37.5220305291232,38.3744471025367));
#29150=CARTESIAN_POINT('Ctrl Pts',(-41.961132976222,37.5296229115031,38.3792231388316));
#29151=CARTESIAN_POINT('Ctrl Pts',(-41.9674673698392,37.5372412255669,38.3839807162004));
#29152=CARTESIAN_POINT('Ctrl Pts',(-41.9738017634564,37.5448595396305,38.3887382935692));
#29153=CARTESIAN_POINT('Ctrl Pts',(-41.9801188332463,37.5525037853775,38.3934774120117));
#29154=CARTESIAN_POINT('Ctrl Pts',(-41.986418441854,37.5601737965954,38.3981979684829));
#29155=CARTESIAN_POINT('Ctrl Pts',(-41.9927180504617,37.5678438078133,38.4029185249541));
#29156=CARTESIAN_POINT('Ctrl Pts',(-41.9990001978867,37.5755395845017,38.4076205194538));
#29157=CARTESIAN_POINT('Ctrl Pts',(-42.0052647475334,37.5832609593277,38.4123038497444));
#29158=CARTESIAN_POINT('Ctrl Pts',(-42.0115292971802,37.5909823341538,38.416987180035));
#29159=CARTESIAN_POINT('Ctrl Pts',(-42.0177762490482,37.5987293071169,38.4216518461161));
#29160=CARTESIAN_POINT('Ctrl Pts',(-42.0240054673073,37.6065017097712,38.4262977465618));
#29161=CARTESIAN_POINT('Ctrl Pts',(-42.0302402217383,37.6142810200913,38.4309477760174));
#29162=CARTESIAN_POINT('Ctrl Pts',(-42.0364572110247,37.6220858053229,38.4355790064668));
#29163=CARTESIAN_POINT('Ctrl Pts',(-42.0426562997468,37.6299158954619,38.4401913370316));
#29164=CARTESIAN_POINT('Ctrl Pts',(-41.7276414848379,37.2750588312903,38.2100174070889));
#29165=CARTESIAN_POINT('Ctrl Pts',(-41.7348061237857,37.282516300026,38.2155932091592));
#29166=CARTESIAN_POINT('Ctrl Pts',(-41.7419529899762,37.2900054443886,38.2211494831666));
#29167=CARTESIAN_POINT('Ctrl Pts',(-41.7490819078759,37.2975260805435,38.2266860927995));
#29168=CARTESIAN_POINT('Ctrl Pts',(-41.7562108257756,37.3050467166984,38.2322227024323));
#29169=CARTESIAN_POINT('Ctrl Pts',(-41.7633217953838,37.312598844645,38.2377396476902));
#29170=CARTESIAN_POINT('Ctrl Pts',(-41.7704146420422,37.3201822790132,38.2432367932204));
#29171=CARTESIAN_POINT('Ctrl Pts',(-41.7775074887006,37.3277657133814,38.2487339387506));
#29172=CARTESIAN_POINT('Ctrl Pts',(-41.7845822124084,37.3353804541706,38.2542112845526));
#29173=CARTESIAN_POINT('Ctrl Pts',(-41.7916386393909,37.3430263144842,38.2596686962389));
#29174=CARTESIAN_POINT('Ctrl Pts',(-41.7986950663732,37.3506721747979,38.2651261079251));
#29175=CARTESIAN_POINT('Ctrl Pts',(-41.8057331966296,37.3583491546353,38.2705635854952));
#29176=CARTESIAN_POINT('Ctrl Pts',(-41.8127528572769,37.3660570655823,38.2759809955335));
#29177=CARTESIAN_POINT('Ctrl Pts',(-41.8197725179242,37.3737649765293,38.2813984055718));
#29178=CARTESIAN_POINT('Ctrl Pts',(-41.8267737089618,37.3815038185855,38.2867957480777));
#29179=CARTESIAN_POINT('Ctrl Pts',(-41.8337562584072,37.3892734018282,38.292172890614));
#29180=CARTESIAN_POINT('Ctrl Pts',(-41.8407388078525,37.3970429850708,38.2975500331503));
#29181=CARTESIAN_POINT('Ctrl Pts',(-41.847702715705,37.4048433094995,38.3029069757164));
#29182=CARTESIAN_POINT('Ctrl Pts',(-41.8546478108907,37.4126741836924,38.3082435868597));
#29183=CARTESIAN_POINT('Ctrl Pts',(-41.8615929060763,37.4205050578853,38.3135801980029));
#29184=CARTESIAN_POINT('Ctrl Pts',(-41.8685191885945,37.4283664818419,38.3188964777229));
#29185=CARTESIAN_POINT('Ctrl Pts',(-41.8754264882883,37.4362582626507,38.3241922955579));
#29186=CARTESIAN_POINT('Ctrl Pts',(-41.8823337879821,37.4441500434594,38.3294881133929));
#29187=CARTESIAN_POINT('Ctrl Pts',(-41.8892221048508,37.4520721811197,38.3347634693425));
#29188=CARTESIAN_POINT('Ctrl Pts',(-41.8960912696628,37.4600244812394,38.3400182339424));
#29189=CARTESIAN_POINT('Ctrl Pts',(-41.9029604344748,37.4679767813591,38.3452729985423));
#29190=CARTESIAN_POINT('Ctrl Pts',(-41.9098104472295,37.4759592439376,38.3505071717921));
#29191=CARTESIAN_POINT('Ctrl Pts',(-41.9166411396284,37.4839716731117,38.3557206252311));
#29192=CARTESIAN_POINT('Ctrl Pts',(-41.9234718320273,37.4919841022858,38.3609340786701));
#29193=CARTESIAN_POINT('Ctrl Pts',(-41.93028320407,37.5000264980549,38.3661268122979));
#29194=CARTESIAN_POINT('Ctrl Pts',(-41.9370750883997,37.508098663094,38.3712986986637));
#29195=CARTESIAN_POINT('Ctrl Pts',(-41.9438669727293,37.5161708281332,38.3764705850296));
#29196=CARTESIAN_POINT('Ctrl Pts',(-41.9506393693455,37.5242727624417,38.3816216241331));
#29197=CARTESIAN_POINT('Ctrl Pts',(-41.9573921118409,37.5324042672428,38.3867516895395));
#29198=CARTESIAN_POINT('Ctrl Pts',(-41.9641448543364,37.5405357720439,38.3918817549459));
#29199=CARTESIAN_POINT('Ctrl Pts',(-41.9708779427107,37.548696847337,38.3969908466547));
#29200=CARTESIAN_POINT('Ctrl Pts',(-41.9775912115145,37.5568872929024,38.4020788392536));
#29201=CARTESIAN_POINT('Ctrl Pts',(-41.9843044803183,37.5650777384679,38.4071668318524));
#29202=CARTESIAN_POINT('Ctrl Pts',(-41.9909979295511,37.5732975543052,38.4122337253407));
#29203=CARTESIAN_POINT('Ctrl Pts',(-41.9976713947294,37.5815465387622,38.4172793953343));
#29204=CARTESIAN_POINT('Ctrl Pts',(-42.0043448599078,37.5897955232191,38.4223250653279));
#29205=CARTESIAN_POINT('Ctrl Pts',(-42.010998341031,37.5980736762952,38.4273495118262));
#29206=CARTESIAN_POINT('Ctrl Pts',(-42.0176316745896,37.606380794915,38.4323526114794));
#29207=CARTESIAN_POINT('Ctrl Pts',(-42.0242650081481,37.6146879135349,38.4373557111327));
#29208=CARTESIAN_POINT('Ctrl Pts',(-42.0308781941414,37.6230239976979,38.4423374639403));
#29209=CARTESIAN_POINT('Ctrl Pts',(-42.0374710700414,37.6313888429159,38.4472977475925));
#29210=CARTESIAN_POINT('Ctrl Pts',(-42.0440698053114,37.6397611223286,38.4522624396604));
#29211=CARTESIAN_POINT('Ctrl Pts',(-42.0506481943707,37.6481622139406,38.4572056243945));
#29212=CARTESIAN_POINT('Ctrl Pts',(-42.0572060752497,37.6565919113109,38.4621271802075));
#29213=CARTESIAN_POINT('Ctrl Pts',(-41.7230729915867,37.275626356627,38.2150958136178));
#29214=CARTESIAN_POINT('Ctrl Pts',(-41.7306622893052,37.2835625164353,38.2210615920481));
#29215=CARTESIAN_POINT('Ctrl Pts',(-41.7382314646438,37.2915345395025,38.2270052607349));
#29216=CARTESIAN_POINT('Ctrl Pts',(-41.7457803069961,37.299542204158,38.2329266545113));
#29217=CARTESIAN_POINT('Ctrl Pts',(-41.7533291493484,37.3075498688135,38.2388480482876));
#29218=CARTESIAN_POINT('Ctrl Pts',(-41.7608576587077,37.3155931750479,38.2447471671446));
#29219=CARTESIAN_POINT('Ctrl Pts',(-41.7683656255999,37.3236718992408,38.2506238471586));
#29220=CARTESIAN_POINT('Ctrl Pts',(-41.7758735924921,37.3317506234335,38.2565005271726));
#29221=CARTESIAN_POINT('Ctrl Pts',(-41.7833610169126,37.3398647655783,38.2623547683379));
#29222=CARTESIAN_POINT('Ctrl Pts',(-41.790827690507,37.3480141000814,38.2681864079499));
#29223=CARTESIAN_POINT('Ctrl Pts',(-41.7982943641013,37.3561634345845,38.2740180475619));
#29224=CARTESIAN_POINT('Ctrl Pts',(-41.8057402868683,37.3643479614441,38.2798270856192));
#29225=CARTESIAN_POINT('Ctrl Pts',(-41.8131652516029,37.3725674531331,38.2856133606714));
#29226=CARTESIAN_POINT('Ctrl Pts',(-41.8205902163375,37.3807869448222,38.2913996357236));
#29227=CARTESIAN_POINT('Ctrl Pts',(-41.8279942230375,37.3890414013376,38.297163147768));
#29228=CARTESIAN_POINT('Ctrl Pts',(-41.8353770656508,37.3973305932187,38.3029037366049));
#29229=CARTESIAN_POINT('Ctrl Pts',(-41.842759908264,37.4056197850998,38.3086443254418));
#29230=CARTESIAN_POINT('Ctrl Pts',(-41.8501215867896,37.4139437123456,38.3143619910705));
#29231=CARTESIAN_POINT('Ctrl Pts',(-41.8574618963422,37.4223021435787,38.3200565745555));
#29232=CARTESIAN_POINT('Ctrl Pts',(-41.8648022058947,37.4306605748119,38.3257511580404));
#29233=CARTESIAN_POINT('Ctrl Pts',(-41.8721211464735,37.4390535100316,38.3314226593808));
#29234=CARTESIAN_POINT('Ctrl Pts',(-41.8794185143709,37.4474807159566,38.3370709209135));
#29235=CARTESIAN_POINT('Ctrl Pts',(-41.8867158822685,37.4559079218816,38.3427191824463));
#29236=CARTESIAN_POINT('Ctrl Pts',(-41.893991677484,37.464369398511,38.3483442041708));
#29237=CARTESIAN_POINT('Ctrl Pts',(-41.9012456974993,37.4728649106725,38.3539458297051));
#29238=CARTESIAN_POINT('Ctrl Pts',(-41.9084997175147,37.481360422834,38.3595474552394));
#29239=CARTESIAN_POINT('Ctrl Pts',(-41.9157319623291,37.4898899705267,38.3651256845829));
#29240=CARTESIAN_POINT('Ctrl Pts',(-41.9229422306246,37.4984533167,38.3706803626433));
#29241=CARTESIAN_POINT('Ctrl Pts',(-41.9301524989203,37.5070166628732,38.3762350407038));
#29242=CARTESIAN_POINT('Ctrl Pts',(-41.9373407906963,37.5156138075261,38.3817661674807));
#29243=CARTESIAN_POINT('Ctrl Pts',(-41.9445069058461,37.5242445117427,38.38727358918));
#29244=CARTESIAN_POINT('Ctrl Pts',(-41.9516730209959,37.5328752159593,38.3927810108792));
#29245=CARTESIAN_POINT('Ctrl Pts',(-41.9588169595188,37.5415394797386,38.3982647275003));
#29246=CARTESIAN_POINT('Ctrl Pts',(-41.9659385225304,37.5502370623123,38.4037245865559));
#29247=CARTESIAN_POINT('Ctrl Pts',(-41.9730600855419,37.5589346448861,38.4091844456114));
#29248=CARTESIAN_POINT('Ctrl Pts',(-41.9801592730415,37.5676655462534,38.4146204471008));
#29249=CARTESIAN_POINT('Ctrl Pts',(-41.9872358873777,37.5764295238067,38.4200324398517));
#29250=CARTESIAN_POINT('Ctrl Pts',(-41.994312501714,37.5851935013599,38.4254444326026));
#29251=CARTESIAN_POINT('Ctrl Pts',(-42.0013665428862,37.5939905550983,38.4308324166144));
#29252=CARTESIAN_POINT('Ctrl Pts',(-42.0083978144872,37.6028204405884,38.4361962420379));
#29253=CARTESIAN_POINT('Ctrl Pts',(-42.0154290860881,37.6116503260784,38.4415600674614));
#29254=CARTESIAN_POINT('Ctrl Pts',(-42.0224375881171,37.6205130433192,38.446899734296));
#29255=CARTESIAN_POINT('Ctrl Pts',(-42.0294231254213,37.6294083460648,38.4522150940239));
#29256=CARTESIAN_POINT('Ctrl Pts',(-42.0364086627255,37.6383036488102,38.4575304537519));
#29257=CARTESIAN_POINT('Ctrl Pts',(-42.0433712353044,37.6472315370596,38.4628215063726));
#29258=CARTESIAN_POINT('Ctrl Pts',(-42.0503106492707,37.6561917627675,38.4680881047078));
#29259=CARTESIAN_POINT('Ctrl Pts',(-42.0572562305902,37.6651599518102,38.4733593836936));
#29260=CARTESIAN_POINT('Ctrl Pts',(-42.0641786121495,37.6741605358844,38.4786061649633));
#29261=CARTESIAN_POINT('Ctrl Pts',(-42.0710776007528,37.6831932643562,38.4838283021851));
#29262=CARTESIAN_POINT('Ctrl Pts',(-41.7184851250818,37.2761712654004,38.2201551666592));
#29263=CARTESIAN_POINT('Ctrl Pts',(-41.7264872714304,37.2845766395827,38.2265062982766));
#29264=CARTESIAN_POINT('Ctrl Pts',(-41.7344667883464,37.2930223452366,38.2328325654919));
#29265=CARTESIAN_POINT('Ctrl Pts',(-41.7424234244465,37.3015081162923,38.239133769005));
#29266=CARTESIAN_POINT('Ctrl Pts',(-41.7503800605466,37.3099938873479,38.2454349725181));
#29267=CARTESIAN_POINT('Ctrl Pts',(-41.7583138158242,37.3185197237962,38.2517111123206));
#29268=CARTESIAN_POINT('Ctrl Pts',(-41.7662244403479,37.3270853570574,38.2579619907056));
#29269=CARTESIAN_POINT('Ctrl Pts',(-41.7741350648715,37.3356509903186,38.2642128690906));
#29270=CARTESIAN_POINT('Ctrl Pts',(-41.7820225586366,37.3442564203866,38.2704384860526));
#29271=CARTESIAN_POINT('Ctrl Pts',(-41.7898866731567,37.3529013761564,38.2766386454592));
#29272=CARTESIAN_POINT('Ctrl Pts',(-41.7977507876768,37.3615463319261,38.2828388048658));
#29273=CARTESIAN_POINT('Ctrl Pts',(-41.8055915229504,37.3702308133956,38.2890135067153));
#29274=CARTESIAN_POINT('Ctrl Pts',(-41.8134086319691,37.378954546977,38.2951625564871));
#29275=CARTESIAN_POINT('Ctrl Pts',(-41.8212257409878,37.3876782805585,38.3013116062587));
#29276=CARTESIAN_POINT('Ctrl Pts',(-41.8290192237492,37.3964412662486,38.3074350039495));
#29277=CARTESIAN_POINT('Ctrl Pts',(-41.8367888347307,37.4052432279819,38.3135325566508));
#29278=CARTESIAN_POINT('Ctrl Pts',(-41.8445584457122,37.4140451897154,38.319630109352));
#29279=CARTESIAN_POINT('Ctrl Pts',(-41.8523041849128,37.4228861274909,38.3257018170627));
#29280=CARTESIAN_POINT('Ctrl Pts',(-41.860025808314,37.4317657627873,38.3317474885023));
#29281=CARTESIAN_POINT('Ctrl Pts',(-41.8677474317152,37.4406453980838,38.337793159942));
#29282=CARTESIAN_POINT('Ctrl Pts',(-41.875444939316,37.4495637309,38.3438127951099));
#29283=CARTESIAN_POINT('Ctrl Pts',(-41.8831180886173,37.4585204802766,38.3498062043658));
#29284=CARTESIAN_POINT('Ctrl Pts',(-41.8907912379186,37.4674772296532,38.3557996136218));
#29285=CARTESIAN_POINT('Ctrl Pts',(-41.8984400289194,37.476472395589,38.361766796965));
#29286=CARTESIAN_POINT('Ctrl Pts',(-41.9060642206555,37.485505694704,38.367707566408));
#29287=CARTESIAN_POINT('Ctrl Pts',(-41.9136884123916,37.494538993819,38.373648335851));
#29288=CARTESIAN_POINT('Ctrl Pts',(-41.9212880048618,37.5036104261121,38.3795626913929));
#29289=CARTESIAN_POINT('Ctrl Pts',(-41.928862758652,37.5127197058007,38.3854504467104));
#29290=CARTESIAN_POINT('Ctrl Pts',(-41.9364375124421,37.5218289854894,38.3913382020278));
#29291=CARTESIAN_POINT('Ctrl Pts',(-41.9439874275511,37.5309761125723,38.39719935712));
#29292=CARTESIAN_POINT('Ctrl Pts',(-41.9515122661296,37.5401607988822,38.4030337273397));
#29293=CARTESIAN_POINT('Ctrl Pts',(-41.9590371047082,37.5493454851921,38.4088680975593));
#29294=CARTESIAN_POINT('Ctrl Pts',(-41.9665368667552,37.5585677307279,38.4146756829056));
#29295=CARTESIAN_POINT('Ctrl Pts',(-41.9740113160014,37.5678272449558,38.4204563004188));
#29296=CARTESIAN_POINT('Ctrl Pts',(-41.9814857652477,37.5770867591837,38.426236917932));
#29297=CARTESIAN_POINT('Ctrl Pts',(-41.9889349016921,37.5863835421024,38.4319905676113));
#29298=CARTESIAN_POINT('Ctrl Pts',(-41.9963584906603,37.5957173008301,38.4377170681963));
#29299=CARTESIAN_POINT('Ctrl Pts',(-42.0037820796284,37.6050510595578,38.4434435687812));
#29300=CARTESIAN_POINT('Ctrl Pts',(-42.0111801211193,37.6144217940933,38.449142920271));
#29301=CARTESIAN_POINT('Ctrl Pts',(-42.0185523820682,37.6238292092247,38.4548149431157));
#29302=CARTESIAN_POINT('Ctrl Pts',(-42.0259246430171,37.6332366243561,38.4604869659604));
#29303=CARTESIAN_POINT('Ctrl Pts',(-42.033271123423,37.6426807200824,38.4661316601591));
#29304=CARTESIAN_POINT('Ctrl Pts',(-42.0405915918455,37.6521611988806,38.471748847884));
#29305=CARTESIAN_POINT('Ctrl Pts',(-42.0479120602679,37.6616416776789,38.4773660356088));
#29306=CARTESIAN_POINT('Ctrl Pts',(-42.055206516706,37.6711585395479,38.482955716859));
#29307=CARTESIAN_POINT('Ctrl Pts',(-42.0624747313583,37.6807114846723,38.4885177155396));
#29308=CARTESIAN_POINT('Ctrl Pts',(-42.0697494055828,37.6902729199067,38.4940846574055));
#29309=CARTESIAN_POINT('Ctrl Pts',(-42.0769977913877,37.6998705026253,38.499623867526));
#29310=CARTESIAN_POINT('Ctrl Pts',(-42.084219659952,37.7095039298065,38.5051351709817));
#29311=CARTESIAN_POINT('Ctrl Pts',(-41.7138972585769,37.2767161741738,38.2252145197005));
#29312=CARTESIAN_POINT('Ctrl Pts',(-41.7223122535556,37.2855907627301,38.2319510045052));
#29313=CARTESIAN_POINT('Ctrl Pts',(-41.730702112049,37.2945101509708,38.2386598702489));
#29314=CARTESIAN_POINT('Ctrl Pts',(-41.7390665418968,37.3034740284267,38.2453408834987));
#29315=CARTESIAN_POINT('Ctrl Pts',(-41.7474309717446,37.3124379058824,38.2520218967486));
#29316=CARTESIAN_POINT('Ctrl Pts',(-41.7557699729406,37.3214462725444,38.2586750574966));
#29317=CARTESIAN_POINT('Ctrl Pts',(-41.7640832550958,37.3304988148741,38.2653001342526));
#29318=CARTESIAN_POINT('Ctrl Pts',(-41.7723965372509,37.3395513572038,38.2719252110086));
#29319=CARTESIAN_POINT('Ctrl Pts',(-41.7806841003605,37.3486480751949,38.2785222037673));
#29320=CARTESIAN_POINT('Ctrl Pts',(-41.7889456558064,37.3577886522314,38.2850908829684));
#29321=CARTESIAN_POINT('Ctrl Pts',(-41.7972072112522,37.3669292292677,38.2916595621696));
#29322=CARTESIAN_POINT('Ctrl Pts',(-41.8054427590326,37.3761136653472,38.2981999278115));
#29323=CARTESIAN_POINT('Ctrl Pts',(-41.8136520123354,37.3853416408209,38.3047117523027));
#29324=CARTESIAN_POINT('Ctrl Pts',(-41.8218612656381,37.3945696162947,38.3112235767938));
#29325=CARTESIAN_POINT('Ctrl Pts',(-41.8300442244608,37.4038411311594,38.3177068601312));
#29326=CARTESIAN_POINT('Ctrl Pts',(-41.8382006038106,37.4131558627451,38.3241613766967));
#29327=CARTESIAN_POINT('Ctrl Pts',(-41.8463569831605,37.4224705943309,38.3306158932622));
#29328=CARTESIAN_POINT('Ctrl Pts',(-41.8544867830361,37.4318285426362,38.3370416430548));
#29329=CARTESIAN_POINT('Ctrl Pts',(-41.8625897202859,37.4412293819959,38.3434384024493));
#29330=CARTESIAN_POINT('Ctrl Pts',(-41.8706926575358,37.4506302213557,38.3498351618437));
#29331=CARTESIAN_POINT('Ctrl Pts',(-41.8787687321586,37.4600739517684,38.3562029308389));
#29332=CARTESIAN_POINT('Ctrl Pts',(-41.8868176628637,37.4695602445966,38.3625414878181));
#29333=CARTESIAN_POINT('Ctrl Pts',(-41.8948665935688,37.4790465374248,38.3688800447972));
#29334=CARTESIAN_POINT('Ctrl Pts',(-41.9028883803549,37.488575392667,38.3751893897593));
#29335=CARTESIAN_POINT('Ctrl Pts',(-41.9108827438117,37.4981464787355,38.381469303111));
#29336=CARTESIAN_POINT('Ctrl Pts',(-41.9188771072685,37.507717564804,38.3877492164627));
#29337=CARTESIAN_POINT('Ctrl Pts',(-41.9268440473946,37.5173308816975,38.393999698203));
#29338=CARTESIAN_POINT('Ctrl Pts',(-41.9347832866793,37.5269860949015,38.4002205307774));
#29339=CARTESIAN_POINT('Ctrl Pts',(-41.942722525964,37.5366413081055,38.4064413633518));
#29340=CARTESIAN_POINT('Ctrl Pts',(-41.950634064406,37.5463384176184,38.4126325467594));
#29341=CARTESIAN_POINT('Ctrl Pts',(-41.9585176264132,37.5560770860217,38.4187938654994));
#29342=CARTESIAN_POINT('Ctrl Pts',(-41.9664011884204,37.565815754425,38.4249551842394));
#29343=CARTESIAN_POINT('Ctrl Pts',(-41.9742567739916,37.5755959817172,38.4310866383109));
#29344=CARTESIAN_POINT('Ctrl Pts',(-41.9820841094725,37.5854174275992,38.4371880142817));
#29345=CARTESIAN_POINT('Ctrl Pts',(-41.9899114449534,37.5952388734812,38.4432893902526));
#29346=CARTESIAN_POINT('Ctrl Pts',(-41.9977105303427,37.6051015379515,38.4493606881218));
#29347=CARTESIAN_POINT('Ctrl Pts',(-42.0054810939427,37.6150050778536,38.4554016965408));
#29348=CARTESIAN_POINT('Ctrl Pts',(-42.0132516575428,37.6249086177557,38.4614427049598));
#29349=CARTESIAN_POINT('Ctrl Pts',(-42.0209936993524,37.6348530330882,38.4674534239276));
#29350=CARTESIAN_POINT('Ctrl Pts',(-42.0287069496492,37.644837977861,38.4734336441935));
#29351=CARTESIAN_POINT('Ctrl Pts',(-42.0364201999461,37.6548229226339,38.4794138644593));
#29352=CARTESIAN_POINT('Ctrl Pts',(-42.044104658729,37.6648483968455,38.4853635860223));
#29353=CARTESIAN_POINT('Ctrl Pts',(-42.0517600582697,37.6749140516966,38.491282601744));
#29354=CARTESIAN_POINT('Ctrl Pts',(-42.0594154578104,37.6849797065475,38.4972016174658));
#29355=CARTESIAN_POINT('Ctrl Pts',(-42.0670417981077,37.6950855420361,38.5030899273454));
#29356=CARTESIAN_POINT('Ctrl Pts',(-42.0746388134458,37.7052312065772,38.5089473263713));
#29357=CARTESIAN_POINT('Ctrl Pts',(-42.0822425805756,37.7153858880031,38.5148099311175));
#29358=CARTESIAN_POINT('Ctrl Pts',(-42.0898169706259,37.725580469366,38.5206415700889));
#29359=CARTESIAN_POINT('Ctrl Pts',(-42.0973617191512,37.7358145952567,38.5264420397782));
#29360=CARTESIAN_POINT('Ctrl Pts',(-41.7092900287824,37.2772384780159,38.2302548290539));
#29361=CARTESIAN_POINT('Ctrl Pts',(-41.7181061010845,37.2865728382894,38.2373720637469));
#29362=CARTESIAN_POINT('Ctrl Pts',(-41.7268943728444,37.2959567462818,38.2444587522097));
#29363=CARTESIAN_POINT('Ctrl Pts',(-41.7356545054327,37.3053898405726,38.2515146216083));
#29364=CARTESIAN_POINT('Ctrl Pts',(-41.7444146380209,37.3148229348634,38.2585704910069));
#29365=CARTESIAN_POINT('Ctrl Pts',(-41.7531466314358,37.3243052154509,38.2655955413399));
#29366=CARTESIAN_POINT('Ctrl Pts',(-41.7618501492037,37.3338363171455,38.2725895021348));
#29367=CARTESIAN_POINT('Ctrl Pts',(-41.7705536669717,37.3433674188402,38.2795834629297));
#29368=CARTESIAN_POINT('Ctrl Pts',(-41.7792287090911,37.35294734164,38.2865463341851));
#29369=CARTESIAN_POINT('Ctrl Pts',(-41.7878749412702,37.3625757166143,38.2934778478106));
#29370=CARTESIAN_POINT('Ctrl Pts',(-41.7965211734494,37.3722040915885,38.3004093614361));
#29371=CARTESIAN_POINT('Ctrl Pts',(-41.8051385956866,37.3818809187351,38.3073095174303));
#29372=CARTESIAN_POINT('Ctrl Pts',(-41.8137268758974,37.39160582541,38.3141780501053));
#29373=CARTESIAN_POINT('Ctrl Pts',(-41.8223151561082,37.4013307320849,38.3210465827803));
#29374=CARTESIAN_POINT('Ctrl Pts',(-41.8308742942908,37.4111037182862,38.3278834921346));
#29375=CARTESIAN_POINT('Ctrl Pts',(-41.8394039605935,37.4209244076846,38.3346885149031));
#29376=CARTESIAN_POINT('Ctrl Pts',(-41.8479336268961,37.4307450970831,38.3414935376716));
#29377=CARTESIAN_POINT('Ctrl Pts',(-41.8564338213171,37.4406134896769,38.3482666738529));
#29378=CARTESIAN_POINT('Ctrl Pts',(-41.8649042162621,37.4505292054806,38.3550076626245));
#29379=CARTESIAN_POINT('Ctrl Pts',(-41.8733746112071,37.4604449212843,38.361748651396));
#29380=CARTESIAN_POINT('Ctrl Pts',(-41.8818152066744,37.4704079602961,38.3684574927564));
#29381=CARTESIAN_POINT('Ctrl Pts',(-41.8902256773526,37.4804179389031,38.3751339283459));
#29382=CARTESIAN_POINT('Ctrl Pts',(-41.8986361480308,37.4904279175102,38.3818103639354));
#29383=CARTESIAN_POINT('Ctrl Pts',(-41.9070164939181,37.5004848357108,38.3884543937525));
#29384=CARTESIAN_POINT('Ctrl Pts',(-41.9153663920104,37.5105883062938,38.3950657619197));
#29385=CARTESIAN_POINT('Ctrl Pts',(-41.9237162901027,37.520691776877,38.401677130087));
#29386=CARTESIAN_POINT('Ctrl Pts',(-41.9320357409245,37.530841800794,38.4082558374545));
#29387=CARTESIAN_POINT('Ctrl Pts',(-41.9403244227673,37.5410379853954,38.4148016289715));
#29388=CARTESIAN_POINT('Ctrl Pts',(-41.9486131046101,37.5512341699968,38.4213474204885));
#29389=CARTESIAN_POINT('Ctrl Pts',(-41.9568710179807,37.5614765161947,38.4278602969742));
#29390=CARTESIAN_POINT('Ctrl Pts',(-41.9650978445669,37.5717646296768,38.4343400075791));
#29391=CARTESIAN_POINT('Ctrl Pts',(-41.9733246711531,37.5820527431589,38.4408197181839));
#29392=CARTESIAN_POINT('Ctrl Pts',(-41.9815204109533,37.5923866239237,38.447266262907));
#29393=CARTESIAN_POINT('Ctrl Pts',(-41.9896847480295,37.6027658741374,38.453679393428));
#29394=CARTESIAN_POINT('Ctrl Pts',(-41.9978490851056,37.6131451243512,38.4600925239489));
#29395=CARTESIAN_POINT('Ctrl Pts',(-42.0059820194561,37.6235697440116,38.4664722402663));
#29396=CARTESIAN_POINT('Ctrl Pts',(-42.0140832375544,37.6340393318199,38.4728182966305));
#29397=CARTESIAN_POINT('Ctrl Pts',(-42.0221844556527,37.6445089196283,38.4791643529947));
#29398=CARTESIAN_POINT('Ctrl Pts',(-42.0302539574975,37.6550234755828,38.4854767494049));
#29399=CARTESIAN_POINT('Ctrl Pts',(-42.038291431984,37.6655825949225,38.4917552426768));
#29400=CARTESIAN_POINT('Ctrl Pts',(-42.0463289064706,37.6761417142622,38.4980337359487));
#29401=CARTESIAN_POINT('Ctrl Pts',(-42.0543343535991,37.6867453969885,38.5042783260844));
#29402=CARTESIAN_POINT('Ctrl Pts',(-42.0623074647211,37.6973932349308,38.5104887725025));
#29403=CARTESIAN_POINT('Ctrl Pts',(-42.070280575843,37.7080410728731,38.5166992189205));
#29404=CARTESIAN_POINT('Ctrl Pts',(-42.0782213509548,37.7187330660247,38.5228755216161));
#29405=CARTESIAN_POINT('Ctrl Pts',(-42.0861294838881,37.7294688028375,38.5290174426298));
#29406=CARTESIAN_POINT('Ctrl Pts',(-42.0940446451165,37.7402140809574,38.5351648222307));
#29407=CARTESIAN_POINT('Ctrl Pts',(-42.1019271052873,37.7510031787688,38.5412777575933));
#29408=CARTESIAN_POINT('Ctrl Pts',(-42.1097765615633,37.7618356837186,38.5473560155564));
#29409=CARTESIAN_POINT('Ctrl Pts',(-41.7046664632442,37.2777417113195,38.2352790722939));
#29410=CARTESIAN_POINT('Ctrl Pts',(-41.7138715660119,37.2875248501967,38.242770189431));
#29411=CARTESIAN_POINT('Ctrl Pts',(-41.7230460825938,37.2973625015263,38.2502276995733));
#29412=CARTESIAN_POINT('Ctrl Pts',(-41.7321896223355,37.3072542464174,38.2576512851773));
#29413=CARTESIAN_POINT('Ctrl Pts',(-41.7413331620773,37.3171459913084,38.2650748707813));
#29414=CARTESIAN_POINT('Ctrl Pts',(-41.7504457249767,37.3270918297587,38.2724645318453));
#29415=CARTESIAN_POINT('Ctrl Pts',(-41.7595269230176,37.3370913382707,38.2798199537147));
#29416=CARTESIAN_POINT('Ctrl Pts',(-41.7686081210585,37.3470908467828,38.2871753755842));
#29417=CARTESIAN_POINT('Ctrl Pts',(-41.7776579542388,37.3571440253542,38.2944965582575));
#29418=CARTESIAN_POINT('Ctrl Pts',(-41.7866760372132,37.3672504459171,38.3017831899959));
#29419=CARTESIAN_POINT('Ctrl Pts',(-41.7956941201876,37.37735686648,38.3090698217343));
#29420=CARTESIAN_POINT('Ctrl Pts',(-41.8046804529541,37.3875165290319,38.3163219025361));
#29421=CARTESIAN_POINT('Ctrl Pts',(-41.8136346528712,37.3977290009708,38.3235391236051));
#29422=CARTESIAN_POINT('Ctrl Pts',(-41.8225888527884,37.4079414729097,38.3307563446742));
#29423=CARTESIAN_POINT('Ctrl Pts',(-41.8315109198541,37.4182067542331,38.3379387060087));
#29424=CARTESIAN_POINT('Ctrl Pts',(-41.8404004741637,37.4285244078417,38.3450859017813));
#29425=CARTESIAN_POINT('Ctrl Pts',(-41.8492900284732,37.4388420614502,38.3522330975538));
#29426=CARTESIAN_POINT('Ctrl Pts',(-41.8581470700244,37.4492120873415,38.3593451277626));
#29427=CARTESIAN_POINT('Ctrl Pts',(-41.8669712216812,37.4596340439559,38.3664216895748));
#29428=CARTESIAN_POINT('Ctrl Pts',(-41.875795373338,37.4700560005704,38.3734982513871));
#29429=CARTESIAN_POINT('Ctrl Pts',(-41.8845866350983,37.4805298879057,38.380539344801));
#29430=CARTESIAN_POINT('Ctrl Pts',(-41.8933446326271,37.4910552599798,38.3875446700045));
#29431=CARTESIAN_POINT('Ctrl Pts',(-41.9021026301559,37.5015806320539,38.394549995208));
#29432=CARTESIAN_POINT('Ctrl Pts',(-41.910827363451,37.5121574888643,38.4015195521993));
#29433=CARTESIAN_POINT('Ctrl Pts',(-41.9195184610102,37.5227853800447,38.4084530442122));
#29434=CARTESIAN_POINT('Ctrl Pts',(-41.9282095585694,37.5334132712252,38.415386536225));
#29435=CARTESIAN_POINT('Ctrl Pts',(-41.9368670208726,37.5440921976628,38.4222839640525));
#29436=CARTESIAN_POINT('Ctrl Pts',(-41.9454904783322,37.5548217028996,38.4291450324364));
#29437=CARTESIAN_POINT('Ctrl Pts',(-41.9541139357918,37.5655512081365,38.4360061008203));
#29438=CARTESIAN_POINT('Ctrl Pts',(-41.9627033888718,37.5763312930231,38.4428308105248));
#29439=CARTESIAN_POINT('Ctrl Pts',(-41.9712584718331,37.5871614985452,38.4496188709562));
#29440=CARTESIAN_POINT('Ctrl Pts',(-41.9798135547945,37.5979917040673,38.4564069313877));
#29441=CARTESIAN_POINT('Ctrl Pts',(-41.9883342676352,37.6088720302228,38.4631583425448));
#29442=CARTESIAN_POINT('Ctrl Pts',(-41.9968202475373,37.6198020137172,38.4698728169447));
#29443=CARTESIAN_POINT('Ctrl Pts',(-42.0053062274393,37.6307319972116,38.4765872913445));
#29444=CARTESIAN_POINT('Ctrl Pts',(-42.0137574744005,37.6417116380421,38.4832648289854));
#29445=CARTESIAN_POINT('Ctrl Pts',(-42.022173628567,37.6527404686982,38.4899051455408));
#29446=CARTESIAN_POINT('Ctrl Pts',(-42.0305897827335,37.6637692993541,38.4965454620962));
#29447=CARTESIAN_POINT('Ctrl Pts',(-42.0389708441033,37.6748473198335,38.5031485575649));
#29448=CARTESIAN_POINT('Ctrl Pts',(-42.0473164558045,37.6859740584228,38.5097141507787));
#29449=CARTESIAN_POINT('Ctrl Pts',(-42.0556620675058,37.6971007970122,38.5162797439925));
#29450=CARTESIAN_POINT('Ctrl Pts',(-42.063972229538,37.7082762537124,38.5228078349527));
#29451=CARTESIAN_POINT('Ctrl Pts',(-42.0722465880516,37.7194999526687,38.529298145691));
#29452=CARTESIAN_POINT('Ctrl Pts',(-42.0805209465652,37.7307236516249,38.5357884564294));
#29453=CARTESIAN_POINT('Ctrl Pts',(-42.0887595015562,37.7419955928303,38.5422409869407));
#29454=CARTESIAN_POINT('Ctrl Pts',(-42.0969619022279,37.7533152963297,38.5486554624809));
#29455=CARTESIAN_POINT('Ctrl Pts',(-42.105171592723,37.7646450601323,38.5550756388391));
#29456=CARTESIAN_POINT('Ctrl Pts',(-42.1133450638489,37.7760226695206,38.5614576912358));
#29457=CARTESIAN_POINT('Ctrl Pts',(-42.1214819684532,37.7874476424097,38.5678013500418));
#29458=CARTESIAN_POINT('Ctrl Pts',(-41.700042897706,37.278244944623,38.2403033155339));
#29459=CARTESIAN_POINT('Ctrl Pts',(-41.7096370309394,37.288476862104,38.2481683151151));
#29460=CARTESIAN_POINT('Ctrl Pts',(-41.7191977923432,37.2987682567707,38.2559966469369));
#29461=CARTESIAN_POINT('Ctrl Pts',(-41.7287247392384,37.309118652262,38.2637879487463));
#29462=CARTESIAN_POINT('Ctrl Pts',(-41.7382516861337,37.3194690477533,38.2715792505558));
#29463=CARTESIAN_POINT('Ctrl Pts',(-41.7477448185176,37.3298784440664,38.2793335223506));
#29464=CARTESIAN_POINT('Ctrl Pts',(-41.7572036968316,37.3403463593958,38.2870504052947));
#29465=CARTESIAN_POINT('Ctrl Pts',(-41.7666625751455,37.3508142747253,38.2947672882388));
#29466=CARTESIAN_POINT('Ctrl Pts',(-41.7760871993865,37.3613407090683,38.3024467823298));
#29467=CARTESIAN_POINT('Ctrl Pts',(-41.7854771331562,37.37192517522,38.3100885321811));
#29468=CARTESIAN_POINT('Ctrl Pts',(-41.7948670669259,37.3825096413715,38.3177302820325));
#29469=CARTESIAN_POINT('Ctrl Pts',(-41.8042223102216,37.3931521393287,38.3253342876419));
#29470=CARTESIAN_POINT('Ctrl Pts',(-41.8135424298451,37.4038521765317,38.332900197105));
#29471=CARTESIAN_POINT('Ctrl Pts',(-41.8228625494686,37.4145522137346,38.3404661065682));
#29472=CARTESIAN_POINT('Ctrl Pts',(-41.8321475454174,37.4253097901801,38.3479939198828));
#29473=CARTESIAN_POINT('Ctrl Pts',(-41.8413969877339,37.4361244079988,38.3554832886594));
#29474=CARTESIAN_POINT('Ctrl Pts',(-41.8506464300503,37.4469390258174,38.3629726574359));
#29475=CARTESIAN_POINT('Ctrl Pts',(-41.8598603187317,37.4578106850061,38.3704235816722));
#29476=CARTESIAN_POINT('Ctrl Pts',(-41.8690382271003,37.4687388824313,38.3778357165252));
#29477=CARTESIAN_POINT('Ctrl Pts',(-41.8782161354689,37.4796670798566,38.3852478513781));
#29478=CARTESIAN_POINT('Ctrl Pts',(-41.8873580635222,37.4906518155152,38.3926211968457));
#29479=CARTESIAN_POINT('Ctrl Pts',(-41.8964635879016,37.5016925810564,38.3999554116631));
#29480=CARTESIAN_POINT('Ctrl Pts',(-41.905569112281,37.5127333465975,38.4072896264807));
#29481=CARTESIAN_POINT('Ctrl Pts',(-41.9146382329839,37.5238301420179,38.4145847106461));
#29482=CARTESIAN_POINT('Ctrl Pts',(-41.92367053001,37.5349824537957,38.4218403265046));
#29483=CARTESIAN_POINT('Ctrl Pts',(-41.932702827036,37.5461347655735,38.4290959423631));
#29484=CARTESIAN_POINT('Ctrl Pts',(-41.9416983008208,37.5573425945316,38.4363120906505));
#29485=CARTESIAN_POINT('Ctrl Pts',(-41.9506565338972,37.5686054204039,38.4434884359012));
#29486=CARTESIAN_POINT('Ctrl Pts',(-41.9596147669736,37.5798682462761,38.450664781152));
#29487=CARTESIAN_POINT('Ctrl Pts',(-41.9685357597629,37.5911860698514,38.4578013240754));
#29488=CARTESIAN_POINT('Ctrl Pts',(-41.9774190990994,37.6025583674136,38.4648977343334));
#29489=CARTESIAN_POINT('Ctrl Pts',(-41.9863024384359,37.6139306649757,38.4719941445915));
#29490=CARTESIAN_POINT('Ctrl Pts',(-41.9951481243171,37.6253574365218,38.4790504221826));
#29491=CARTESIAN_POINT('Ctrl Pts',(-42.003955747045,37.636838153297,38.4860662404613));
#29492=CARTESIAN_POINT('Ctrl Pts',(-42.0127633697729,37.6483188700721,38.4930820587401));
#29493=CARTESIAN_POINT('Ctrl Pts',(-42.0215329293449,37.6598535320727,38.5000574177044));
#29494=CARTESIAN_POINT('Ctrl Pts',(-42.0302640195796,37.6714416055764,38.506991994451));
#29495=CARTESIAN_POINT('Ctrl Pts',(-42.0389951098142,37.6830296790801,38.5139265711977));
#29496=CARTESIAN_POINT('Ctrl Pts',(-42.0476877307091,37.6946711640841,38.5208203657249));
#29497=CARTESIAN_POINT('Ctrl Pts',(-42.056341479625,37.7063655219231,38.5276730588806));
#29498=CARTESIAN_POINT('Ctrl Pts',(-42.0649952285409,37.7180598797622,38.5345257520362));
#29499=CARTESIAN_POINT('Ctrl Pts',(-42.0736101054769,37.7298071104363,38.541337343821));
#29500=CARTESIAN_POINT('Ctrl Pts',(-42.0821857113822,37.7416066704065,38.5481075188797));
#29501=CARTESIAN_POINT('Ctrl Pts',(-42.0907613172874,37.7534062303768,38.5548776939382));
#29502=CARTESIAN_POINT('Ctrl Pts',(-42.0992976521577,37.7652581196358,38.5616064522654));
#29503=CARTESIAN_POINT('Ctrl Pts',(-42.1077943205678,37.7771617898219,38.568293482332));
#29504=CARTESIAN_POINT('Ctrl Pts',(-42.1162985403295,37.7890760393073,38.5749864554474));
#29505=CARTESIAN_POINT('Ctrl Pts',(-42.1247630224106,37.8010421602726,38.5816376248783));
#29506=CARTESIAN_POINT('Ctrl Pts',(-42.1331873753432,37.8130596011009,38.5882466845272));
#29507=CARTESIAN_POINT('Ctrl Pts',(-41.6954029970919,37.2787291081676,38.2453114933174));
#29508=CARTESIAN_POINT('Ctrl Pts',(-41.705374151905,37.2893988547556,38.2535435440881));
#29509=CARTESIAN_POINT('Ctrl Pts',(-41.7153090277789,37.3001332597734,38.2617357328736));
#29510=CARTESIAN_POINT('Ctrl Pts',(-41.7252071244471,37.3109317828591,38.269887647392));
#29511=CARTESIAN_POINT('Ctrl Pts',(-41.7351052211153,37.3217303059448,38.2780395619104));
#29512=CARTESIAN_POINT('Ctrl Pts',(-41.7449665385822,37.3325929471042,38.2861512021675));
#29513=CARTESIAN_POINT('Ctrl Pts',(-41.7547905802872,37.3435191595641,38.2942221599408));
#29514=CARTESIAN_POINT('Ctrl Pts',(-41.7646146219922,37.354445372024,38.302293117714));
#29515=CARTESIAN_POINT('Ctrl Pts',(-41.7744013879321,37.3654351557807,38.3103233930009));
#29516=CARTESIAN_POINT('Ctrl Pts',(-41.7841503852857,37.3764879576831,38.3183125816596));
#29517=CARTESIAN_POINT('Ctrl Pts',(-41.7938993826392,37.3875407595854,38.3263017703184));
#29518=CARTESIAN_POINT('Ctrl Pts',(-41.8036106114032,37.3986565796297,38.3342498723465));
#29519=CARTESIAN_POINT('Ctrl Pts',(-41.8132835825446,37.4098348583421,38.3421564877236));
#29520=CARTESIAN_POINT('Ctrl Pts',(-41.8229565536861,37.4210131370545,38.3500631031007));
#29521=CARTESIAN_POINT('Ctrl Pts',(-41.8325912672018,37.4322538744313,38.3579282318242));
#29522=CARTESIAN_POINT('Ctrl Pts',(-41.8421872378963,37.443556504732,38.365751478035));
#29523=CARTESIAN_POINT('Ctrl Pts',(-41.8517832085907,37.4548591350325,38.3735747242459));
#29524=CARTESIAN_POINT('Ctrl Pts',(-41.8613404364607,37.4662236582531,38.3813560879416));
#29525=CARTESIAN_POINT('Ctrl Pts',(-41.8708584401965,37.4776495024429,38.3890951774638));
#29526=CARTESIAN_POINT('Ctrl Pts',(-41.8803764439323,37.4890753466328,38.3968342669861));
#29527=CARTESIAN_POINT('Ctrl Pts',(-41.8898552235308,37.5005625117879,38.4045310823324));
#29528=CARTESIAN_POINT('Ctrl Pts',(-41.899294301616,37.5121104198047,38.4121852360844));
#29529=CARTESIAN_POINT('Ctrl Pts',(-41.9087333797013,37.5236583278214,38.4198393898364));
#29530=CARTESIAN_POINT('Ctrl Pts',(-41.9181327562374,37.5352669786346,38.4274508819364));
#29531=CARTESIAN_POINT('Ctrl Pts',(-41.9274919578949,37.5469357881649,38.4350193293532));
#29532=CARTESIAN_POINT('Ctrl Pts',(-41.9368511595524,37.5586045976952,38.4425877767701));
#29533=CARTESIAN_POINT('Ctrl Pts',(-41.9461701862917,37.570333565871,38.4501131794401));
#29534=CARTESIAN_POINT('Ctrl Pts',(-41.9554485687568,37.5821221024738,38.4575951585563));
#29535=CARTESIAN_POINT('Ctrl Pts',(-41.964726951222,37.5939106390765,38.4650771376724));
#29536=CARTESIAN_POINT('Ctrl Pts',(-41.9739646894053,37.6057587440936,38.4725156932246));
#29537=CARTESIAN_POINT('Ctrl Pts',(-41.9831613180177,37.6176658213109,38.4799104507449));
#29538=CARTESIAN_POINT('Ctrl Pts',(-41.9923579466302,37.6295728985282,38.4873052082651));
#29539=CARTESIAN_POINT('Ctrl Pts',(-42.0015134656686,37.6415389479416,38.494656167751));
#29540=CARTESIAN_POINT('Ctrl Pts',(-42.0106274139663,37.6535633674186,38.501962959127));
#29541=CARTESIAN_POINT('Ctrl Pts',(-42.019741362264,37.6655877868956,38.5092697505029));
#29542=CARTESIAN_POINT('Ctrl Pts',(-42.028813739818,37.6776705764321,38.5165323737665));
#29543=CARTESIAN_POINT('Ctrl Pts',(-42.0378440896301,37.6898111280371,38.5237504632711));
#29544=CARTESIAN_POINT('Ctrl Pts',(-42.0468744394422,37.7019516796421,38.5309685527758));
#29545=CARTESIAN_POINT('Ctrl Pts',(-42.0558627615093,37.7141499933116,38.5381421085192));
#29546=CARTESIAN_POINT('Ctrl Pts',(-42.0648086030478,37.726405455257,38.5452707693207));
#29547=CARTESIAN_POINT('Ctrl Pts',(-42.0737544445863,37.7386609172024,38.5523994301222));
#29548=CARTESIAN_POINT('Ctrl Pts',(-42.0826578055931,37.7509735274196,38.5594831959794));
#29549=CARTESIAN_POINT('Ctrl Pts',(-42.0915182375439,37.7633426663837,38.5665217102134));
#29550=CARTESIAN_POINT('Ctrl Pts',(-42.1003786694947,37.7757118053479,38.5735602244475));
#29551=CARTESIAN_POINT('Ctrl Pts',(-42.1091961723865,37.7881374730549,38.580553487056));
#29552=CARTESIAN_POINT('Ctrl Pts',(-42.1179703019997,37.8006190443054,38.5875011458977));
#29553=CARTESIAN_POINT('Ctrl Pts',(-42.126752229556,37.8131117084607,38.5944549794202));
#29554=CARTESIAN_POINT('Ctrl Pts',(-42.1354907067083,37.8256603755839,38.6013631280908));
#29555=CARTESIAN_POINT('Ctrl Pts',(-42.1441852923974,37.8382644131475,38.608225243387));
#29556=CARTESIAN_POINT('Ctrl Pts',(-41.6907493022857,37.2791971682105,38.2503061045895));
#29557=CARTESIAN_POINT('Ctrl Pts',(-41.7010860575057,37.2902935419084,38.2588974308395));
#29558=CARTESIAN_POINT('Ctrl Pts',(-41.7113835341543,37.3014599201502,38.2674455992172));
#29559=CARTESIAN_POINT('Ctrl Pts',(-41.7216411691384,37.3126956923255,38.2759501422807));
#29560=CARTESIAN_POINT('Ctrl Pts',(-41.7318988041226,37.3239314645008,38.2844546853442));
#29561=CARTESIAN_POINT('Ctrl Pts',(-41.7421165974454,37.3352366306143,38.2929156030983));
#29562=CARTESIAN_POINT('Ctrl Pts',(-41.7522939903866,37.3466105724872,38.3013324328907));
#29563=CARTESIAN_POINT('Ctrl Pts',(-41.7624713833279,37.35798451436,38.3097492626831));
#29564=CARTESIAN_POINT('Ctrl Pts',(-41.7726083758836,37.3694272319876,38.3181220045104));
#29565=CARTESIAN_POINT('Ctrl Pts',(-41.7827044137518,37.3809380996695,38.3264502005419));
#29566=CARTESIAN_POINT('Ctrl Pts',(-41.7928004516199,37.3924489673513,38.3347783965733));
#29567=CARTESIAN_POINT('Ctrl Pts',(-41.8028555347964,37.4040279850829,38.3430620468056));
#29568=CARTESIAN_POINT('Ctrl Pts',(-41.8128691134583,37.4156745197107,38.3513006982795));
#29569=CARTESIAN_POINT('Ctrl Pts',(-41.8228826921201,37.4273210543384,38.3595393497535));
#29570=CARTESIAN_POINT('Ctrl Pts',(-41.8328547662634,37.4390351058577,38.3677330024657));
#29571=CARTESIAN_POINT('Ctrl Pts',(-41.8427847906039,37.4508160337313,38.3758812083785));
#29572=CARTESIAN_POINT('Ctrl Pts',(-41.8527148149444,37.4625969616049,38.3840294142911));
#29573=CARTESIAN_POINT('Ctrl Pts',(-41.8626027894783,37.4744447658281,38.392132173401));
#29574=CARTESIAN_POINT('Ctrl Pts',(-41.8724481735202,37.4863587985498,38.4001890426401));
#29575=CARTESIAN_POINT('Ctrl Pts',(-41.8822935575621,37.4982728312715,38.4082459118793));
#29576=CARTESIAN_POINT('Ctrl Pts',(-41.892096351108,37.5102530924869,38.4162568912445));
#29577=CARTESIAN_POINT('Ctrl Pts',(-41.9018560181304,37.5222989271022,38.4242215426866));
#29578=CARTESIAN_POINT('Ctrl Pts',(-41.9116156851527,37.5343447617176,38.4321861941288));
#29579=CARTESIAN_POINT('Ctrl Pts',(-41.9213322256173,37.5464561696706,38.4401045175926));
#29580=CARTESIAN_POINT('Ctrl Pts',(-41.9310051082727,37.5586324888085,38.4479760801976));
#29581=CARTESIAN_POINT('Ctrl Pts',(-41.9406779909281,37.5708088079463,38.4558476428027));
#29582=CARTESIAN_POINT('Ctrl Pts',(-41.9503072157368,37.5830500382009,38.463672444488));
#29583=CARTESIAN_POINT('Ctrl Pts',(-41.9598922561705,37.5953555102244,38.4714500573998));
#29584=CARTESIAN_POINT('Ctrl Pts',(-41.9694772966042,37.6076609822479,38.4792276703115));
#29585=CARTESIAN_POINT('Ctrl Pts',(-41.9790181526549,37.6200306960276,38.4869580944392));
#29586=CARTESIAN_POINT('Ctrl Pts',(-41.9885143026182,37.6324639751736,38.4946409070749));
#29587=CARTESIAN_POINT('Ctrl Pts',(-41.9980104525814,37.6448972543196,38.5023237197104));
#29588=CARTESIAN_POINT('Ctrl Pts',(-42.0074618964534,37.6573940988272,38.5099589208508));
#29589=CARTESIAN_POINT('Ctrl Pts',(-42.0168681174187,37.6699538253549,38.5175460929948));
#29590=CARTESIAN_POINT('Ctrl Pts',(-42.026274338384,37.6825135518827,38.5251332651387));
#29591=CARTESIAN_POINT('Ctrl Pts',(-42.0356353364388,37.6951361604256,38.5326724082832));
#29592=CARTESIAN_POINT('Ctrl Pts',(-42.0449505997135,37.7078209607656,38.5401631101795));
#29593=CARTESIAN_POINT('Ctrl Pts',(-42.0542658629882,37.7205057611056,38.5476538120758));
#29594=CARTESIAN_POINT('Ctrl Pts',(-42.063535391479,37.7332527532376,38.555096072721));
#29595=CARTESIAN_POINT('Ctrl Pts',(-42.0727586783179,37.7460612401418,38.562489485164));
#29596=CARTESIAN_POINT('Ctrl Pts',(-42.0819819651568,37.7588697270461,38.569882897607));
#29597=CARTESIAN_POINT('Ctrl Pts',(-42.0911590103401,37.7717397087176,38.5772274618448));
#29598=CARTESIAN_POINT('Ctrl Pts',(-42.1002893120568,37.7846704814115,38.5845227762687));
#29599=CARTESIAN_POINT('Ctrl Pts',(-42.1094196137735,37.7976012541054,38.5918180906926));
#29600=CARTESIAN_POINT('Ctrl Pts',(-42.1185031720199,37.8105928178165,38.5990641552995));
#29601=CARTESIAN_POINT('Ctrl Pts',(-42.1275394900971,37.8236444621519,38.6062605738666));
#29602=CARTESIAN_POINT('Ctrl Pts',(-42.1365838391356,37.8367077060402,38.6134633881979));
#29603=CARTESIAN_POINT('Ctrl Pts',(-42.1455808640018,37.8498311374031,38.6206164682147));
#29604=CARTESIAN_POINT('Ctrl Pts',(-42.1545300718383,37.8630140373325,38.627719422056));
#29605=CARTESIAN_POINT('Ctrl Pts',(-41.6814419126733,37.2801332882965,38.2602953271335));
#29606=CARTESIAN_POINT('Ctrl Pts',(-41.692509868707,37.2920829162141,38.2696052043424));
#29607=CARTESIAN_POINT('Ctrl Pts',(-41.7035325469051,37.3041132409037,38.2788653319044));
#29608=CARTESIAN_POINT('Ctrl Pts',(-41.7145092585211,37.3162235112583,38.2880751320582));
#29609=CARTESIAN_POINT('Ctrl Pts',(-41.7254859701371,37.3283337816128,38.2972849322119));
#29610=CARTESIAN_POINT('Ctrl Pts',(-41.7364167151718,37.3405239976348,38.30644440496));
#29611=CARTESIAN_POINT('Ctrl Pts',(-41.7473008105857,37.3527933983334,38.3155529787907));
#29612=CARTESIAN_POINT('Ctrl Pts',(-41.7581849059995,37.3650627990321,38.3246615526213));
#29613=CARTESIAN_POINT('Ctrl Pts',(-41.7690223517866,37.3774113844015,38.3337192275295));
#29614=CARTESIAN_POINT('Ctrl Pts',(-41.7798124706839,37.3898383836423,38.3427254383063));
#29615=CARTESIAN_POINT('Ctrl Pts',(-41.7906025895811,37.4022653828832,38.3517316490831));
#29616=CARTESIAN_POINT('Ctrl Pts',(-41.8013453815828,37.4147707959893,38.3606863957238));
#29617=CARTESIAN_POINT('Ctrl Pts',(-41.8120401752855,37.4273538424477,38.3695891193914));
#29618=CARTESIAN_POINT('Ctrl Pts',(-41.8227349689883,37.4399368889061,38.378491843059));
#29619=CARTESIAN_POINT('Ctrl Pts',(-41.8333817643865,37.4525975687106,38.3873425437489));
#29620=CARTESIAN_POINT('Ctrl Pts',(-41.8439798960192,37.4653350917302,38.3961406690652));
#29621=CARTESIAN_POINT('Ctrl Pts',(-41.8545780276519,37.4780726147497,38.4049387943816));
#29622=CARTESIAN_POINT('Ctrl Pts',(-41.8651274955135,37.4908869809781,38.4136843443197));
#29623=CARTESIAN_POINT('Ctrl Pts',(-41.8756276401675,37.5037773907635,38.4223767729926));
#29624=CARTESIAN_POINT('Ctrl Pts',(-41.8861277848215,37.516667800549,38.4310692016655));
#29625=CARTESIAN_POINT('Ctrl Pts',(-41.8965786062624,37.529634253885,38.4397085090687));
#29626=CARTESIAN_POINT('Ctrl Pts',(-41.906979451159,37.5426759416976,38.448294155891));
#29627=CARTESIAN_POINT('Ctrl Pts',(-41.9173802960555,37.5557176295101,38.4568798027133));
#29628=CARTESIAN_POINT('Ctrl Pts',(-41.9277311643771,37.5688345517426,38.4654117889052));
#29629=CARTESIAN_POINT('Ctrl Pts',(-41.9380314090283,37.5820258900957,38.4738895818864));
#29630=CARTESIAN_POINT('Ctrl Pts',(-41.9483316536795,37.5952172284488,38.4823673748677));
#29631=CARTESIAN_POINT('Ctrl Pts',(-41.958581274627,37.6084829828606,38.4907909745839));
#29632=CARTESIAN_POINT('Ctrl Pts',(-41.9687796309978,37.6218223257258,38.4991598550868));
#29633=CARTESIAN_POINT('Ctrl Pts',(-41.9789779873686,37.6351616685908,38.5075287355896));
#29634=CARTESIAN_POINT('Ctrl Pts',(-41.9891250791542,37.6485745998954,38.5158428968686));
#29635=CARTESIAN_POINT('Ctrl Pts',(-41.9992202718191,37.6620602828989,38.5241018197348));
#29636=CARTESIAN_POINT('Ctrl Pts',(-42.0093154644839,37.6755459659026,38.532360742601));
#29637=CARTESIAN_POINT('Ctrl Pts',(-42.019358758023,37.6891044005982,38.5405644270504));
#29638=CARTESIAN_POINT('Ctrl Pts',(-42.0293495243234,37.7027347412276,38.5487123607303));
#29639=CARTESIAN_POINT('Ctrl Pts',(-42.0393402906239,37.7163650818568,38.5568602944103));
#29640=CARTESIAN_POINT('Ctrl Pts',(-42.0492785296805,37.7300673284127,38.5649524773167));
#29641=CARTESIAN_POINT('Ctrl Pts',(-42.0591636198804,37.7438406262226,38.5729884039963));
#29642=CARTESIAN_POINT('Ctrl Pts',(-42.0690487100803,37.7576139240325,38.5810243306759));
#29643=CARTESIAN_POINT('Ctrl Pts',(-42.0788806514184,37.7714582730893,38.5890040011246));
#29644=CARTESIAN_POINT('Ctrl Pts',(-42.0886588288581,37.7853728099114,38.5969269168506));
#29645=CARTESIAN_POINT('Ctrl Pts',(-42.0984370062978,37.7992873467335,38.6048498325766));
#29646=CARTESIAN_POINT('Ctrl Pts',(-42.1081614198342,37.8132720713135,38.6127159935759));
#29647=CARTESIAN_POINT('Ctrl Pts',(-42.1178314610826,37.8273261114669,38.6205249083793));
#29648=CARTESIAN_POINT('Ctrl Pts',(-42.127501502331,37.8413801516203,38.6283338231828));
#29649=CARTESIAN_POINT('Ctrl Pts',(-42.1371171712866,37.8555035073398,38.6360854917864));
#29650=CARTESIAN_POINT('Ctrl Pts',(-42.1466778662919,37.8696952978447,38.6437794298044));
#29651=CARTESIAN_POINT('Ctrl Pts',(-42.1562470582947,37.8838997011991,38.6514802057533));
#29652=CARTESIAN_POINT('Ctrl Pts',(-42.1657611785889,37.8981726610412,38.6591231484625));
#29653=CARTESIAN_POINT('Ctrl Pts',(-42.1752196307201,37.9125132857024,38.6667077793939));
#29654=CARTESIAN_POINT('Ctrl Pts',(-41.6720797281154,37.281005440121,38.2702306591526));
#29655=CARTESIAN_POINT('Ctrl Pts',(-41.6838331847125,37.2937633030351,38.2802276560053));
#29656=CARTESIAN_POINT('Ctrl Pts',(-41.6955349997854,37.3066132044251,38.2901679110195));
#29657=CARTESIAN_POINT('Ctrl Pts',(-41.707184337945,37.3195542276318,38.3000507155175));
#29658=CARTESIAN_POINT('Ctrl Pts',(-41.7188336761045,37.3324952508385,38.3099335200156));
#29659=CARTESIAN_POINT('Ctrl Pts',(-41.7304305373428,37.3455273958532,38.319758873991));
#29660=CARTESIAN_POINT('Ctrl Pts',(-41.7419740936924,37.3586497331262,38.3295260768912));
#29661=CARTESIAN_POINT('Ctrl Pts',(-41.753517650042,37.3717720703992,38.3392932797915));
#29662=CARTESIAN_POINT('Ctrl Pts',(-41.7650079014953,37.3849845999216,38.3490023316102));
#29663=CARTESIAN_POINT('Ctrl Pts',(-41.7764440276226,37.3982863793831,38.3586525400184));
#29664=CARTESIAN_POINT('Ctrl Pts',(-41.78788015375,37.4115881588446,38.3683027484267));
#29665=CARTESIAN_POINT('Ctrl Pts',(-41.7992621545438,37.4249791882362,38.377894113418));
#29666=CARTESIAN_POINT('Ctrl Pts',(-41.8105892172277,37.438458512619,38.387425950984));
#29667=CARTESIAN_POINT('Ctrl Pts',(-41.8219162799116,37.4519378370016,38.3969577885501));
#29668=CARTESIAN_POINT('Ctrl Pts',(-41.833188404478,37.4655054563663,38.4064300986844));
#29669=CARTESIAN_POINT('Ctrl Pts',(-41.8444047859174,37.479160403279,38.4158422057947));
#29670=CARTESIAN_POINT('Ctrl Pts',(-41.8556211673568,37.4928153501917,38.425254312905));
#29671=CARTESIAN_POINT('Ctrl Pts',(-41.8667818056617,37.5065576246432,38.4346062169849));
#29672=CARTESIAN_POINT('Ctrl Pts',(-41.8778859037026,37.5203862468399,38.4438972509529));
#29673=CARTESIAN_POINT('Ctrl Pts',(-41.8889900017434,37.5342148690365,38.4531882849209));
#29674=CARTESIAN_POINT('Ctrl Pts',(-41.9000375595128,37.5481298389691,38.4624184487706));
#29675=CARTESIAN_POINT('Ctrl Pts',(-41.9110277878729,37.5621301646213,38.4715870840247));
#29676=CARTESIAN_POINT('Ctrl Pts',(-41.9220180162329,37.5761304902734,38.4807557192787));
#29677=CARTESIAN_POINT('Ctrl Pts',(-41.9329509151763,37.5902161716359,38.489862825931));
#29678=CARTESIAN_POINT('Ctrl Pts',(-41.9438257036674,37.6043862046088,38.4989077542001));
#29679=CARTESIAN_POINT('Ctrl Pts',(-41.9547004921585,37.6185562375817,38.5079526824692));
#29680=CARTESIAN_POINT('Ctrl Pts',(-41.9655171701902,37.6328106221554,38.5169354323492));
#29681=CARTESIAN_POINT('Ctrl Pts',(-41.9762749649388,37.647148342287,38.5258553628462));
#29682=CARTESIAN_POINT('Ctrl Pts',(-41.9870327596873,37.6614860624186,38.5347752933432));
#29683=CARTESIAN_POINT('Ctrl Pts',(-41.9977316711457,37.6759071180982,38.5436324044513));
#29684=CARTESIAN_POINT('Ctrl Pts',(-42.0083709348107,37.6904104814819,38.5524260640536));
#29685=CARTESIAN_POINT('Ctrl Pts',(-42.0190101984756,37.7049138448655,38.561219723656));
#29686=CARTESIAN_POINT('Ctrl Pts',(-42.0295898143401,37.7194995159433,38.5699499317467));
#29687=CARTESIAN_POINT('Ctrl Pts',(-42.0401090263286,37.7341664552137,38.5786160651747));
#29688=CARTESIAN_POINT('Ctrl Pts',(-42.0506282383171,37.7488333944841,38.5872821986028));
#29689=CARTESIAN_POINT('Ctrl Pts',(-42.0610870464226,37.7635816019373,38.5958842573624));
#29690=CARTESIAN_POINT('Ctrl Pts',(-42.0714847031035,37.7784100265598,38.6044216273555));
#29691=CARTESIAN_POINT('Ctrl Pts',(-42.0818823597843,37.7932384511822,38.6129589973486));
#29692=CARTESIAN_POINT('Ctrl Pts',(-42.0922188650336,37.808147092964,38.6214316785695));
#29693=CARTESIAN_POINT('Ctrl Pts',(-42.1024934799483,37.8231348895265,38.6298390660592));
#29694=CARTESIAN_POINT('Ctrl Pts',(-42.1127680948631,37.838122686089,38.6382464535489));
#29695=CARTESIAN_POINT('Ctrl Pts',(-42.1229808194365,37.8531896374223,38.6465885473018));
#29696=CARTESIAN_POINT('Ctrl Pts',(-42.1331309235081,37.8683346699313,38.654864751583));
#29697=CARTESIAN_POINT('Ctrl Pts',(-42.1432810275798,37.8834797024403,38.6631409558641));
#29698=CARTESIAN_POINT('Ctrl Pts',(-42.1533685111429,37.898702816115,38.6713512706679));
#29699=CARTESIAN_POINT('Ctrl Pts',(-42.1633926528822,37.9140029262941,38.6794951095668));
#29700=CARTESIAN_POINT('Ctrl Pts',(-42.1734257035038,37.9293166343336,38.6876461862427));
#29701=CARTESIAN_POINT('Ctrl Pts',(-42.1833952996557,37.9447074757883,38.6957306687958));
#29702=CARTESIAN_POINT('Ctrl Pts',(-42.1933007270679,37.9601743521583,38.7037479786483));
#29703=CARTESIAN_POINT('Ctrl Pts',(-41.6626778025171,37.2818311977891,38.2801269060787));
#29704=CARTESIAN_POINT('Ctrl Pts',(-41.6750793521725,37.2953573955639,38.2907803473701));
#29705=CARTESIAN_POINT('Ctrl Pts',(-41.6874226859157,37.3089873490621,38.3013698231234));
#29706=CARTESIAN_POINT('Ctrl Pts',(-41.6997068034004,37.3227199536653,38.3118944751311));
#29707=CARTESIAN_POINT('Ctrl Pts',(-41.7119909208852,37.3364525582684,38.3224191271388));
#29708=CARTESIAN_POINT('Ctrl Pts',(-41.7242158221008,37.3502878139645,38.3328789553917));
#29709=CARTESIAN_POINT('Ctrl Pts',(-41.7363805162991,37.3642245994969,38.3432731121893));
#29710=CARTESIAN_POINT('Ctrl Pts',(-41.7485452104974,37.3781613850294,38.353667268987));
#29711=CARTESIAN_POINT('Ctrl Pts',(-41.7606496976679,37.3921997003858,38.3639957543202));
#29712=CARTESIAN_POINT('Ctrl Pts',(-41.7726929968212,37.406338407853,38.3742577311332));
#29713=CARTESIAN_POINT('Ctrl Pts',(-41.7847362959746,37.4204771153202,38.3845197079461));
#29714=CARTESIAN_POINT('Ctrl Pts',(-41.7967184071002,37.4347162148858,38.3947151762297));
#29715=CARTESIAN_POINT('Ctrl Pts',(-41.8086383591267,37.4490545525641,38.4048433097082));
#29716=CARTESIAN_POINT('Ctrl Pts',(-41.8205583111532,37.4633928902424,38.4149714431867));
#29717=CARTESIAN_POINT('Ctrl Pts',(-41.8324161040701,37.4778304660209,38.4250322418513));
#29718=CARTESIAN_POINT('Ctrl Pts',(-41.844210776881,37.4923661098289,38.43502489034));
#29719=CARTESIAN_POINT('Ctrl Pts',(-41.856005449692,37.5069017536367,38.4450175388289));
#29720=CARTESIAN_POINT('Ctrl Pts',(-41.8677370023867,37.5215354654614,38.4549420371332));
#29721=CARTESIAN_POINT('Ctrl Pts',(-41.8794044841998,37.5362660593363,38.4647975809376));
#29722=CARTESIAN_POINT('Ctrl Pts',(-41.8910719660129,37.5509966532113,38.474653124742));
#29723=CARTESIAN_POINT('Ctrl Pts',(-41.9026753769342,37.5658241291238,38.4844397140379));
#29724=CARTESIAN_POINT('Ctrl Pts',(-41.9142137765834,37.580747285404,38.4941565556864));
#29725=CARTESIAN_POINT('Ctrl Pts',(-41.9257521762325,37.5956704416843,38.5038733973348));
#29726=CARTESIAN_POINT('Ctrl Pts',(-41.9372255645993,37.6106892783193,38.5135204913274));
#29727=CARTESIAN_POINT('Ctrl Pts',(-41.9486330118411,37.6258025781309,38.5230970558303));
#29728=CARTESIAN_POINT('Ctrl Pts',(-41.9600404590829,37.6409158779426,38.5326736203333));
#29729=CARTESIAN_POINT('Ctrl Pts',(-41.9713819651896,37.6561236409176,38.5421796553383));
#29730=CARTESIAN_POINT('Ctrl Pts',(-41.9826566110065,37.6714246345665,38.5516143904435));
#29731=CARTESIAN_POINT('Ctrl Pts',(-41.9939312568235,37.6867256282154,38.5610491255488));
#29732=CARTESIAN_POINT('Ctrl Pts',(-42.0051390423408,37.702119852525,38.570412560746));
#29733=CARTESIAN_POINT('Ctrl Pts',(-42.016279059241,37.7176060598942,38.5797039371903));
#29734=CARTESIAN_POINT('Ctrl Pts',(-42.0274190761412,37.7330922672635,38.5889953136346));
#29735=CARTESIAN_POINT('Ctrl Pts',(-42.0384913244147,37.7486704576788,38.5982146313178));
#29736=CARTESIAN_POINT('Ctrl Pts',(-42.0494949067281,37.7643393686301,38.6073611430746));
#29737=CARTESIAN_POINT('Ctrl Pts',(-42.0604984890416,37.7800082795815,38.6165076548315));
#29738=CARTESIAN_POINT('Ctrl Pts',(-42.0714334053855,37.7957679110552,38.625581360654));
#29739=CARTESIAN_POINT('Ctrl Pts',(-42.0822987695567,37.8116169858364,38.6345815251779));
#29740=CARTESIAN_POINT('Ctrl Pts',(-42.0931641337279,37.8274660606176,38.6435816897018));
#29741=CARTESIAN_POINT('Ctrl Pts',(-42.1039599457167,37.8434045786925,38.6525083129191));
#29742=CARTESIAN_POINT('Ctrl Pts',(-42.1146853305936,37.8594312483488,38.6613606713857));
#29743=CARTESIAN_POINT('Ctrl Pts',(-42.1254107154704,37.8754579180051,38.6702130298523));
#29744=CARTESIAN_POINT('Ctrl Pts',(-42.1360656732259,37.8915727392288,38.6789911235603));
#29745=CARTESIAN_POINT('Ctrl Pts',(-42.1466493403455,37.9077744060193,38.6876942411029));
#29746=CARTESIAN_POINT('Ctrl Pts',(-42.1572330074652,37.9239760728097,38.6963973586456));
#29747=CARTESIAN_POINT('Ctrl Pts',(-42.1677453839397,37.9402645851528,38.7050255000152));
#29748=CARTESIAN_POINT('Ctrl Pts',(-42.17818561781,37.9566386229715,38.7135779659575));
#29749=CARTESIAN_POINT('Ctrl Pts',(-42.1886351303615,37.973027213096,38.7221380328411));
#29750=CARTESIAN_POINT('Ctrl Pts',(-42.1990123720102,37.9895014807696,38.7306222897181));
#29751=CARTESIAN_POINT('Ctrl Pts',(-42.209316500248,38.0060600884928,38.7390300477671));
#29752=CARTESIAN_POINT('Ctrl Pts',(-41.6532758769187,37.2826569554572,38.2900231530048));
#29753=CARTESIAN_POINT('Ctrl Pts',(-41.6663255196325,37.2969514880927,38.3013330387349));
#29754=CARTESIAN_POINT('Ctrl Pts',(-41.6793103720459,37.3113614936992,38.3125717352273));
#29755=CARTESIAN_POINT('Ctrl Pts',(-41.6922292688559,37.3258856796987,38.3237382347446));
#29756=CARTESIAN_POINT('Ctrl Pts',(-41.7051481656659,37.3404098656984,38.3349047342619));
#29757=CARTESIAN_POINT('Ctrl Pts',(-41.7180011068587,37.3550482320758,38.3459990367924));
#29758=CARTESIAN_POINT('Ctrl Pts',(-41.7307869389058,37.3697994658677,38.3570201474874));
#29759=CARTESIAN_POINT('Ctrl Pts',(-41.7435727709529,37.3845506996595,38.3680412581824));
#29760=CARTESIAN_POINT('Ctrl Pts',(-41.7562914938406,37.39941480085,38.3789891770303));
#29761=CARTESIAN_POINT('Ctrl Pts',(-41.7689419660199,37.4143904363229,38.3898629222479));
#29762=CARTESIAN_POINT('Ctrl Pts',(-41.7815924381992,37.4293660717959,38.4007366674656));
#29763=CARTESIAN_POINT('Ctrl Pts',(-41.7941746596566,37.4444532415353,38.4115362390414));
#29764=CARTESIAN_POINT('Ctrl Pts',(-41.8066875010257,37.4596505925093,38.4222606684324));
#29765=CARTESIAN_POINT('Ctrl Pts',(-41.8192003423948,37.4748479434832,38.4329850978234));
#29766=CARTESIAN_POINT('Ctrl Pts',(-41.8316438036622,37.4901554756755,38.4436343850181));
#29767=CARTESIAN_POINT('Ctrl Pts',(-41.8440167678447,37.5055718163786,38.4542075748854));
#29768=CARTESIAN_POINT('Ctrl Pts',(-41.8563897320273,37.5209881570818,38.4647807647527));
#29769=CARTESIAN_POINT('Ctrl Pts',(-41.8686921991118,37.5365133062795,38.4752778572815));
#29770=CARTESIAN_POINT('Ctrl Pts',(-41.8809230646971,37.5521458718328,38.4856979109224));
#29771=CARTESIAN_POINT('Ctrl Pts',(-41.8931539302824,37.5677784373861,38.4961179645632));
#29772=CARTESIAN_POINT('Ctrl Pts',(-41.9053131943556,37.5835184192784,38.5064609793052));
#29773=CARTESIAN_POINT('Ctrl Pts',(-41.9173997652938,37.5993644061868,38.516726027348));
#29774=CARTESIAN_POINT('Ctrl Pts',(-41.929486336232,37.6152103930952,38.5269910753909));
#29775=CARTESIAN_POINT('Ctrl Pts',(-41.9415002140224,37.6311623850027,38.5371781567238));
#29776=CARTESIAN_POINT('Ctrl Pts',(-41.9534403200148,37.6472189516531,38.5472863574605));
#29777=CARTESIAN_POINT('Ctrl Pts',(-41.9653804260072,37.6632755183035,38.5573945581973));
#29778=CARTESIAN_POINT('Ctrl Pts',(-41.9772467601889,37.6794366596797,38.5674238783273));
#29779=CARTESIAN_POINT('Ctrl Pts',(-41.9890382570742,37.695700926846,38.5773734180408));
#29780=CARTESIAN_POINT('Ctrl Pts',(-42.0008297539595,37.7119651940124,38.5873229577543));
#29781=CARTESIAN_POINT('Ctrl Pts',(-42.0125464135358,37.7283325869518,38.5971927170407));
#29782=CARTESIAN_POINT('Ctrl Pts',(-42.0241871836713,37.7448016383066,38.606981810327));
#29783=CARTESIAN_POINT('Ctrl Pts',(-42.0358279538069,37.7612706896614,38.6167709036133));
#29784=CARTESIAN_POINT('Ctrl Pts',(-42.0473928344892,37.7778413994143,38.6264793308889));
#29785=CARTESIAN_POINT('Ctrl Pts',(-42.0588807871277,37.7945122820466,38.6361062209745));
#29786=CARTESIAN_POINT('Ctrl Pts',(-42.0703687397661,37.8111831646789,38.6457331110602));
#29787=CARTESIAN_POINT('Ctrl Pts',(-42.0817797643485,37.827954220173,38.6552784639456));
#29788=CARTESIAN_POINT('Ctrl Pts',(-42.0931128360099,37.844823945113,38.6647414230003));
#29789=CARTESIAN_POINT('Ctrl Pts',(-42.1044459076713,37.8616936700531,38.6742043820549));
#29790=CARTESIAN_POINT('Ctrl Pts',(-42.1157010263998,37.8786620644211,38.6835849472687));
#29791=CARTESIAN_POINT('Ctrl Pts',(-42.1268771812388,37.8957276071712,38.6928822767122));
#29792=CARTESIAN_POINT('Ctrl Pts',(-42.1380533360778,37.9127931499213,38.7021796061556));
#29793=CARTESIAN_POINT('Ctrl Pts',(-42.1491505270153,37.9299558410353,38.7113936998188));
#29794=CARTESIAN_POINT('Ctrl Pts',(-42.1601677571829,37.9472141421073,38.7205237306229));
#29795=CARTESIAN_POINT('Ctrl Pts',(-42.1711849873505,37.9644724431792,38.729653761427));
#29796=CARTESIAN_POINT('Ctrl Pts',(-42.1821222567365,37.9818263541906,38.7386997293624));
#29797=CARTESIAN_POINT('Ctrl Pts',(-42.1929785827378,37.9992743196491,38.7476608223481));
#29798=CARTESIAN_POINT('Ctrl Pts',(-42.2038445572192,38.0167377918585,38.7566298794394));
#29799=CARTESIAN_POINT('Ctrl Pts',(-42.2146294443647,38.034295485751,38.7655139106404));
#29800=CARTESIAN_POINT('Ctrl Pts',(-42.2253322734281,38.0519458248273,38.7743121168858));
#29801=CARTESIAN_POINT('Ctrl Pts',(-41.6438340612598,37.2834361450012,38.2998801682775));
#29802=CARTESIAN_POINT('Ctrl Pts',(-41.6574945992981,37.2984594669515,38.3118162074907));
#29803=CARTESIAN_POINT('Ctrl Pts',(-41.6710835592186,37.3136103595045,38.3236735992583));
#29804=CARTESIAN_POINT('Ctrl Pts',(-41.6845995924923,37.3288873197827,38.3354511677636));
#29805=CARTESIAN_POINT('Ctrl Pts',(-41.6981156257661,37.3441642800609,38.3472287362689));
#29806=CARTESIAN_POINT('Ctrl Pts',(-41.7115587323755,37.3595673080445,38.3589264814965));
#29807=CARTESIAN_POINT('Ctrl Pts',(-41.7249275781878,37.3750948759654,38.3705432433879));
#29808=CARTESIAN_POINT('Ctrl Pts',(-41.738296424,37.3906224438864,38.3821600052791));
#29809=CARTESIAN_POINT('Ctrl Pts',(-41.7515910089977,37.4062745517245,38.3936957838189));
#29810=CARTESIAN_POINT('Ctrl Pts',(-41.7648100137066,37.4220496471208,38.405149434934));
#29811=CARTESIAN_POINT('Ctrl Pts',(-41.7780290184155,37.4378247425171,38.416603086049));
#29812=CARTESIAN_POINT('Ctrl Pts',(-41.7911724428184,37.4537228254511,38.4279746097245));
#29813=CARTESIAN_POINT('Ctrl Pts',(-41.8042389823588,37.4697423192777,38.4392628780974));
#29814=CARTESIAN_POINT('Ctrl Pts',(-41.8173055218992,37.4857618131042,38.4505511464703));
#29815=CARTESIAN_POINT('Ctrl Pts',(-41.83029517656,37.5019027178025,38.461756159526));
#29816=CARTESIAN_POINT('Ctrl Pts',(-41.8432066569589,37.5181634327507,38.472876805833));
#29817=CARTESIAN_POINT('Ctrl Pts',(-41.8561181373577,37.5344241476989,38.48399745214));
#29818=CARTESIAN_POINT('Ctrl Pts',(-41.8689514434778,37.5508046728759,38.4950337316839));
#29819=CARTESIAN_POINT('Ctrl Pts',(-41.8817053013641,37.5673033839973,38.5059845496832));
#29820=CARTESIAN_POINT('Ctrl Pts',(-41.8944591592503,37.5838020951187,38.5169353676825));
#29821=CARTESIAN_POINT('Ctrl Pts',(-41.9071335688862,37.6004189921631,38.5278007241229));
#29822=CARTESIAN_POINT('Ctrl Pts',(-41.9197272719944,37.6171524275023,38.5385795410877));
#29823=CARTESIAN_POINT('Ctrl Pts',(-41.9323209751025,37.6338858628415,38.5493583580525));
#29824=CARTESIAN_POINT('Ctrl Pts',(-41.9448339716667,37.6507358364539,38.5600506355277));
#29825=CARTESIAN_POINT('Ctrl Pts',(-41.9572650193348,37.6677006776908,38.5706553126729));
#29826=CARTESIAN_POINT('Ctrl Pts',(-41.9696960670028,37.6846655189277,38.5812599898182));
#29827=CARTESIAN_POINT('Ctrl Pts',(-41.982045165719,37.7017452276741,38.591777066537));
#29828=CARTESIAN_POINT('Ctrl Pts',(-41.9943110893787,37.7189381107715,38.6022054994369));
#29829=CARTESIAN_POINT('Ctrl Pts',(-42.0065770130384,37.7361309938689,38.6126339323367));
#29830=CARTESIAN_POINT('Ctrl Pts',(-42.018759761582,37.7534370511925,38.6229737213125));
#29831=CARTESIAN_POINT('Ctrl Pts',(-42.030858125247,37.7708545670661,38.6332238403209));
#29832=CARTESIAN_POINT('Ctrl Pts',(-42.0429564889119,37.7882720829396,38.6434739593292));
#29833=CARTESIAN_POINT('Ctrl Pts',(-42.0549704676829,37.8058010573424,38.6536344083581));
#29834=CARTESIAN_POINT('Ctrl Pts',(-42.0668988684252,37.8234397525212,38.6637041790089));
#29835=CARTESIAN_POINT('Ctrl Pts',(-42.0788272691675,37.8410784477,38.6737739496597));
#29836=CARTESIAN_POINT('Ctrl Pts',(-42.0906700918649,37.8588268636301,38.6837530419181));
#29837=CARTESIAN_POINT('Ctrl Pts',(-42.1024261602874,37.8766832409345,38.6936404653252));
#29838=CARTESIAN_POINT('Ctrl Pts',(-42.11418222871,37.8945396182387,38.7035278887324));
#29839=CARTESIAN_POINT('Ctrl Pts',(-42.1258515428427,37.9125039568964,38.7133236432767));
#29840=CARTESIAN_POINT('Ctrl Pts',(-42.1374329435463,37.9305744761275,38.7230267565294));
#29841=CARTESIAN_POINT('Ctrl Pts',(-42.1490143442499,37.9486449953587,38.7327298697821));
#29842=CARTESIAN_POINT('Ctrl Pts',(-42.1605078315089,37.9668216951379,38.7423403417292));
#29843=CARTESIAN_POINT('Ctrl Pts',(-42.1719122635506,37.9851027737687,38.751857218275));
#29844=CARTESIAN_POINT('Ctrl Pts',(-42.1833166955923,38.0033838523996,38.7613740948208));
#29845=CARTESIAN_POINT('Ctrl Pts',(-42.1946320723956,38.0217693098399,38.7707973759381));
#29846=CARTESIAN_POINT('Ctrl Pts',(-42.2058572697418,38.0402573237214,38.7801261259639));
#29847=CARTESIAN_POINT('Ctrl Pts',(-42.2170924433998,38.0587617686893,38.7894631668478));
#29848=CARTESIAN_POINT('Ctrl Pts',(-42.2282372772824,38.0773689526413,38.7987055086735));
#29849=CARTESIAN_POINT('Ctrl Pts',(-42.2392906618862,38.0960770276315,38.8078522316841));
#29850=CARTESIAN_POINT('Ctrl Pts',(-41.6343622916671,37.2841803659718,38.3097077240225));
#29851=CARTESIAN_POINT('Ctrl Pts',(-41.6486044484638,37.2998999854371,38.3222438581765));
#29852=CARTESIAN_POINT('Ctrl Pts',(-41.6627681091417,37.3157595051562,38.334693743636));
#29853=CARTESIAN_POINT('Ctrl Pts',(-41.6768517259748,37.3317571920888,38.3470560199468));
#29854=CARTESIAN_POINT('Ctrl Pts',(-41.690935342808,37.3477548790215,38.3594182962576));
#29855=CARTESIAN_POINT('Ctrl Pts',(-41.7049389157739,37.3638907331423,38.3716929633999));
#29856=CARTESIAN_POINT('Ctrl Pts',(-41.7188609146401,37.3801629912147,38.3838786800665));
#29857=CARTESIAN_POINT('Ctrl Pts',(-41.7327829135062,37.3964352492871,38.396064396733));
#29858=CARTESIAN_POINT('Ctrl Pts',(-41.7466233382503,37.4128439112853,38.4081611629044));
#29859=CARTESIAN_POINT('Ctrl Pts',(-41.7603806764678,37.429387184162,38.4201676567132));
#29860=CARTESIAN_POINT('Ctrl Pts',(-41.7741380146853,37.4459304570387,38.4321741505219));
#29861=CARTESIAN_POINT('Ctrl Pts',(-41.7878122663543,37.4626083407673,38.4440903719491));
#29862=CARTESIAN_POINT('Ctrl Pts',(-41.8014019372285,37.4794190128817,38.4559150188561));
#29863=CARTESIAN_POINT('Ctrl Pts',(-41.8149916081027,37.4962296849961,38.4677396657631));
#29864=CARTESIAN_POINT('Ctrl Pts',(-41.8284966981604,37.5131731454694,38.4794727381312));
#29865=CARTESIAN_POINT('Ctrl Pts',(-41.8419157316407,37.5302475428145,38.4911129538354));
#29866=CARTESIAN_POINT('Ctrl Pts',(-41.855334765121,37.5473219401595,38.5027531695397));
#29867=CARTESIAN_POINT('Ctrl Pts',(-41.8686677420024,37.5645272743491,38.5143005285616));
#29868=CARTESIAN_POINT('Ctrl Pts',(-41.8819132053312,37.58186166528,38.5257537690699));
#29869=CARTESIAN_POINT('Ctrl Pts',(-41.8951586686601,37.5991960562109,38.5372070095782));
#29870=CARTESIAN_POINT('Ctrl Pts',(-41.9083166184154,37.6166595038555,38.5485661315547));
#29871=CARTESIAN_POINT('Ctrl Pts',(-41.9213856167695,37.6342500999053,38.5598298937377));
#29872=CARTESIAN_POINT('Ctrl Pts',(-41.9344546151236,37.6518406959551,38.5710936559207));
#29873=CARTESIAN_POINT('Ctrl Pts',(-41.9474346620557,37.6695584403821,38.5822620582923));
#29874=CARTESIAN_POINT('Ctrl Pts',(-41.9603243391784,37.6874013970898,38.5933338804314));
#29875=CARTESIAN_POINT('Ctrl Pts',(-41.9732140163012,37.7052443537974,38.6044057025707));
#29876=CARTESIAN_POINT('Ctrl Pts',(-41.9860133235591,37.7232125226721,38.6153809443842));
#29877=CARTESIAN_POINT('Ctrl Pts',(-41.9987208623842,37.7413039404193,38.6262584067077));
#29878=CARTESIAN_POINT('Ctrl Pts',(-42.0114284012094,37.7593953581666,38.6371358690313));
#29879=CARTESIAN_POINT('Ctrl Pts',(-42.0240441715429,37.777610024664,38.6479155517638));
#29880=CARTESIAN_POINT('Ctrl Pts',(-42.0365667948123,37.7959459495368,38.658596276982));
#29881=CARTESIAN_POINT('Ctrl Pts',(-42.0490894180816,37.8142818744097,38.6692770022));
#29882=CARTESIAN_POINT('Ctrl Pts',(-42.0615188942673,37.8327390576306,38.6798587698879));
#29883=CARTESIAN_POINT('Ctrl Pts',(-42.0738538651359,37.8513154822757,38.6903404237066));
#29884=CARTESIAN_POINT('Ctrl Pts',(-42.0861888360046,37.8698919069209,38.7008220775252));
#29885=CARTESIAN_POINT('Ctrl Pts',(-42.0984293015361,37.8885875729586,38.7112036174569));
#29886=CARTESIAN_POINT('Ctrl Pts',(-42.1105739241704,37.9074004374591,38.7214839090885));
#29887=CARTESIAN_POINT('Ctrl Pts',(-42.1227185468047,37.9262133019595,38.7317642007201));
#29888=CARTESIAN_POINT('Ctrl Pts',(-42.1347673265229,37.9451433648946,38.7419432440364));
#29889=CARTESIAN_POINT('Ctrl Pts',(-42.1467189466908,37.964188557661,38.7520199267026));
#29890=CARTESIAN_POINT('Ctrl Pts',(-42.1586705668587,37.9832337504274,38.7620966093687));
#29891=CARTESIAN_POINT('Ctrl Pts',(-42.1705250274568,38.0023940729928,38.7720709313674));
#29892=CARTESIAN_POINT('Ctrl Pts',(-42.1822810331068,38.0216674316579,38.7819418027877));
#29893=CARTESIAN_POINT('Ctrl Pts',(-42.1940370387568,38.0409407903231,38.791812674208));
#29894=CARTESIAN_POINT('Ctrl Pts',(-42.2056945894344,38.0603271850404,38.8015800950206));
#29895=CARTESIAN_POINT('Ctrl Pts',(-42.2172524112672,38.0798244973725,38.811242997896));
#29896=CARTESIAN_POINT('Ctrl Pts',(-42.2288205050293,38.0993391377976,38.8209144886053));
#29897=CARTESIAN_POINT('Ctrl Pts',(-42.2402886926352,38.1189648932256,38.8304812756349));
#29898=CARTESIAN_POINT('Ctrl Pts',(-42.2516557185626,38.1386996149097,38.8399423114431));
#29899=CARTESIAN_POINT('Ctrl Pts',(-41.6248905220744,37.2849245869424,38.3195352797675));
#29900=CARTESIAN_POINT('Ctrl Pts',(-41.6397142976295,37.3013405039226,38.3326715088623));
#29901=CARTESIAN_POINT('Ctrl Pts',(-41.6544526590647,37.3179086508079,38.3457138880137));
#29902=CARTESIAN_POINT('Ctrl Pts',(-41.6691038594573,37.334627064395,38.3586608721299));
#29903=CARTESIAN_POINT('Ctrl Pts',(-41.6837550598498,37.3513454779822,38.3716078562462));
#29904=CARTESIAN_POINT('Ctrl Pts',(-41.6983190991723,37.36821415824,38.3844594453032));
#29905=CARTESIAN_POINT('Ctrl Pts',(-41.7127942510923,37.385231106464,38.397214116745));
#29906=CARTESIAN_POINT('Ctrl Pts',(-41.7272694030124,37.4022480546879,38.4099687881869));
#29907=CARTESIAN_POINT('Ctrl Pts',(-41.741655667503,37.4194132708462,38.4226265419898));
#29908=CARTESIAN_POINT('Ctrl Pts',(-41.755951339229,37.4367247212032,38.4351858784923));
#29909=CARTESIAN_POINT('Ctrl Pts',(-41.7702470109551,37.4540361715602,38.4477452149948));
#29910=CARTESIAN_POINT('Ctrl Pts',(-41.7844520898901,37.4714938560836,38.4602061341736));
#29911=CARTESIAN_POINT('Ctrl Pts',(-41.7985648920981,37.4890957064858,38.4725671596147));
#29912=CARTESIAN_POINT('Ctrl Pts',(-41.8126776943061,37.5066975568881,38.4849281850559));
#29913=CARTESIAN_POINT('Ctrl Pts',(-41.8266982197609,37.5244435731363,38.4971893167365));
#29914=CARTESIAN_POINT('Ctrl Pts',(-41.8406248063226,37.5423316528782,38.509349101838));
#29915=CARTESIAN_POINT('Ctrl Pts',(-41.8545513928842,37.5602197326201,38.5215088869395));
#29916=CARTESIAN_POINT('Ctrl Pts',(-41.8683840405269,37.5782498758223,38.5335673254393));
#29917=CARTESIAN_POINT('Ctrl Pts',(-41.8821211092983,37.5964199465627,38.5455229884566));
#29918=CARTESIAN_POINT('Ctrl Pts',(-41.8958581780698,37.6145900173031,38.5574786514739));
#29919=CARTESIAN_POINT('Ctrl Pts',(-41.9094996679445,37.6329000155479,38.5693315389865));
#29920=CARTESIAN_POINT('Ctrl Pts',(-41.9230439615446,37.6513477723083,38.5810802463877));
#29921=CARTESIAN_POINT('Ctrl Pts',(-41.9365882551445,37.6697955290687,38.5928289537889));
#29922=CARTESIAN_POINT('Ctrl Pts',(-41.9500353524446,37.6883810443104,38.6044734810568));
#29923=CARTESIAN_POINT('Ctrl Pts',(-41.9633836590221,37.7071021164888,38.61601244819));
#29924=CARTESIAN_POINT('Ctrl Pts',(-41.9767319655996,37.7258231886672,38.6275514153232));
#29925=CARTESIAN_POINT('Ctrl Pts',(-41.9899814813991,37.74467981767,38.6389848222313));
#29926=CARTESIAN_POINT('Ctrl Pts',(-42.0031306353897,37.7636697700671,38.6503113139786));
#29927=CARTESIAN_POINT('Ctrl Pts',(-42.0162797893803,37.7826597224643,38.6616378057259));
#29928=CARTESIAN_POINT('Ctrl Pts',(-42.0293285815038,37.8017829981353,38.6728573822152));
#29929=CARTESIAN_POINT('Ctrl Pts',(-42.0422754643776,37.8210373320075,38.683968713643));
#29930=CARTESIAN_POINT('Ctrl Pts',(-42.0552223472514,37.8402916658797,38.6950800450709));
#29931=CARTESIAN_POINT('Ctrl Pts',(-42.0680673208517,37.8596770579189,38.7060831314177));
#29932=CARTESIAN_POINT('Ctrl Pts',(-42.0808088618467,37.8791912120302,38.7169766684042));
#29933=CARTESIAN_POINT('Ctrl Pts',(-42.0935504028417,37.8987053661416,38.7278702053908));
#29934=CARTESIAN_POINT('Ctrl Pts',(-42.1061885112073,37.9183482822871,38.7386541929957));
#29935=CARTESIAN_POINT('Ctrl Pts',(-42.1187216880534,37.9381176339837,38.7493273528518));
#29936=CARTESIAN_POINT('Ctrl Pts',(-42.1312548648995,37.9578869856802,38.7600005127078));
#29937=CARTESIAN_POINT('Ctrl Pts',(-42.1436831102031,37.9777827728929,38.7705628447961));
#29938=CARTESIAN_POINT('Ctrl Pts',(-42.1560049498353,37.9978026391945,38.7810130968757));
#29939=CARTESIAN_POINT('Ctrl Pts',(-42.1683267894674,38.0178225054961,38.7914633489553));
#29940=CARTESIAN_POINT('Ctrl Pts',(-42.1805422234048,38.0379664508477,38.8018015210056));
#29941=CARTESIAN_POINT('Ctrl Pts',(-42.192649802663,38.0582320895472,38.8120263873004));
#29942=CARTESIAN_POINT('Ctrl Pts',(-42.2047573819213,38.0784977282466,38.8222512535952));
#29943=CARTESIAN_POINT('Ctrl Pts',(-42.2167571064732,38.0988850602409,38.832362814103));
#29944=CARTESIAN_POINT('Ctrl Pts',(-42.2286475527926,38.1193916710235,38.842359869828));
#29945=CARTESIAN_POINT('Ctrl Pts',(-42.2405485666589,38.1399165069059,38.8523658103628));
#29946=CARTESIAN_POINT('Ctrl Pts',(-42.2523401079879,38.1605608338099,38.8622570425963));
#29947=CARTESIAN_POINT('Ctrl Pts',(-42.264020775239,38.1813222021877,38.8720323912022));
#29948=CARTESIAN_POINT('Ctrl Pts',(-41.6153886967966,37.285633720554,38.3293332759128));
#29949=CARTESIAN_POINT('Ctrl Pts',(-41.6307648261287,37.3027135135746,38.3430436449347));
#29950=CARTESIAN_POINT('Ctrl Pts',(-41.6460484915149,37.3199581010959,38.3566524179197));
#29951=CARTESIAN_POINT('Ctrl Pts',(-41.6612377308598,37.3373652698898,38.3701578485853));
#29952=CARTESIAN_POINT('Ctrl Pts',(-41.6764269702048,37.3547724386838,38.3836632792508));
#29953=CARTESIAN_POINT('Ctrl Pts',(-41.6915217834752,37.3723421887124,38.3970653675675));
#29954=CARTESIAN_POINT('Ctrl Pts',(-41.7065202327379,37.3900722651408,38.4103623936964));
#29955=CARTESIAN_POINT('Ctrl Pts',(-41.7215186820006,37.4078023415691,38.4236594198254));
#29956=CARTESIAN_POINT('Ctrl Pts',(-41.7364207672228,37.4256927443586,38.4368513837376));
#29957=CARTESIAN_POINT('Ctrl Pts',(-41.7512245751282,37.4437411776422,38.4499365924771));
#29958=CARTESIAN_POINT('Ctrl Pts',(-41.7660283830335,37.4617896109258,38.4630218012165));
#29959=CARTESIAN_POINT('Ctrl Pts',(-41.7807339135895,37.4799960746643,38.4760002547544));
#29960=CARTESIAN_POINT('Ctrl Pts',(-41.7953392786647,37.4983582325443,38.488870287449));
#29961=CARTESIAN_POINT('Ctrl Pts',(-41.8099446437399,37.5167203904243,38.5017403201436));
#29962=CARTESIAN_POINT('Ctrl Pts',(-41.8244498433024,37.5352382424059,38.5145019319667));
#29963=CARTESIAN_POINT('Ctrl Pts',(-41.8388530148473,37.553909412325,38.5271534850154));
#29964=CARTESIAN_POINT('Ctrl Pts',(-41.8532561863922,37.5725805822442,38.539805038064));
#29965=CARTESIAN_POINT('Ctrl Pts',(-41.8675573298881,37.5914050700601,38.5523465323107));
#29966=CARTESIAN_POINT('Ctrl Pts',(-41.8817546089319,37.6103804603642,38.564776358009));
#29967=CARTESIAN_POINT('Ctrl Pts',(-41.8959518879759,37.6293558506681,38.5772061837074));
#29968=CARTESIAN_POINT('Ctrl Pts',(-41.9100453025368,37.6484821434189,38.5895243408303));
#29969=CARTESIAN_POINT('Ctrl Pts',(-41.9240330427824,37.6677568845784,38.601729248199));
#29970=CARTESIAN_POINT('Ctrl Pts',(-41.9380207830281,37.687031625738,38.6139341555677));
#29971=CARTESIAN_POINT('Ctrl Pts',(-41.9519028489279,37.7064548152644,38.6260258131555));
#29972=CARTESIAN_POINT('Ctrl Pts',(-41.9656774576819,37.7260239611165,38.6380026687541));
#29973=CARTESIAN_POINT('Ctrl Pts',(-41.979452066436,37.7455931069687,38.6499795243528));
#29974=CARTESIAN_POINT('Ctrl Pts',(-41.9931192180142,37.7653082091039,38.6618415779362));
#29975=CARTESIAN_POINT('Ctrl Pts',(-42.0066771571042,37.785166738113,38.6735873066626));
#29976=CARTESIAN_POINT('Ctrl Pts',(-42.0202350961943,37.8050252671221,38.6853330353891));
#29977=CARTESIAN_POINT('Ctrl Pts',(-42.0336838227664,37.8250272229619,38.696962439233));
#29978=CARTESIAN_POINT('Ctrl Pts',(-42.0470216094439,37.8451700394999,38.7084740251079));
#29979=CARTESIAN_POINT('Ctrl Pts',(-42.0603593961213,37.865312856038,38.7199856109827));
#29980=CARTESIAN_POINT('Ctrl Pts',(-42.0735862428749,37.8855965332304,38.7313793788634));
#29981=CARTESIAN_POINT('Ctrl Pts',(-42.0867004507042,37.9060184688758,38.7426538657995));
#29982=CARTESIAN_POINT('Ctrl Pts',(-42.0998146585335,37.9264404045212,38.7539283527356));
#29983=CARTESIAN_POINT('Ctrl Pts',(-42.1128162274098,37.9470005985752,38.7650835587024));
#29984=CARTESIAN_POINT('Ctrl Pts',(-42.1257034871429,37.9676964134305,38.7761180512591));
#29985=CARTESIAN_POINT('Ctrl Pts',(-42.138590746876,37.9883922282858,38.7871525438156));
#29986=CARTESIAN_POINT('Ctrl Pts',(-42.1513636974377,38.0092236638974,38.7980663229379));
#29987=CARTESIAN_POINT('Ctrl Pts',(-42.1640206978744,38.030188047925,38.8088579870595));
#29988=CARTESIAN_POINT('Ctrl Pts',(-42.176677698311,38.0511524319525,38.8196496511812));
#29989=CARTESIAN_POINT('Ctrl Pts',(-42.189218748595,38.0722497643502,38.8303192002788));
#29990=CARTESIAN_POINT('Ctrl Pts',(-42.2016422374281,38.0934773387253,38.8408652640187));
#29991=CARTESIAN_POINT('Ctrl Pts',(-42.2140657262613,38.1147049131006,38.8514113277587));
#29992=CARTESIAN_POINT('Ctrl Pts',(-42.2263716536165,38.136062729407,38.861833906118));
#29993=CARTESIAN_POINT('Ctrl Pts',(-42.2385584382627,38.1575480478897,38.8721316603454));
#29994=CARTESIAN_POINT('Ctrl Pts',(-42.2507560538243,38.1790524612914,38.8824385666263));
#29995=CARTESIAN_POINT('Ctrl Pts',(-42.2628343147816,38.2006846035563,38.8926204267812));
#29996=CARTESIAN_POINT('Ctrl Pts',(-42.2747916662362,38.2224416948671,38.9026759304956));
#29997=CARTESIAN_POINT('Ctrl Pts',(-41.6058635266892,37.286315601138,38.3391083125477));
#29998=CARTESIAN_POINT('Ctrl Pts',(-41.6217688958728,37.3040329697291,38.3533711969399));
#29999=CARTESIAN_POINT('Ctrl Pts',(-41.6375746651768,37.3219278508808,38.36752464459));
#30000=CARTESIAN_POINT('Ctrl Pts',(-41.6532786431145,37.3399977634488,38.3815666931073));
#30001=CARTESIAN_POINT('Ctrl Pts',(-41.6689826210522,37.3580676760168,38.3956087416246));
#30002=CARTESIAN_POINT('Ctrl Pts',(-41.6845848075833,37.3763126199546,38.4095393909731));
#30003=CARTESIAN_POINT('Ctrl Pts',(-41.7000830394478,37.3947300655812,38.4233567096532));
#30004=CARTESIAN_POINT('Ctrl Pts',(-41.7155812713123,37.4131475112078,38.4371740283333));
#30005=CARTESIAN_POINT('Ctrl Pts',(-41.7309755484705,37.4317374584759,38.4508780163097));
#30006=CARTESIAN_POINT('Ctrl Pts',(-41.7462637364893,37.4504973298695,38.4644667735097));
#30007=CARTESIAN_POINT('Ctrl Pts',(-41.7615519245081,37.4692572012631,38.4780555307096));
#30008=CARTESIAN_POINT('Ctrl Pts',(-41.7767340233484,37.4881869967341,38.4915290570984));
#30009=CARTESIAN_POINT('Ctrl Pts',(-41.7918079279958,37.5072840916458,38.5048854845569));
#30010=CARTESIAN_POINT('Ctrl Pts',(-41.8068818326432,37.5263811865576,38.5182419120155));
#30011=CARTESIAN_POINT('Ctrl Pts',(-41.8218475430591,37.5456455808612,38.5314812405097));
#30012=CARTESIAN_POINT('Ctrl Pts',(-41.8367029842316,37.5650746035277,38.5446016343923));
#30013=CARTESIAN_POINT('Ctrl Pts',(-41.8515584254041,37.5845036261943,38.5577220282749));
#30014=CARTESIAN_POINT('Ctrl Pts',(-41.8663035972952,37.6040972771739,38.5707234875124));
#30015=CARTESIAN_POINT('Ctrl Pts',(-41.8809364554709,37.6238528397859,38.5836042094385));
#30016=CARTESIAN_POINT('Ctrl Pts',(-41.8955693136467,37.6436084023978,38.5964849313646));
#30017=CARTESIAN_POINT('Ctrl Pts',(-41.9100898580695,37.6635258765915,38.6092449159461));
#30018=CARTESIAN_POINT('Ctrl Pts',(-41.9244960754504,37.6836025007876,38.6218823939976));
#30019=CARTESIAN_POINT('Ctrl Pts',(-41.9389022928313,37.7036791249839,38.6345198720492));
#30020=CARTESIAN_POINT('Ctrl Pts',(-41.9531941831333,37.723914899131,38.6470348435383));
#30021=CARTESIAN_POINT('Ctrl Pts',(-41.9673697647705,37.7443070175174,38.6594255732507));
#30022=CARTESIAN_POINT('Ctrl Pts',(-41.9815453464077,37.7646991359038,38.6718163029631));
#30023=CARTESIAN_POINT('Ctrl Pts',(-41.9956046193437,37.7852475984771,38.6840827908671));
#30024=CARTESIAN_POINT('Ctrl Pts',(-42.0095456342452,37.8059495561709,38.6962233362008));
#30025=CARTESIAN_POINT('Ctrl Pts',(-42.0234866491467,37.8266515138647,38.7083638815347));
#30026=CARTESIAN_POINT('Ctrl Pts',(-42.037309405978,37.847506966626,38.7203784842671));
#30027=CARTESIAN_POINT('Ctrl Pts',(-42.051011988199,37.8685130228238,38.7322654785607));
#30028=CARTESIAN_POINT('Ctrl Pts',(-42.0647145704201,37.8895190790215,38.7441524728544));
#30029=CARTESIAN_POINT('Ctrl Pts',(-42.0782969779956,37.9106757386019,38.7559118586786));
#30030=CARTESIAN_POINT('Ctrl Pts',(-42.0917573277104,37.9319800681713,38.7675420055821));
#30031=CARTESIAN_POINT('Ctrl Pts',(-42.1052176774251,37.9532843977408,38.7791721524855));
#30032=CARTESIAN_POINT('Ctrl Pts',(-42.1185559692445,37.9747363972447,38.7906730604383));
#30033=CARTESIAN_POINT('Ctrl Pts',(-42.1317703538001,37.9963330923403,38.8020431348271));
#30034=CARTESIAN_POINT('Ctrl Pts',(-42.1449847383556,38.0179297874359,38.813413209216));
#30035=CARTESIAN_POINT('Ctrl Pts',(-42.1580752156135,38.0396711780678,38.8246524500119));
#30036=CARTESIAN_POINT('Ctrl Pts',(-42.1710399705648,38.0615542497689,38.8357592988819));
#30037=CARTESIAN_POINT('Ctrl Pts',(-42.1840047255163,38.0834373214698,38.8468661477519));
#30038=CARTESIAN_POINT('Ctrl Pts',(-42.196843758128,38.1054620741839,38.8578406046676));
#30039=CARTESIAN_POINT('Ctrl Pts',(-42.2095552882544,38.1276254541553,38.8686811480087));
#30040=CARTESIAN_POINT('Ctrl Pts',(-42.2222668183807,38.1497888341268,38.8795216913498));
#30041=CARTESIAN_POINT('Ctrl Pts',(-42.2348508459891,38.1720908412988,38.8902283210885));
#30042=CARTESIAN_POINT('Ctrl Pts',(-42.2473056262907,38.1945283834742,38.9007995527392));
#30043=CARTESIAN_POINT('Ctrl Pts',(-42.2597714756867,38.2169858668503,38.9113801794943));
#30044=CARTESIAN_POINT('Ctrl Pts',(-42.2721078479066,38.2395791261907,38.9218251673591));
#30045=CARTESIAN_POINT('Ctrl Pts',(-42.2843130294414,38.2623050233617,38.9321330655328));
#30046=CARTESIAN_POINT('Ctrl Pts',(-41.5963383565818,37.286997481722,38.3488833491826));
#30047=CARTESIAN_POINT('Ctrl Pts',(-41.6127729656169,37.3053524258835,38.3636987489452));
#30048=CARTESIAN_POINT('Ctrl Pts',(-41.6291008388388,37.3238976006658,38.3783968712603));
#30049=CARTESIAN_POINT('Ctrl Pts',(-41.6453195553693,37.3426302570077,38.3929755376294));
#30050=CARTESIAN_POINT('Ctrl Pts',(-41.6615382718997,37.3613629133496,38.4075542039984));
#30051=CARTESIAN_POINT('Ctrl Pts',(-41.6776478316914,37.3802830511966,38.4220134143787));
#30052=CARTESIAN_POINT('Ctrl Pts',(-41.6936458461577,37.3993878660215,38.43635102561));
#30053=CARTESIAN_POINT('Ctrl Pts',(-41.7096438606239,37.4184926808463,38.4506886368413));
#30054=CARTESIAN_POINT('Ctrl Pts',(-41.725530329718,37.4377821725933,38.4649046488818));
#30055=CARTESIAN_POINT('Ctrl Pts',(-41.7413028978504,37.4572534820969,38.4789969545423));
#30056=CARTESIAN_POINT('Ctrl Pts',(-41.7570754659828,37.4767247916005,38.4930892602028));
#30057=CARTESIAN_POINT('Ctrl Pts',(-41.7727341331073,37.4963779188038,38.5070578594423));
#30058=CARTESIAN_POINT('Ctrl Pts',(-41.7882765773269,37.5162099507473,38.5209006816648));
#30059=CARTESIAN_POINT('Ctrl Pts',(-41.8038190215465,37.5360419826907,38.5347435038874));
#30060=CARTESIAN_POINT('Ctrl Pts',(-41.8192452428157,37.5560529193164,38.5484605490526));
#30061=CARTESIAN_POINT('Ctrl Pts',(-41.8345529536159,37.5762397947304,38.5620497837692));
#30062=CARTESIAN_POINT('Ctrl Pts',(-41.849860664416,37.5964266701443,38.5756390184859));
#30063=CARTESIAN_POINT('Ctrl Pts',(-41.8650498647023,37.6167894842876,38.5891004427142));
#30064=CARTESIAN_POINT('Ctrl Pts',(-41.8801183020099,37.6373252192075,38.602432060868));
#30065=CARTESIAN_POINT('Ctrl Pts',(-41.8951867393174,37.6578609541275,38.6157636790217));
#30066=CARTESIAN_POINT('Ctrl Pts',(-41.9101344136022,37.6785696097642,38.6289654910619));
#30067=CARTESIAN_POINT('Ctrl Pts',(-41.9249591081184,37.6994481169969,38.6420355397963));
#30068=CARTESIAN_POINT('Ctrl Pts',(-41.9397838026345,37.7203266242297,38.6551055885306));
#30069=CARTESIAN_POINT('Ctrl Pts',(-41.9544855173388,37.7413749829976,38.668043873921));
#30070=CARTESIAN_POINT('Ctrl Pts',(-41.9690620718591,37.7625900739183,38.6808484777472));
#30071=CARTESIAN_POINT('Ctrl Pts',(-41.9836386263794,37.7838051648389,38.6936530815734));
#30072=CARTESIAN_POINT('Ctrl Pts',(-41.9980900206732,37.8051869878503,38.706324003798));
#30073=CARTESIAN_POINT('Ctrl Pts',(-42.0124141113862,37.8267323742288,38.7188593657391));
#30074=CARTESIAN_POINT('Ctrl Pts',(-42.0267382020992,37.8482777606074,38.7313947276802));
#30075=CARTESIAN_POINT('Ctrl Pts',(-42.0409349891896,37.8699867102901,38.7437945293013));
#30076=CARTESIAN_POINT('Ctrl Pts',(-42.0550023669542,37.8918560061476,38.7560569320136));
#30077=CARTESIAN_POINT('Ctrl Pts',(-42.0690697447188,37.913725302005,38.768319334726));
#30078=CARTESIAN_POINT('Ctrl Pts',(-42.0830077131163,37.9357549439734,38.7804443384939));
#30079=CARTESIAN_POINT('Ctrl Pts',(-42.0968142047165,37.9579416674669,38.7924301453646));
#30080=CARTESIAN_POINT('Ctrl Pts',(-42.1106206963167,37.9801283909604,38.8044159522353));
#30081=CARTESIAN_POINT('Ctrl Pts',(-42.1242957110792,38.0024721959143,38.8162625621741));
#30082=CARTESIAN_POINT('Ctrl Pts',(-42.1378372204572,38.0249697712501,38.8279682183953));
#30083=CARTESIAN_POINT('Ctrl Pts',(-42.1513787298352,38.047467346586,38.8396738746164));
#30084=CARTESIAN_POINT('Ctrl Pts',(-42.1647867337893,38.0701186922381,38.851238577086));
#30085=CARTESIAN_POINT('Ctrl Pts',(-42.1780592432554,38.0929204516126,38.8626606107043));
#30086=CARTESIAN_POINT('Ctrl Pts',(-42.1913317527215,38.1157222109872,38.8740826443226));
#30087=CARTESIAN_POINT('Ctrl Pts',(-42.204468767661,38.1386743840176,38.8853620090564));
#30088=CARTESIAN_POINT('Ctrl Pts',(-42.2174683390806,38.1617735695853,38.8964970319986));
#30089=CARTESIAN_POINT('Ctrl Pts',(-42.2304679105001,38.1848727551531,38.9076320549408));
#30090=CARTESIAN_POINT('Ctrl Pts',(-42.2433300383618,38.2081189531906,38.9186227360591));
#30091=CARTESIAN_POINT('Ctrl Pts',(-42.2560528143186,38.2315087190587,38.9294674451329));
#30092=CARTESIAN_POINT('Ctrl Pts',(-42.2687868975491,38.2549192724092,38.9403217923623));
#30093=CARTESIAN_POINT('Ctrl Pts',(-42.2813813810315,38.278473648825,38.9510299079371));
#30094=CARTESIAN_POINT('Ctrl Pts',(-42.2938343926466,38.3021683518564,38.9615902005701));
#30095=CARTESIAN_POINT('Ctrl Pts',(-41.5867897802837,37.2876520376445,38.3586353659586));
#30096=CARTESIAN_POINT('Ctrl Pts',(-41.6037304885494,37.3066182518131,38.3739816725687));
#30097=CARTESIAN_POINT('Ctrl Pts',(-41.620557238131,37.3257875696053,38.3892027655024));
#30098=CARTESIAN_POINT('Ctrl Pts',(-41.6372673645311,37.3451569561447,38.4042962352317));
#30099=CARTESIAN_POINT('Ctrl Pts',(-41.6539774909312,37.3645263426841,38.4193897049609));
#30100=CARTESIAN_POINT('Ctrl Pts',(-41.6705709940942,37.3840957979064,38.4343555514354));
#30101=CARTESIAN_POINT('Ctrl Pts',(-41.6870452463718,37.4038622237152,38.4491914054513));
#30102=CARTESIAN_POINT('Ctrl Pts',(-41.7035194986494,37.4236286495241,38.4640272594672));
#30103=CARTESIAN_POINT('Ctrl Pts',(-41.7198744999866,37.4435920458539,38.4787331209752));
#30104=CARTESIAN_POINT('Ctrl Pts',(-41.7361076604127,37.4637492523649,38.493306661843));
#30105=CARTESIAN_POINT('Ctrl Pts',(-41.7523408208388,37.483906458876,38.5078802027108));
#30106=CARTESIAN_POINT('Ctrl Pts',(-41.7684521402996,37.5042574755014,38.5223214228898));
#30107=CARTESIAN_POINT('Ctrl Pts',(-41.7844390673187,37.5247990806544,38.5366280360533));
#30108=CARTESIAN_POINT('Ctrl Pts',(-41.8004259943379,37.5453406858074,38.5509346492168));
#30109=CARTESIAN_POINT('Ctrl Pts',(-41.8162885288619,37.5660728794197,38.5651066553171));
#30110=CARTESIAN_POINT('Ctrl Pts',(-41.8320241587134,37.5869923796731,38.5791418105536));
#30111=CARTESIAN_POINT('Ctrl Pts',(-41.8477597885648,37.6079118799265,38.59317696579));
#30112=CARTESIAN_POINT('Ctrl Pts',(-41.8633685136913,37.6290186867515,38.6070752701159));
#30113=CARTESIAN_POINT('Ctrl Pts',(-41.8788478620063,37.6503094591325,38.6208345229642));
#30114=CARTESIAN_POINT('Ctrl Pts',(-41.8943272103213,37.6716002315136,38.6345937758125));
#30115=CARTESIAN_POINT('Ctrl Pts',(-41.9096771817734,37.69307496938,38.6482139771374));
#30116=CARTESIAN_POINT('Ctrl Pts',(-41.924895345147,37.7147302735725,38.6616929702995));
#30117=CARTESIAN_POINT('Ctrl Pts',(-41.9401135085206,37.736385577765,38.6751719634615));
#30118=CARTESIAN_POINT('Ctrl Pts',(-41.9551998637651,37.7582214482115,38.6885097484157));
#30119=CARTESIAN_POINT('Ctrl Pts',(-41.9701520213029,37.7802344286799,38.7017042131301));
#30120=CARTESIAN_POINT('Ctrl Pts',(-41.9851041788406,37.8022474091484,38.7148986778445));
#30121=CARTESIAN_POINT('Ctrl Pts',(-41.9999221386806,37.8244374997358,38.7279498224257));
#30122=CARTESIAN_POINT('Ctrl Pts',(-42.0146035535198,37.8468011878927,38.7408555798182));
#30123=CARTESIAN_POINT('Ctrl Pts',(-42.029284968359,37.8691648760496,38.7537613372108));
#30124=CARTESIAN_POINT('Ctrl Pts',(-42.0438298382064,37.8917021618657,38.766521707518));
#30125=CARTESIAN_POINT('Ctrl Pts',(-42.058235859008,37.9144094782492,38.7791346699066));
#30126=CARTESIAN_POINT('Ctrl Pts',(-42.0726418798095,37.9371167946327,38.7917476322951));
#30127=CARTESIAN_POINT('Ctrl Pts',(-42.0869090515172,37.9599941415081,38.8042131867229));
#30128=CARTESIAN_POINT('Ctrl Pts',(-42.1010351139354,37.9830378980317,38.8165293589193));
#30129=CARTESIAN_POINT('Ctrl Pts',(-42.1151611763537,38.0060816545551,38.8288455311156));
#30130=CARTESIAN_POINT('Ctrl Pts',(-42.1291461294356,38.0292918206501,38.8410123210396));
#30131=CARTESIAN_POINT('Ctrl Pts',(-42.1429877575575,38.0526647228616,38.8530278016054));
#30132=CARTESIAN_POINT('Ctrl Pts',(-42.1568293856795,38.0760376250732,38.8650432821713));
#30133=CARTESIAN_POINT('Ctrl Pts',(-42.1705276887953,38.0995732633236,38.8769074533392));
#30134=CARTESIAN_POINT('Ctrl Pts',(-42.1840804965524,38.1232679127047,38.8886184358165));
#30135=CARTESIAN_POINT('Ctrl Pts',(-42.1976333043096,38.1469625620857,38.900329418294));
#30136=CARTESIAN_POINT('Ctrl Pts',(-42.2110406166629,38.1708162225187,38.9118872120419));
#30137=CARTESIAN_POINT('Ctrl Pts',(-42.2243003092155,38.1948251188158,38.9232899861538));
#30138=CARTESIAN_POINT('Ctrl Pts',(-42.2375600017681,38.218834015113,38.9346927602656));
#30139=CARTESIAN_POINT('Ctrl Pts',(-42.2506720744758,38.2429981471945,38.9459405147036));
#30140=CARTESIAN_POINT('Ctrl Pts',(-42.2636344495679,38.2673136907831,38.9570314675243));
#30141=CARTESIAN_POINT('Ctrl Pts',(-42.2766083448756,38.2916508446324,38.968132277348));
#30142=CARTESIAN_POINT('Ctrl Pts',(-42.2894322762548,38.3161396788477,38.9790760064518));
#30143=CARTESIAN_POINT('Ctrl Pts',(-42.3021042079305,38.3407763115497,38.9898609182514));
#30144=CARTESIAN_POINT('Ctrl Pts',(-41.5772224901889,37.2882847468617,38.3683689778196));
#30145=CARTESIAN_POINT('Ctrl Pts',(-41.5946507223381,37.3078407290261,38.3842282194709));
#30146=CARTESIAN_POINT('Ctrl Pts',(-41.6119577122494,37.327612795967,38.3999542445415));
#30147=CARTESIAN_POINT('Ctrl Pts',(-41.6291405389079,37.3475976106221,38.4155443988461));
#30148=CARTESIAN_POINT('Ctrl Pts',(-41.6463233655664,37.3675824252771,38.4311345531509));
#30149=CARTESIAN_POINT('Ctrl Pts',(-41.663382028907,37.3877799875703,38.4465888366305));
#30150=CARTESIAN_POINT('Ctrl Pts',(-41.6803136498262,37.4081868886259,38.4619046409637));
#30151=CARTESIAN_POINT('Ctrl Pts',(-41.6972452707455,37.4285937896815,38.4772204452969));
#30152=CARTESIAN_POINT('Ctrl Pts',(-41.7140498491792,37.4492100294219,38.4923977704254));
#30153=CARTESIAN_POINT('Ctrl Pts',(-41.7307245489078,37.4700321283081,38.5074340547719));
#30154=CARTESIAN_POINT('Ctrl Pts',(-41.7473992486363,37.4908542271945,38.5224703391184));
#30155=CARTESIAN_POINT('Ctrl Pts',(-41.7639440695964,37.5118821851476,38.5373655826258));
#30156=CARTESIAN_POINT('Ctrl Pts',(-41.7803562194093,37.5331124531404,38.5521172713255));
#30157=CARTESIAN_POINT('Ctrl Pts',(-41.7967683692221,37.5543427211332,38.5668689600252));
#30158=CARTESIAN_POINT('Ctrl Pts',(-41.8130478478255,37.5757752990849,38.5814770938612));
#30159=CARTESIAN_POINT('Ctrl Pts',(-41.8291919076243,37.5974065696779,38.5959392073223));
#30160=CARTESIAN_POINT('Ctrl Pts',(-41.8453359674232,37.6190378402709,38.6104013207834));
#30161=CARTESIAN_POINT('Ctrl Pts',(-41.8613446083561,37.6408678034231,38.6247174138146));
#30162=CARTESIAN_POINT('Ctrl Pts',(-41.8772151285393,37.6628927747474,38.6388850701946));
#30163=CARTESIAN_POINT('Ctrl Pts',(-41.8930856487224,37.6849177460716,38.6530527265745));
#30164=CARTESIAN_POINT('Ctrl Pts',(-41.9088180480953,37.7071377254845,38.6670719462493));
#30165=CARTESIAN_POINT('Ctrl Pts',(-41.9244096713972,37.7295489627732,38.6809403631027));
#30166=CARTESIAN_POINT('Ctrl Pts',(-41.9400012946991,37.7519602000619,38.694808779956));
#30167=CARTESIAN_POINT('Ctrl Pts',(-41.9554521418707,37.7745626951413,38.7085263939354));
#30168=CARTESIAN_POINT('Ctrl Pts',(-41.9707596051706,37.7973526332393,38.7220908898283));
#30169=CARTESIAN_POINT('Ctrl Pts',(-41.9860670684705,37.8201425713374,38.7356553857213));
#30170=CARTESIAN_POINT('Ctrl Pts',(-42.001231147894,37.8431199525268,38.7490667636172));
#30171=CARTESIAN_POINT('Ctrl Pts',(-42.016249283993,37.8662808984502,38.7623227597117));
#30172=CARTESIAN_POINT('Ctrl Pts',(-42.031267420092,37.8894418443737,38.7755787558061));
#30173=CARTESIAN_POINT('Ctrl Pts',(-42.0461396128623,37.9127863550969,38.7886793701855));
#30174=CARTESIAN_POINT('Ctrl Pts',(-42.0608633522257,37.9363104906126,38.8016223917728));
#30175=CARTESIAN_POINT('Ctrl Pts',(-42.075587091589,37.9598346261284,38.81456541336));
#30176=CARTESIAN_POINT('Ctrl Pts',(-42.0901623774896,37.9835383863474,38.8273508421058));
#30177=CARTESIAN_POINT('Ctrl Pts',(-42.1045867499601,38.0074177706295,38.8399765201292));
#30178=CARTESIAN_POINT('Ctrl Pts',(-42.1190111224306,38.0312971549117,38.8526021981525));
#30179=CARTESIAN_POINT('Ctrl Pts',(-42.1332845814163,38.0553521631663,38.8650681254053));
#30180=CARTESIAN_POINT('Ctrl Pts',(-42.1474047178913,38.0795787354709,38.8773721979308));
#30181=CARTESIAN_POINT('Ctrl Pts',(-42.1615248543663,38.1038053077755,38.8896762704562));
#30182=CARTESIAN_POINT('Ctrl Pts',(-42.175491668277,38.128203444038,38.9018184882076));
#30183=CARTESIAN_POINT('Ctrl Pts',(-42.1893028023519,38.1527690264238,38.9137968018627));
#30184=CARTESIAN_POINT('Ctrl Pts',(-42.2031139364269,38.1773346088097,38.9257751155178));
#30185=CARTESIAN_POINT('Ctrl Pts',(-42.2167693906136,38.2020676372257,38.9375895250311));
#30186=CARTESIAN_POINT('Ctrl Pts',(-42.2302668601911,38.2269639373153,38.9492380364066));
#30187=CARTESIAN_POINT('Ctrl Pts',(-42.2437643297685,38.2518602374049,38.9608865477822));
#30188=CARTESIAN_POINT('Ctrl Pts',(-42.2571038146854,38.2769198090737,38.9723691609758));
#30189=CARTESIAN_POINT('Ctrl Pts',(-42.2702830635487,38.302138422852,38.9836839379911));
#30190=CARTESIAN_POINT('Ctrl Pts',(-42.2834740253727,38.3273794494882,38.9950087709313));
#30191=CARTESIAN_POINT('Ctrl Pts',(-42.2965044660913,38.3527798006676,39.0061654689777));
#30192=CARTESIAN_POINT('Ctrl Pts',(-42.3093721826523,38.378335182382,39.0171521461915));
#30193=CARTESIAN_POINT('Ctrl Pts',(-41.5676552000942,37.2889174560789,38.3781025896805));
#30194=CARTESIAN_POINT('Ctrl Pts',(-41.5855709561268,37.3090632062391,38.3944747663732));
#30195=CARTESIAN_POINT('Ctrl Pts',(-41.6033581863678,37.3294380223288,38.4107057235805));
#30196=CARTESIAN_POINT('Ctrl Pts',(-41.6210137132847,37.3500382650995,38.4267925624606));
#30197=CARTESIAN_POINT('Ctrl Pts',(-41.6386692402017,37.3706385078701,38.4428794013408));
#30198=CARTESIAN_POINT('Ctrl Pts',(-41.6561930637196,37.3914641772344,38.4588221218257));
#30199=CARTESIAN_POINT('Ctrl Pts',(-41.6735820532807,37.4125115535366,38.4746178764762));
#30200=CARTESIAN_POINT('Ctrl Pts',(-41.6909710428417,37.4335589298388,38.4904136311266));
#30201=CARTESIAN_POINT('Ctrl Pts',(-41.7082251983718,37.4548280129899,38.5060624198756));
#30202=CARTESIAN_POINT('Ctrl Pts',(-41.7253414374028,37.4763150042514,38.5215614477008));
#30203=CARTESIAN_POINT('Ctrl Pts',(-41.7424576764339,37.4978019955129,38.5370604755261));
#30204=CARTESIAN_POINT('Ctrl Pts',(-41.759435998893,37.519506894794,38.5524097423618));
#30205=CARTESIAN_POINT('Ctrl Pts',(-41.7762733714997,37.5414258256264,38.5676065065977));
#30206=CARTESIAN_POINT('Ctrl Pts',(-41.7931107441064,37.563344756459,38.5828032708336));
#30207=CARTESIAN_POINT('Ctrl Pts',(-41.8098071667891,37.5854777187501,38.5978475324052));
#30208=CARTESIAN_POINT('Ctrl Pts',(-41.8263596565353,37.6078207596827,38.612736604091));
#30209=CARTESIAN_POINT('Ctrl Pts',(-41.8429121462815,37.6301638006153,38.6276256757767));
#30210=CARTESIAN_POINT('Ctrl Pts',(-41.859320703021,37.6527169200947,38.6423595575134));
#30211=CARTESIAN_POINT('Ctrl Pts',(-41.8755823950722,37.6754760903623,38.6569356174249));
#30212=CARTESIAN_POINT('Ctrl Pts',(-41.8918440871234,37.6982352606297,38.6715116773365));
#30213=CARTESIAN_POINT('Ctrl Pts',(-41.9079589144172,37.7212004815889,38.6859299153611));
#30214=CARTESIAN_POINT('Ctrl Pts',(-41.9239239976474,37.7443676519738,38.7001877559059));
#30215=CARTESIAN_POINT('Ctrl Pts',(-41.9398890808776,37.7675348223587,38.7144455964506));
#30216=CARTESIAN_POINT('Ctrl Pts',(-41.9557044199763,37.7909039420712,38.728543039455));
#30217=CARTESIAN_POINT('Ctrl Pts',(-41.9713671890384,37.8144708377988,38.7424775665265));
#30218=CARTESIAN_POINT('Ctrl Pts',(-41.9870299581004,37.8380377335264,38.756412093598));
#30219=CARTESIAN_POINT('Ctrl Pts',(-42.0025401571074,37.8618024053179,38.7701837048088));
#30220=CARTESIAN_POINT('Ctrl Pts',(-42.0178950144663,37.8857606090078,38.7837899396051));
#30221=CARTESIAN_POINT('Ctrl Pts',(-42.0332498718251,37.9097188126977,38.7973961744014));
#30222=CARTESIAN_POINT('Ctrl Pts',(-42.0484493875181,37.933870548328,38.810837032853));
#30223=CARTESIAN_POINT('Ctrl Pts',(-42.0634908454433,37.958211502976,38.824110113639));
#30224=CARTESIAN_POINT('Ctrl Pts',(-42.0785323033685,37.9825524576241,38.8373831944249));
#30225=CARTESIAN_POINT('Ctrl Pts',(-42.093415703462,38.0070826311866,38.8504884974888));
#30226=CARTESIAN_POINT('Ctrl Pts',(-42.1081383859847,38.0317976432275,38.8634236813391));
#30227=CARTESIAN_POINT('Ctrl Pts',(-42.1228610685075,38.0565126552683,38.8763588651893));
#30228=CARTESIAN_POINT('Ctrl Pts',(-42.1374230333971,38.0814125056826,38.8891239297711));
#30229=CARTESIAN_POINT('Ctrl Pts',(-42.1518216782251,38.1064927480802,38.9017165942561));
#30230=CARTESIAN_POINT('Ctrl Pts',(-42.1662203230532,38.1315729904777,38.9143092587412));
#30231=CARTESIAN_POINT('Ctrl Pts',(-42.1804556477587,38.1568336247523,38.9267295230761));
#30232=CARTESIAN_POINT('Ctrl Pts',(-42.1945251081514,38.182270140143,38.9389751679089));
#30233=CARTESIAN_POINT('Ctrl Pts',(-42.2085945685441,38.2077066555336,38.9512208127417));
#30234=CARTESIAN_POINT('Ctrl Pts',(-42.2224981645643,38.2333190519327,38.9632918380203));
#30235=CARTESIAN_POINT('Ctrl Pts',(-42.2362334111666,38.2591027558148,38.9751860866595));
#30236=CARTESIAN_POINT('Ctrl Pts',(-42.2499686577689,38.2848864596969,38.9870803352988));
#30237=CARTESIAN_POINT('Ctrl Pts',(-42.2635355548949,38.3108414709527,38.9987978072482));
#30238=CARTESIAN_POINT('Ctrl Pts',(-42.2769316775296,38.3369631549211,39.0103364084579));
#30239=CARTESIAN_POINT('Ctrl Pts',(-42.2903397058698,38.3631080543441,39.0218852645147));
#30240=CARTESIAN_POINT('Ctrl Pts',(-42.3035766559278,38.3894199224876,39.0332549315036));
#30241=CARTESIAN_POINT('Ctrl Pts',(-42.3166401573741,38.4158940532142,39.0444433741316));
#30242=CARTESIAN_POINT('Ctrl Pts',(-41.5580691595818,37.2895282758387,38.3878177606096));
#30243=CARTESIAN_POINT('Ctrl Pts',(-41.576453838129,37.3102422736121,38.4046848944203));
#30244=CARTESIAN_POINT('Ctrl Pts',(-41.5947026462334,37.3311984273574,38.4214027387092));
#30245=CARTESIAN_POINT('Ctrl Pts',(-41.6128121369395,37.3523927792619,38.4379681363462));
#30246=CARTESIAN_POINT('Ctrl Pts',(-41.6309216276457,37.3735871311664,38.4545335339833));
#30247=CARTESIAN_POINT('Ctrl Pts',(-41.6488918008674,37.39501968113,38.4709464848899));
#30248=CARTESIAN_POINT('Ctrl Pts',(-41.6667192621919,37.4166863814999,38.4872038894299));
#30249=CARTESIAN_POINT('Ctrl Pts',(-41.6845467235163,37.4383530818698,38.5034612939699));
#30250=CARTESIAN_POINT('Ctrl Pts',(-41.7022314728587,37.4602539325432,38.5195631520664));
#30251=CARTESIAN_POINT('Ctrl Pts',(-41.7197701696272,37.482384797551,38.5355064227447));
#30252=CARTESIAN_POINT('Ctrl Pts',(-41.7373088663957,37.5045156625588,38.551449693423));
#30253=CARTESIAN_POINT('Ctrl Pts',(-41.754701510507,37.5268765417961,38.5672343766076));
#30254=CARTESIAN_POINT('Ctrl Pts',(-41.7719448164483,37.5494632125342,38.5828574911305));
#30255=CARTESIAN_POINT('Ctrl Pts',(-41.7891881223896,37.5720498832724,38.5984806056533));
#30256=CARTESIAN_POINT('Ctrl Pts',(-41.8062820900792,37.5948623454045,38.6139421514404));
#30257=CARTESIAN_POINT('Ctrl Pts',(-41.8232234903209,37.6178962910326,38.6292392082528));
#30258=CARTESIAN_POINT('Ctrl Pts',(-41.8401648905627,37.6409302366608,38.6445362650652));
#30259=CARTESIAN_POINT('Ctrl Pts',(-41.8569537232762,37.6641856656757,38.6596688328305));
#30260=CARTESIAN_POINT('Ctrl Pts',(-41.8735868167985,37.6876581866323,38.6746340533385));
#30261=CARTESIAN_POINT('Ctrl Pts',(-41.8902199103208,37.7111307075889,38.6895992738465));
#30262=CARTESIAN_POINT('Ctrl Pts',(-41.9066972645729,37.7348203203759,38.7043971470262));
#30263=CARTESIAN_POINT('Ctrl Pts',(-41.9230157666195,37.7587225516539,38.7190248777729));
#30264=CARTESIAN_POINT('Ctrl Pts',(-41.939334268666,37.782624782932,38.7336526085196));
#30265=CARTESIAN_POINT('Ctrl Pts',(-41.9554939184296,37.8067396325878,38.7481101967638));
#30266=CARTESIAN_POINT('Ctrl Pts',(-41.971491662875,37.8310625470722,38.7623949115585));
#30267=CARTESIAN_POINT('Ctrl Pts',(-41.9874894073204,37.8553854615566,38.7766796263532));
#30268=CARTESIAN_POINT('Ctrl Pts',(-42.0033252463718,37.8799164407544,38.7907914676305));
#30269=CARTESIAN_POINT('Ctrl Pts',(-42.0189961880445,37.9046508526205,38.8047277696299));
#30270=CARTESIAN_POINT('Ctrl Pts',(-42.0346671297171,37.9293852644866,38.8186640716294));
#30271=CARTESIAN_POINT('Ctrl Pts',(-42.0501731739366,37.9543231089039,38.8324248342847));
#30272=CARTESIAN_POINT('Ctrl Pts',(-42.0655113908957,37.9794596770759,38.8460074580256));
#30273=CARTESIAN_POINT('Ctrl Pts',(-42.0808496078549,38.0045962452478,38.8595900817665));
#30274=CARTESIAN_POINT('Ctrl Pts',(-42.0960199974808,38.0299315370551,38.8729945665287));
#30275=CARTESIAN_POINT('Ctrl Pts',(-42.1110196932476,38.0554607687221,38.8862183799112));
#30276=CARTESIAN_POINT('Ctrl Pts',(-42.1260193890143,38.0809900003891,38.8994421932938));
#30277=CARTESIAN_POINT('Ctrl Pts',(-42.1408483908508,38.1067131717948,38.912485335234));
#30278=CARTESIAN_POINT('Ctrl Pts',(-42.1555038965921,38.1326254259851,38.9253453414547));
#30279=CARTESIAN_POINT('Ctrl Pts',(-42.1701594023335,38.1585376801753,38.9382053476754));
#30280=CARTESIAN_POINT('Ctrl Pts',(-42.1846414119102,38.1846390170274,38.9508822181156));
#30281=CARTESIAN_POINT('Ctrl Pts',(-42.1989471885747,38.2109245082375,38.9633735575496));
#30282=CARTESIAN_POINT('Ctrl Pts',(-42.2132529652392,38.2372099994476,38.9758648969837));
#30283=CARTESIAN_POINT('Ctrl Pts',(-42.2273825089236,38.263679644891,38.9881707053525));
#30284=CARTESIAN_POINT('Ctrl Pts',(-42.2413331493284,38.2903284467695,39.0002886573846));
#30285=CARTESIAN_POINT('Ctrl Pts',(-42.2552837897332,38.3169772486478,39.0124066094168));
#30286=CARTESIAN_POINT('Ctrl Pts',(-42.2690555267923,38.3438052068348,39.0243367050547));
#30287=CARTESIAN_POINT('Ctrl Pts',(-42.2826457576608,38.3708072559186,39.0360766898576));
#30288=CARTESIAN_POINT('Ctrl Pts',(-42.2962480667472,38.3978333028752,39.0478271084856));
#30289=CARTESIAN_POINT('Ctrl Pts',(-42.3096685468105,38.425033750182,39.0593870781533));
#30290=CARTESIAN_POINT('Ctrl Pts',(-42.3229046566779,38.452403453028,39.0707544102742));
#30291=CARTESIAN_POINT('Ctrl Pts',(-41.5484677647746,37.2901211708148,38.3975178306748));
#30292=CARTESIAN_POINT('Ctrl Pts',(-41.5673061531269,37.311385584891,38.4148648435003));
#30293=CARTESIAN_POINT('Ctrl Pts',(-41.5860012811259,37.3329053256431,38.4320544470383));
#30294=CARTESIAN_POINT('Ctrl Pts',(-41.6045494205091,37.3546761015114,38.4490832132649));
#30295=CARTESIAN_POINT('Ctrl Pts',(-41.6230975598923,37.3764468773797,38.4661119794914));
#30296=CARTESIAN_POINT('Ctrl Pts',(-41.6414987105613,37.3984686882489,38.4829799083159));
#30297=CARTESIAN_POINT('Ctrl Pts',(-41.6597492028795,37.420737142435,38.4996836358636));
#30298=CARTESIAN_POINT('Ctrl Pts',(-41.6779996951978,37.443005596621,38.5163873634113));
#30299=CARTESIAN_POINT('Ctrl Pts',(-41.6960995290685,37.4655206940058,38.5329268895937));
#30300=CARTESIAN_POINT('Ctrl Pts',(-41.7140450949451,37.488277944532,38.5492989160273));
#30301=CARTESIAN_POINT('Ctrl Pts',(-41.7319906608217,37.5110351950581,38.5656709424609));
#30302=CARTESIAN_POINT('Ctrl Pts',(-41.7497819586091,37.5340345986049,38.581875469059));
#30303=CARTESIAN_POINT('Ctrl Pts',(-41.7674154402901,37.5572715685325,38.5979092642452));
#30304=CARTESIAN_POINT('Ctrl Pts',(-41.7850489219711,37.5805085384601,38.6139430594314));
#30305=CARTESIAN_POINT('Ctrl Pts',(-41.8025245874523,37.6039830746453,38.6298061231207));
#30306=CARTESIAN_POINT('Ctrl Pts',(-41.8198389516615,37.6276904956952,38.6454952918329));
#30307=CARTESIAN_POINT('Ctrl Pts',(-41.8371533158706,37.6513979167452,38.6611844605451));
#30308=CARTESIAN_POINT('Ctrl Pts',(-41.8543063787158,37.6753382225342,38.6766997341969));
#30309=CARTESIAN_POINT('Ctrl Pts',(-41.8712947194597,37.6995066387835,38.6920380186659));
#30310=CARTESIAN_POINT('Ctrl Pts',(-41.8882830602036,37.723675055033,38.7073763031348));
#30311=CARTESIAN_POINT('Ctrl Pts',(-41.9051066787561,37.7480715816146,38.7225375983396));
#30312=CARTESIAN_POINT('Ctrl Pts',(-41.9217622200788,37.7726913532685,38.7375188807495));
#30313=CARTESIAN_POINT('Ctrl Pts',(-41.9384177614015,37.7973111249223,38.7525001631594));
#30314=CARTESIAN_POINT('Ctrl Pts',(-41.9549052254061,37.8221541415177,38.7673014326951));
#30315=CARTESIAN_POINT('Ctrl Pts',(-41.9712213240919,37.8472154487537,38.7819197376237));
#30316=CARTESIAN_POINT('Ctrl Pts',(-41.9875374227776,37.8722767559897,38.7965380425524));
#30317=CARTESIAN_POINT('Ctrl Pts',(-42.003682156058,37.8975563537332,38.8109733827966));
#30318=CARTESIAN_POINT('Ctrl Pts',(-42.0196523042808,37.9230492006185,38.8252228795986));
#30319=CARTESIAN_POINT('Ctrl Pts',(-42.0356224525036,37.9485420475038,38.8394723764007));
#30320=CARTESIAN_POINT('Ctrl Pts',(-42.0514180155842,37.9742481433955,38.8535360296852));
#30321=CARTESIAN_POINT('Ctrl Pts',(-42.0670358435035,38.0001623618738,38.8674110348178));
#30322=CARTESIAN_POINT('Ctrl Pts',(-42.0826536714229,38.0260765803519,38.8812860399505));
#30323=CARTESIAN_POINT('Ctrl Pts',(-42.0980937640983,38.0521989212791,38.8949723968578));
#30324=CARTESIAN_POINT('Ctrl Pts',(-42.1133530424,38.0785241752259,38.9084673761477));
#30325=CARTESIAN_POINT('Ctrl Pts',(-42.1286123207017,38.1048494291727,38.9219623554375));
#30326=CARTESIAN_POINT('Ctrl Pts',(-42.1436907845489,38.1313775959995,38.9352659570384));
#30327=CARTESIAN_POINT('Ctrl Pts',(-42.1585854269294,38.1581033853453,38.9483755278889));
#30328=CARTESIAN_POINT('Ctrl Pts',(-42.17348006931,38.1848291746911,38.9614850987395));
#30329=CARTESIAN_POINT('Ctrl Pts',(-42.188190890145,38.2117525864143,38.9744006387701));
#30330=CARTESIAN_POINT('Ctrl Pts',(-42.2027149557394,38.2388682513324,38.9871195723083));
#30331=CARTESIAN_POINT('Ctrl Pts',(-42.2172390213338,38.2659839162503,38.9998385058467));
#30332=CARTESIAN_POINT('Ctrl Pts',(-42.2315763316105,38.2932918342195,39.0123608328251));
#30333=CARTESIAN_POINT('Ctrl Pts',(-42.2457240273616,38.3207865593774,39.0246840559876));
#30334=CARTESIAN_POINT('Ctrl Pts',(-42.2598717231127,38.3482812845353,39.0370072791501));
#30335=CARTESIAN_POINT('Ctrl Pts',(-42.2738298042631,38.3759628167363,39.0491313984311));
#30336=CARTESIAN_POINT('Ctrl Pts',(-42.2875954872323,38.4038256356102,39.0610539959869));
#30337=CARTESIAN_POINT('Ctrl Pts',(-42.3013734043511,38.4317132173598,39.0729871896636));
#30338=CARTESIAN_POINT('Ctrl Pts',(-42.3149585810787,38.4597824080118,39.0847185031907));
#30339=CARTESIAN_POINT('Ctrl Pts',(-42.3283483033489,38.4880275999658,39.0962455928629));
#30340=CARTESIAN_POINT('Ctrl Pts',(-41.5388663699673,37.2907140657908,38.4072179007401));
#30341=CARTESIAN_POINT('Ctrl Pts',(-41.5581584681248,37.3125288961699,38.4250447925802));
#30342=CARTESIAN_POINT('Ctrl Pts',(-41.5772999160183,37.3346122239288,38.4427061553675));
#30343=CARTESIAN_POINT('Ctrl Pts',(-41.5962867040786,37.3569594237608,38.4601982901835));
#30344=CARTESIAN_POINT('Ctrl Pts',(-41.615273492139,37.3793066235928,38.4776904249995));
#30345=CARTESIAN_POINT('Ctrl Pts',(-41.6341056202551,37.4019176953677,38.495013331742));
#30346=CARTESIAN_POINT('Ctrl Pts',(-41.6527791435672,37.42478790337,38.5121633822974));
#30347=CARTESIAN_POINT('Ctrl Pts',(-41.6714526668793,37.4476581113723,38.5293134328528));
#30348=CARTESIAN_POINT('Ctrl Pts',(-41.6899675852783,37.4707874554685,38.546290627121));
#30349=CARTESIAN_POINT('Ctrl Pts',(-41.708320020263,37.4941710915129,38.5630914093099));
#30350=CARTESIAN_POINT('Ctrl Pts',(-41.7266724552478,37.5175547275574,38.5798921914988));
#30351=CARTESIAN_POINT('Ctrl Pts',(-41.7448624067111,37.5411926554138,38.5965165615103));
#30352=CARTESIAN_POINT('Ctrl Pts',(-41.7628860641319,37.5650799245308,38.6129610373599));
#30353=CARTESIAN_POINT('Ctrl Pts',(-41.7809097215526,37.5889671936478,38.6294055132095));
#30354=CARTESIAN_POINT('Ctrl Pts',(-41.7987670848255,37.6131038038861,38.6456700948011));
#30355=CARTESIAN_POINT('Ctrl Pts',(-41.816454413002,37.6374847003579,38.661751375413));
#30356=CARTESIAN_POINT('Ctrl Pts',(-41.8341417411785,37.6618655968296,38.6778326560249));
#30357=CARTESIAN_POINT('Ctrl Pts',(-41.8516590341555,37.6864907793926,38.6937306355633));
#30358=CARTESIAN_POINT('Ctrl Pts',(-41.8690026221209,37.7113550909348,38.7094419839932));
#30359=CARTESIAN_POINT('Ctrl Pts',(-41.8863462100864,37.736219402477,38.7251533324231));
#30360=CARTESIAN_POINT('Ctrl Pts',(-41.9035160929392,37.7613228428534,38.7406780496528));
#30361=CARTESIAN_POINT('Ctrl Pts',(-41.920508673538,37.786660154883,38.756012883726));
#30362=CARTESIAN_POINT('Ctrl Pts',(-41.9375012541369,37.8119974669126,38.7713477177992));
#30363=CARTESIAN_POINT('Ctrl Pts',(-41.9543165323828,37.8375686504476,38.7864926686264));
#30364=CARTESIAN_POINT('Ctrl Pts',(-41.9709509853088,37.8633683504351,38.801444563689));
#30365=CARTESIAN_POINT('Ctrl Pts',(-41.9875854382349,37.8891680504226,38.8163964587517));
#30366=CARTESIAN_POINT('Ctrl Pts',(-42.0040390657441,37.9151962667122,38.8311552979626));
#30367=CARTESIAN_POINT('Ctrl Pts',(-42.020308420517,37.9414475486165,38.8457179895674));
#30368=CARTESIAN_POINT('Ctrl Pts',(-42.03657777529,37.967698830521,38.8602806811721));
#30369=CARTESIAN_POINT('Ctrl Pts',(-42.0526628572317,37.9941731778871,38.8746472250857));
#30370=CARTESIAN_POINT('Ctrl Pts',(-42.0685602961113,38.0208650466716,38.88881461161));
#30371=CARTESIAN_POINT('Ctrl Pts',(-42.084457734991,38.0475569154561,38.9029819981344));
#30372=CARTESIAN_POINT('Ctrl Pts',(-42.1001675307158,38.0744663055032,38.9169502271869));
#30373=CARTESIAN_POINT('Ctrl Pts',(-42.1156863915524,38.1015875817298,38.9307163723841));
#30374=CARTESIAN_POINT('Ctrl Pts',(-42.1312052523891,38.1287088579564,38.9444825175813));
#30375=CARTESIAN_POINT('Ctrl Pts',(-42.146533178247,38.1560420202043,38.9580465788428));
#30376=CARTESIAN_POINT('Ctrl Pts',(-42.1616669572668,38.1835813447057,38.9714057143231));
#30377=CARTESIAN_POINT('Ctrl Pts',(-42.1768007362866,38.211120669207,38.9847648498035));
#30378=CARTESIAN_POINT('Ctrl Pts',(-42.1917403683798,38.2388661558012,38.9979190594246));
#30379=CARTESIAN_POINT('Ctrl Pts',(-42.2064827229041,38.2668119944271,39.0108655870671));
#30380=CARTESIAN_POINT('Ctrl Pts',(-42.2212250774283,38.2947578330531,39.0238121147095));
#30381=CARTESIAN_POINT('Ctrl Pts',(-42.2357701542975,38.3229040235479,39.0365509602978));
#30382=CARTESIAN_POINT('Ctrl Pts',(-42.2501149053948,38.3512446719854,39.0490794545905));
#30383=CARTESIAN_POINT('Ctrl Pts',(-42.2644596564921,38.3795853204229,39.0616079488833));
#30384=CARTESIAN_POINT('Ctrl Pts',(-42.2786040817338,38.4081204266379,39.0739260918075));
#30385=CARTESIAN_POINT('Ctrl Pts',(-42.2925452168037,38.4368440153019,39.0860313021162));
#30386=CARTESIAN_POINT('Ctrl Pts',(-42.306498741955,38.4655931318444,39.0981472708417));
#30387=CARTESIAN_POINT('Ctrl Pts',(-42.320248615347,38.4945310658416,39.1100499282281));
#30388=CARTESIAN_POINT('Ctrl Pts',(-42.3337919500199,38.5236517469037,39.1217367754516));
#30389=CARTESIAN_POINT('Ctrl Pts',(-41.5292495984737,37.2912890098431,38.4169028479196));
#30390=CARTESIAN_POINT('Ctrl Pts',(-41.5489801744942,37.3136364084946,38.4351945310541));
#30391=CARTESIAN_POINT('Ctrl Pts',(-41.5685526648667,37.3362655562732,38.4533125154055));
#30392=CARTESIAN_POINT('Ctrl Pts',(-41.5879627668261,37.3591714789373,38.4712528185517));
#30393=CARTESIAN_POINT('Ctrl Pts',(-41.6073728687856,37.3820774016012,38.4891931216979));
#30394=CARTESIAN_POINT('Ctrl Pts',(-41.6266205822024,37.405260098996,38.5069557435165));
#30395=CARTESIAN_POINT('Ctrl Pts',(-41.6457016756296,37.4287144753495,38.5245367796226));
#30396=CARTESIAN_POINT('Ctrl Pts',(-41.6647827690567,37.452168851703,38.5421178157288));
#30397=CARTESIAN_POINT('Ctrl Pts',(-41.6836972423668,37.4758949068577,38.5595172660032));
#30398=CARTESIAN_POINT('Ctrl Pts',(-41.7024409372682,37.4998874257178,38.5767313057839));
#30399=CARTESIAN_POINT('Ctrl Pts',(-41.7211846321696,37.5238799445779,38.5939453455648));
#30400=CARTESIAN_POINT('Ctrl Pts',(-41.7397575485418,37.5481389269893,38.6109739747415));
#30401=CARTESIAN_POINT('Ctrl Pts',(-41.758155603082,37.5726590408337,38.6278134500664));
#30402=CARTESIAN_POINT('Ctrl Pts',(-41.7765536576222,37.5971791546782,38.6446529253913));
#30403=CARTESIAN_POINT('Ctrl Pts',(-41.7947768502118,37.621960399797,38.6613032467549));
#30404=CARTESIAN_POINT('Ctrl Pts',(-41.8128211743291,37.6469973293907,38.6777607539682));
#30405=CARTESIAN_POINT('Ctrl Pts',(-41.8308654984464,37.6720342589844,38.6942182611814));
#30406=CARTESIAN_POINT('Ctrl Pts',(-41.8487309539755,37.6973268728927,38.7104829541389));
#30407=CARTESIAN_POINT('Ctrl Pts',(-41.8664136129311,37.7228696120156,38.7265512573074));
#30408=CARTESIAN_POINT('Ctrl Pts',(-41.8840962718867,37.7484123511386,38.742619560476));
#30409=CARTESIAN_POINT('Ctrl Pts',(-41.9015961341555,37.7742052153137,38.7584914737537));
#30410=CARTESIAN_POINT('Ctrl Pts',(-41.9189093520144,37.8002425355872,38.7741635078405));
#30411=CARTESIAN_POINT('Ctrl Pts',(-41.9362225698734,37.8262798558608,38.7898355419273));
#30412=CARTESIAN_POINT('Ctrl Pts',(-41.953349143217,37.8525616320841,38.8053076967389));
#30413=CARTESIAN_POINT('Ctrl Pts',(-41.9702853062599,37.8790820878963,38.8205765707031));
#30414=CARTESIAN_POINT('Ctrl Pts',(-41.9872214693027,37.9056025437085,38.8358454446673));
#30415=CARTESIAN_POINT('Ctrl Pts',(-42.0039672219417,37.9323616789571,38.850911037702));
#30416=CARTESIAN_POINT('Ctrl Pts',(-42.0205188820049,37.9593536124801,38.8657700375203));
#30417=CARTESIAN_POINT('Ctrl Pts',(-42.0370705420681,37.9863455460031,38.8806290373385));
#30418=CARTESIAN_POINT('Ctrl Pts',(-42.053428109449,38.013570277627,38.8952814438449));
#30419=CARTESIAN_POINT('Ctrl Pts',(-42.069587987193,38.0410218239313,38.9097240354583));
#30420=CARTESIAN_POINT('Ctrl Pts',(-42.0857478649369,38.0684733702357,38.9241666270717));
#30421=CARTESIAN_POINT('Ctrl Pts',(-42.1017100529399,38.0961517310441,38.9383994036993));
#30422=CARTESIAN_POINT('Ctrl Pts',(-42.1174710410429,38.1240508233014,38.9524192358795));
#30423=CARTESIAN_POINT('Ctrl Pts',(-42.1332320291459,38.1519499155588,38.9664390680596));
#30424=CARTESIAN_POINT('Ctrl Pts',(-42.1487918172394,38.1800697390476,38.9802459556711));
#30425=CARTESIAN_POINT('Ctrl Pts',(-42.1641469835165,38.2084041138213,38.993836862806));
#30426=CARTESIAN_POINT('Ctrl Pts',(-42.1795021497936,38.2367384885949,39.0074277699409));
#30427=CARTESIAN_POINT('Ctrl Pts',(-42.1946526941551,38.2652874144759,39.0208026965141));
#30428=CARTESIAN_POINT('Ctrl Pts',(-42.2095952845997,38.294044617103,39.0339587013158));
#30429=CARTESIAN_POINT('Ctrl Pts',(-42.2245378750442,38.3228018197301,39.0471147061175));
#30430=CARTESIAN_POINT('Ctrl Pts',(-42.2392725114835,38.351767298959,39.0600517890953));
#30431=CARTESIAN_POINT('Ctrl Pts',(-42.2537959532316,38.3809346890054,39.0727671052191));
#30432=CARTESIAN_POINT('Ctrl Pts',(-42.2683193949798,38.4101020790518,39.085482421343));
#30433=CARTESIAN_POINT('Ctrl Pts',(-42.2826316419432,38.4394713797283,39.097975970531));
#30434=CARTESIAN_POINT('Ctrl Pts',(-42.2967295461582,38.4690361365363,39.110245005117));
#30435=CARTESIAN_POINT('Ctrl Pts',(-42.310839979782,38.4986271688047,39.1225249437173));
#30436=CARTESIAN_POINT('Ctrl Pts',(-42.3247356894058,38.5284140045892,39.1345799683876));
#30437=CARTESIAN_POINT('Ctrl Pts',(-42.3384136130202,38.558390086054,39.1464074229614));
#30438=CARTESIAN_POINT('Ctrl Pts',(-41.5196199854034,37.2918489624882,38.4265751654796));
#30439=CARTESIAN_POINT('Ctrl Pts',(-41.5397763593754,37.3147139246234,38.4453188414494));
#30440=CARTESIAN_POINT('Ctrl Pts',(-41.5597671768411,37.3378739508545,38.4638806099285));
#30441=CARTESIAN_POINT('Ctrl Pts',(-41.5795878307549,37.3613237037659,38.482256193207));
#30442=CARTESIAN_POINT('Ctrl Pts',(-41.5994084846687,37.3847734566774,38.5006317764855));
#30443=CARTESIAN_POINT('Ctrl Pts',(-41.6190589748855,37.4085129360958,38.5188211744265));
#30444=CARTESIAN_POINT('Ctrl Pts',(-41.6385347728,37.4325366710798,38.536820195149));
#30445=CARTESIAN_POINT('Ctrl Pts',(-41.6580105707144,37.4565604060638,38.5548192158715));
#30446=CARTESIAN_POINT('Ctrl Pts',(-41.677311676184,37.4808683964366,38.5726278592417));
#30447=CARTESIAN_POINT('Ctrl Pts',(-41.6964336411126,37.505455040225,38.5902420211136));
#30448=CARTESIAN_POINT('Ctrl Pts',(-41.7155556060412,37.5300416840132,38.6078561829855));
#30449=CARTESIAN_POINT('Ctrl Pts',(-41.7344984302935,37.554906981043,38.6252758632343));
#30450=CARTESIAN_POINT('Ctrl Pts',(-41.7532577483422,37.580045200905,38.6424970473537));
#30451=CARTESIAN_POINT('Ctrl Pts',(-41.7720170663908,37.6051834207671,38.659718231473));
#30452=CARTESIAN_POINT('Ctrl Pts',(-41.7905928781026,37.6305945632822,38.6767409193396));
#30453=CARTESIAN_POINT('Ctrl Pts',(-41.808980902532,37.6562727722492,38.6935611879397));
#30454=CARTESIAN_POINT('Ctrl Pts',(-41.8273689269614,37.6819509812161,38.7103814565398));
#30455=CARTESIAN_POINT('Ctrl Pts',(-41.8455691639783,37.7078962564534,38.7269993057545));
#30456=CARTESIAN_POINT('Ctrl Pts',(-41.8635774191899,37.7341026186593,38.743410905863));
#30457=CARTESIAN_POINT('Ctrl Pts',(-41.8815856744014,37.7603089808652,38.7598225059716));
#30458=CARTESIAN_POINT('Ctrl Pts',(-41.8994019476804,37.7867764298557,38.7760278568591));
#30459=CARTESIAN_POINT('Ctrl Pts',(-41.9170221331224,37.8134988659925,38.7920232238713));
#30460=CARTESIAN_POINT('Ctrl Pts',(-41.9346423185645,37.8402213021293,38.8080185908835));
#30461=CARTESIAN_POINT('Ctrl Pts',(-41.9520664160503,37.8671987252411,38.8238039739227));
#30462=CARTESIAN_POINT('Ctrl Pts',(-41.9692904100445,37.8944249181274,38.8393757350887));
#30463=CARTESIAN_POINT('Ctrl Pts',(-41.9865144040386,37.9216511110137,38.8549474962546));
#30464=CARTESIAN_POINT('Ctrl Pts',(-42.0035382944246,37.9491260734988,38.8703056354524));
#30465=CARTESIAN_POINT('Ctrl Pts',(-42.0203581579091,37.976843473755,38.8854466132742));
#30466=CARTESIAN_POINT('Ctrl Pts',(-42.0371780213936,38.0045608740113,38.900587591096));
#30467=CARTESIAN_POINT('Ctrl Pts',(-42.0537938578574,38.0325207118424,38.9155114074348));
#30468=CARTESIAN_POINT('Ctrl Pts',(-42.0702018380465,38.0607165436773,38.9302146229761));
#30469=CARTESIAN_POINT('Ctrl Pts',(-42.0866098182356,38.0889123755123,38.9449178385174));
#30470=CARTESIAN_POINT('Ctrl Pts',(-42.1028099420337,38.1173442011513,38.9594004531572));
#30471=CARTESIAN_POINT('Ctrl Pts',(-42.1187984759912,38.1460054682499,38.9736591292596));
#30472=CARTESIAN_POINT('Ctrl Pts',(-42.1347870099487,38.1746667353486,38.987917805362));
#30473=CARTESIAN_POINT('Ctrl Pts',(-42.150563953945,38.2035574436675,39.0019525427967));
#30474=CARTESIAN_POINT('Ctrl Pts',(-42.1661256720702,38.2326709351807,39.015760107203));
#30475=CARTESIAN_POINT('Ctrl Pts',(-42.1816873901954,38.2617844266939,39.0295676716092));
#30476=CARTESIAN_POINT('Ctrl Pts',(-42.197033882339,38.2911207011994,39.0431480628913));
#30477=CARTESIAN_POINT('Ctrl Pts',(-42.2121616117635,38.3206729978371,39.0564981512768));
#30478=CARTESIAN_POINT('Ctrl Pts',(-42.227289341188,38.3502252944748,39.0698482396623));
#30479=CARTESIAN_POINT('Ctrl Pts',(-42.2421983077933,38.379993613074,39.082968025087));
#30480=CARTESIAN_POINT('Ctrl Pts',(-42.2568850756873,38.4099710932844,39.0958544839902));
#30481=CARTESIAN_POINT('Ctrl Pts',(-42.2715718435813,38.4399485734949,39.1087409428933));
#30482=CARTESIAN_POINT('Ctrl Pts',(-42.2860364126601,38.4701352151043,39.1213940751837));
#30483=CARTESIAN_POINT('Ctrl Pts',(-42.3002754494465,38.5005240613567,39.1338109648444));
#30484=CARTESIAN_POINT('Ctrl Pts',(-42.3145271410722,38.5309399154729,39.1462388899246));
#30485=CARTESIAN_POINT('Ctrl Pts',(-42.3285528992461,38.561558333592,39.1584301521826));
#30486=CARTESIAN_POINT('Ctrl Pts',(-42.3423494858242,38.5923722469452,39.1703819369987));
#30487=CARTESIAN_POINT('Ctrl Pts',(-41.5003607592628,37.2929688677784,38.4459198005997));
#30488=CARTESIAN_POINT('Ctrl Pts',(-41.5213687291377,37.3168689568809,38.4655674622402));
#30489=CARTESIAN_POINT('Ctrl Pts',(-41.5421962007899,37.3410907400172,38.4850167989745));
#30490=CARTESIAN_POINT('Ctrl Pts',(-41.5628379586124,37.3656281534234,38.5042629425176));
#30491=CARTESIAN_POINT('Ctrl Pts',(-41.5834797164349,37.3901655668296,38.5235090860608));
#30492=CARTESIAN_POINT('Ctrl Pts',(-41.6039357602518,37.4150186102955,38.5425520362467));
#30493=CARTESIAN_POINT('Ctrl Pts',(-41.6242009671407,37.4401810625406,38.5613870262018));
#30494=CARTESIAN_POINT('Ctrl Pts',(-41.6444661740297,37.4653435147855,38.5802220161569));
#30495=CARTESIAN_POINT('Ctrl Pts',(-41.6645405438182,37.4908153755945,38.5988490457189));
#30496=CARTESIAN_POINT('Ctrl Pts',(-41.6844190488013,37.5165902692392,38.6172634517729));
#30497=CARTESIAN_POINT('Ctrl Pts',(-41.7042975537844,37.542365162884,38.6356778578269));
#30498=CARTESIAN_POINT('Ctrl Pts',(-41.7239801937969,37.5684430891506,38.65387964022));
#30499=CARTESIAN_POINT('Ctrl Pts',(-41.7434620388624,37.5948175210478,38.6718642419281));
#30500=CARTESIAN_POINT('Ctrl Pts',(-41.7629438839279,37.6211919529449,38.6898488436363));
#30501=CARTESIAN_POINT('Ctrl Pts',(-41.7822249338842,37.6478628902529,38.707616264509));
#30502=CARTESIAN_POINT('Ctrl Pts',(-41.8013003589378,37.6748236579662,38.7251620558827));
#30503=CARTESIAN_POINT('Ctrl Pts',(-41.8203757839915,37.7017844256796,38.7427078472564));
#30504=CARTESIAN_POINT('Ctrl Pts',(-41.839245583984,37.7290350235749,38.7600320089856));
#30505=CARTESIAN_POINT('Ctrl Pts',(-41.8579050317074,37.7565686319467,38.7771302029742));
#30506=CARTESIAN_POINT('Ctrl Pts',(-41.8765644794308,37.7841022403185,38.7942283969628));
#30507=CARTESIAN_POINT('Ctrl Pts',(-41.8950135747302,37.8119188589395,38.8111006230699));
#30508=CARTESIAN_POINT('Ctrl Pts',(-41.9132476953384,37.8400115268029,38.8277426559328));
#30509=CARTESIAN_POINT('Ctrl Pts',(-41.9314818159467,37.8681041946664,38.8443846887957));
#30510=CARTESIAN_POINT('Ctrl Pts',(-41.9495009617168,37.896472911555,38.8607965282903));
#30511=CARTESIAN_POINT('Ctrl Pts',(-41.9673006176136,37.9251105785895,38.8769740638598));
#30512=CARTESIAN_POINT('Ctrl Pts',(-41.9851002735103,37.953748245624,38.8931515994293));
#30513=CARTESIAN_POINT('Ctrl Pts',(-42.0026804393904,37.9826548625821,38.909094830953));
#30514=CARTESIAN_POINT('Ctrl Pts',(-42.0200367097175,38.0118231963049,38.924799764782));
#30515=CARTESIAN_POINT('Ctrl Pts',(-42.0373929800445,38.0409915300278,38.9405046986109));
#30516=CARTESIAN_POINT('Ctrl Pts',(-42.0545253546742,38.0704215802733,38.9559713346146));
#30517=CARTESIAN_POINT('Ctrl Pts',(-42.0714295397536,38.1001059831694,38.9711957980117));
#30518=CARTESIAN_POINT('Ctrl Pts',(-42.0883337248329,38.1297903860654,38.9864202614089));
#30519=CARTESIAN_POINT('Ctrl Pts',(-42.1050097202214,38.1597291413657,39.0014025520731));
#30520=CARTESIAN_POINT('Ctrl Pts',(-42.1214533458878,38.1899147581469,39.01613891602));
#30521=CARTESIAN_POINT('Ctrl Pts',(-42.1378969715542,38.2201003749281,39.0308752799669));
#30522=CARTESIAN_POINT('Ctrl Pts',(-42.1541082273559,38.2505328529074,39.0453657170479));
#30523=CARTESIAN_POINT('Ctrl Pts',(-42.1700830491774,38.2812045778996,39.0596065959968));
#30524=CARTESIAN_POINT('Ctrl Pts',(-42.1860578709989,38.3118763028919,39.0738474749456));
#30525=CARTESIAN_POINT('Ctrl Pts',(-42.2017962587068,38.3427872746465,39.0878387956457));
#30526=CARTESIAN_POINT('Ctrl Pts',(-42.2172942660912,38.3739297593054,39.1015770511987));
#30527=CARTESIAN_POINT('Ctrl Pts',(-42.2327922734756,38.4050722439644,39.1153153067518));
#30528=CARTESIAN_POINT('Ctrl Pts',(-42.2480499004129,38.4364462413039,39.1288004970705));
#30529=CARTESIAN_POINT('Ctrl Pts',(-42.2630633205988,38.4680439018423,39.1420292415324));
#30530=CARTESIAN_POINT('Ctrl Pts',(-42.2780767407846,38.4996415623808,39.1552579859942));
#30531=CARTESIAN_POINT('Ctrl Pts',(-42.2928459540939,38.5314628858563,39.168230284489));
#30532=CARTESIAN_POINT('Ctrl Pts',(-42.3073672560232,38.5634999109975,39.1809428842993));
#30533=CARTESIAN_POINT('Ctrl Pts',(-42.3219014636528,38.5955654088094,39.1936667823392));
#30534=CARTESIAN_POINT('Ctrl Pts',(-42.3361873189266,38.6278469915978,39.2061305197727));
#30535=CARTESIAN_POINT('Ctrl Pts',(-42.3502212314322,38.6603365687275,39.2183309650732));
#30536=CARTESIAN_POINT('Ctrl Pts',(-41.4810505382599,37.2940292410687,38.4652142825554));
#30537=CARTESIAN_POINT('Ctrl Pts',(-41.5028597677074,37.318904858524,38.4857150693105));
#30538=CARTESIAN_POINT('Ctrl Pts',(-41.5244734170253,37.3441290497964,38.506000959708));
#30539=CARTESIAN_POINT('Ctrl Pts',(-41.5458856178102,37.3696949679436,38.5260664478572));
#30540=CARTESIAN_POINT('Ctrl Pts',(-41.567297818595,37.395260886091,38.5461319360062));
#30541=CARTESIAN_POINT('Ctrl Pts',(-41.5885085706376,37.4211685308637,38.565977021711));
#30542=CARTESIAN_POINT('Ctrl Pts',(-41.6095121145511,37.4474108703597,38.5855963183546));
#30543=CARTESIAN_POINT('Ctrl Pts',(-41.6305156584647,37.4736532098558,38.6052156149982));
#30544=CARTESIAN_POINT('Ctrl Pts',(-41.651311994044,37.5002302438191,38.6246091223891));
#30545=CARTESIAN_POINT('Ctrl Pts',(-41.6718954740267,37.5271347591798,38.64377157609));
#30546=CARTESIAN_POINT('Ctrl Pts',(-41.6924789540094,37.5540392745403,38.6629340297909));
#30547=CARTESIAN_POINT('Ctrl Pts',(-41.7128495781944,37.5812712710359,38.6818654296146));
#30548=CARTESIAN_POINT('Ctrl Pts',(-41.7330018144911,37.6088233583184,38.7005606361427));
#30549=CARTESIAN_POINT('Ctrl Pts',(-41.7531540507878,37.6363754456009,38.7192558426709));
#30550=CARTESIAN_POINT('Ctrl Pts',(-41.7730878989981,37.6642476233992,38.7377148557188));
#30551=CARTESIAN_POINT('Ctrl Pts',(-41.7927979451909,37.6924323280774,38.7559326636636));
#30552=CARTESIAN_POINT('Ctrl Pts',(-41.8125079913837,37.7206170327555,38.7741504716083));
#30553=CARTESIAN_POINT('Ctrl Pts',(-41.8319942353652,37.7491142640362,38.7921270742699));
#30554=CARTESIAN_POINT('Ctrl Pts',(-41.8512513842813,37.7779162890641,38.8098575905164));
#30555=CARTESIAN_POINT('Ctrl Pts',(-41.8705085331973,37.8067183140921,38.8275881067629));
#30556=CARTESIAN_POINT('Ctrl Pts',(-41.8895365868606,37.8358251325889,38.8450725364234));
#30557=CARTESIAN_POINT('Ctrl Pts',(-41.9083303763512,37.8652288466486,38.8623061314902));
#30558=CARTESIAN_POINT('Ctrl Pts',(-41.9271241658417,37.8946325607082,38.879539726557));
#30559=CARTESIAN_POINT('Ctrl Pts',(-41.9456836909767,37.9243331700466,38.8965224868639));
#30560=CARTESIAN_POINT('Ctrl Pts',(-41.9640039095648,37.9543226159753,38.9132498000987));
#30561=CARTESIAN_POINT('Ctrl Pts',(-41.9823241281528,37.984312061904,38.9299771133336));
#30562=CARTESIAN_POINT('Ctrl Pts',(-42.0004050400183,38.0145903441468,38.9464489793472));
#30563=CARTESIAN_POINT('Ctrl Pts',(-42.0182417324114,38.0451492475406,38.9626609239792));
#30564=CARTESIAN_POINT('Ctrl Pts',(-42.0360784248044,38.0757081509344,38.9788728686112));
#30565=CARTESIAN_POINT('Ctrl Pts',(-42.0536708975543,38.1065476751967,38.9948248917171));
#30566=CARTESIAN_POINT('Ctrl Pts',(-42.0710143700199,38.1376594531819,39.01051265976));
#30567=CARTESIAN_POINT('Ctrl Pts',(-42.0883578424855,38.168771231167,39.026200427803));
#30568=CARTESIAN_POINT('Ctrl Pts',(-42.1054523144972,38.2001552625715,39.0416239406297));
#30569=CARTESIAN_POINT('Ctrl Pts',(-42.1222931400975,38.2318030327456,39.0567790076379));
#30570=CARTESIAN_POINT('Ctrl Pts',(-42.1391339656979,38.2634508029195,39.0719340746463));
#30571=CARTESIAN_POINT('Ctrl Pts',(-42.1557211447188,38.2953623115353,39.0868206956727));
#30572=CARTESIAN_POINT('Ctrl Pts',(-42.1720501684025,38.3275289010664,39.1014348253432));
#30573=CARTESIAN_POINT('Ctrl Pts',(-42.1883791920861,38.3596954905976,39.1160489550136));
#30574=CARTESIAN_POINT('Ctrl Pts',(-42.2044500602723,38.3921171607325,39.1303905931859));
#30575=CARTESIAN_POINT('Ctrl Pts',(-42.2202584038194,38.4247851156183,39.1444558418065));
#30576=CARTESIAN_POINT('Ctrl Pts',(-42.2360667473665,38.4574530705043,39.158521090427));
#30577=CARTESIAN_POINT('Ctrl Pts',(-42.2516125661229,38.4903673098427,39.1723099493739));
#30578=CARTESIAN_POINT('Ctrl Pts',(-42.2668916329426,38.5235189043152,39.185818670113));
#30579=CARTESIAN_POINT('Ctrl Pts',(-42.2821706997623,38.5566704987877,39.1993273908521));
#30580=CARTESIAN_POINT('Ctrl Pts',(-42.2971830144957,38.5900594480711,39.2125559732512));
#30581=CARTESIAN_POINT('Ctrl Pts',(-42.3119244942714,38.623676694153,39.2255008202899));
#30582=CARTESIAN_POINT('Ctrl Pts',(-42.326679075429,38.6573238173155,39.2384571719662));
#30583=CARTESIAN_POINT('Ctrl Pts',(-42.3411623398628,38.6911996428923,39.2511292835741));
#30584=CARTESIAN_POINT('Ctrl Pts',(-42.3553703406829,38.7252949646174,39.2635137024035));
#30585=CARTESIAN_POINT('Ctrl Pts',(-41.4617031412175,37.2950462146149,38.4844722020825));
#30586=CARTESIAN_POINT('Ctrl Pts',(-41.4842771920991,37.3208536029999,38.505788299774));
#30587=CARTESIAN_POINT('Ctrl Pts',(-41.5066404845182,37.3470366168299,38.5268728237077));
#30588=CARTESIAN_POINT('Ctrl Pts',(-41.5287864577224,37.3735875747549,38.5477195882852));
#30589=CARTESIAN_POINT('Ctrl Pts',(-41.5509324309266,37.4001385326801,38.5685663528626));
#30590=CARTESIAN_POINT('Ctrl Pts',(-41.5728610846616,37.4270574343957,38.5891753578446));
#30591=CARTESIAN_POINT('Ctrl Pts',(-41.5945659856856,37.4543363826632,38.6095405571367));
#30592=CARTESIAN_POINT('Ctrl Pts',(-41.6162708867097,37.4816153309308,38.6299057564287));
#30593=CARTESIAN_POINT('Ctrl Pts',(-41.6377520347735,37.5092543254373,38.650027149797));
#30594=CARTESIAN_POINT('Ctrl Pts',(-41.6590031279208,37.5372452576896,38.6698988341983));
#30595=CARTESIAN_POINT('Ctrl Pts',(-41.680254221068,37.5652361899419,38.6897705185996));
#30596=CARTESIAN_POINT('Ctrl Pts',(-41.7012752590547,37.5935790596188,38.7093924938059));
#30597=CARTESIAN_POINT('Ctrl Pts',(-41.7220600749075,37.6222655517302,38.7287590032889));
#30598=CARTESIAN_POINT('Ctrl Pts',(-41.7428448907603,37.6509520438417,38.7481255127719));
#30599=CARTESIAN_POINT('Ctrl Pts',(-41.7633934842396,37.6799821580562,38.7672365563075));
#30600=CARTESIAN_POINT('Ctrl Pts',(-41.783699826976,37.7093473777702,38.7860865272641));
#30601=CARTESIAN_POINT('Ctrl Pts',(-41.8040061697124,37.7387125974843,38.8049364982207));
#30602=CARTESIAN_POINT('Ctrl Pts',(-41.8240702614719,37.7684129223586,38.8235253963801));
#30603=CARTESIAN_POINT('Ctrl Pts',(-41.8438862160216,37.7984396391645,38.8418477682894));
#30604=CARTESIAN_POINT('Ctrl Pts',(-41.8637021705714,37.8284663559705,38.8601701401986));
#30605=CARTESIAN_POINT('Ctrl Pts',(-41.8832699876851,37.8588194643661,38.8782259856497));
#30606=CARTESIAN_POINT('Ctrl Pts',(-41.9025839267211,37.8894900596093,38.896010007568));
#30607=CARTESIAN_POINT('Ctrl Pts',(-41.921897865757,37.9201606548526,38.9137940294863));
#30608=CARTESIAN_POINT('Ctrl Pts',(-41.9409579264945,37.9511487365941,38.9313062276698));
#30609=CARTESIAN_POINT('Ctrl Pts',(-41.959758517255,37.9824452138141,38.9485414645386));
#30610=CARTESIAN_POINT('Ctrl Pts',(-41.9785591080156,38.013741691034,38.9657767014075));
#30611=CARTESIAN_POINT('Ctrl Pts',(-41.9971002285865,38.045346563388,38.9827349767773));
#30612=CARTESIAN_POINT('Ctrl Pts',(-42.0153764395253,38.0772505588784,38.9994113155473));
#30613=CARTESIAN_POINT('Ctrl Pts',(-42.0336526504642,38.1091545543687,39.0160876543173));
#30614=CARTESIAN_POINT('Ctrl Pts',(-42.0516639515643,38.1413576726435,39.0324820563089));
#30615=CARTESIAN_POINT('Ctrl Pts',(-42.0694050588234,38.1738504662258,39.048589711872));
#30616=CARTESIAN_POINT('Ctrl Pts',(-42.0871461660825,38.2063432598082,39.064697367435));
#30617=CARTESIAN_POINT('Ctrl Pts',(-42.104617079297,38.239125728325,39.0805182763847));
#30618=CARTESIAN_POINT('Ctrl Pts',(-42.1218126729988,38.2721882543348,39.0960477973172));
#30619=CARTESIAN_POINT('Ctrl Pts',(-42.1390082667007,38.3052507803445,39.1115773182498));
#30620=CARTESIAN_POINT('Ctrl Pts',(-42.1559285406899,38.33859336345,39.1268154509731));
#30621=CARTESIAN_POINT('Ctrl Pts',(-42.1725685310459,38.3722062219227,39.141757725081));
#30622=CARTESIAN_POINT('Ctrl Pts',(-42.189208521402,38.4058190803953,39.1566999991889));
#30623=CARTESIAN_POINT('Ctrl Pts',(-42.2055682279336,38.4397022138511,39.1713464145106));
#30624=CARTESIAN_POINT('Ctrl Pts',(-42.2216428511641,38.4738456819071,39.1856926741767));
#30625=CARTESIAN_POINT('Ctrl Pts',(-42.2377174743946,38.5079891499631,39.2000389338428));
#30626=CARTESIAN_POINT('Ctrl Pts',(-42.2535070141421,38.5423929522459,39.2140850377029));
#30627=CARTESIAN_POINT('Ctrl Pts',(-42.2690068382058,38.5770469956607,39.2278268650306));
#30628=CARTESIAN_POINT('Ctrl Pts',(-42.2845066622695,38.6117010390754,39.2415686923582));
#30629=CARTESIAN_POINT('Ctrl Pts',(-42.2997167704714,38.6466053232244,39.2550062429957));
#30630=CARTESIAN_POINT('Ctrl Pts',(-42.3146327005994,38.6817496081857,39.2681355747486));
#30631=CARTESIAN_POINT('Ctrl Pts',(-42.3295618871507,38.7169251273719,39.2812765750988));
#30632=CARTESIAN_POINT('Ctrl Pts',(-42.3441963723255,38.7523410737258,39.2941088082959));
#30633=CARTESIAN_POINT('Ctrl Pts',(-42.3585318550746,38.7879870388601,39.3066285029924));
#30634=CARTESIAN_POINT('Ctrl Pts',(-41.4423557441752,37.2960631881612,38.5037301216096));
#30635=CARTESIAN_POINT('Ctrl Pts',(-41.4656946164909,37.3228023474757,38.5258615302376));
#30636=CARTESIAN_POINT('Ctrl Pts',(-41.4888075520112,37.3499441838633,38.5477446877073));
#30637=CARTESIAN_POINT('Ctrl Pts',(-41.5116872976347,37.3774801815662,38.5693727287131));
#30638=CARTESIAN_POINT('Ctrl Pts',(-41.5345670432582,37.4050161792692,38.591000769719));
#30639=CARTESIAN_POINT('Ctrl Pts',(-41.5572135986857,37.4329463379276,38.6123736939783));
#30640=CARTESIAN_POINT('Ctrl Pts',(-41.5796198568202,37.4612618949667,38.6334847959188));
#30641=CARTESIAN_POINT('Ctrl Pts',(-41.6020261149547,37.4895774520057,38.6545958978593));
#30642=CARTESIAN_POINT('Ctrl Pts',(-41.6241920755031,37.5182784070554,38.6754451772049));
#30643=CARTESIAN_POINT('Ctrl Pts',(-41.6461107818148,37.5473557561995,38.6960260923066));
#30644=CARTESIAN_POINT('Ctrl Pts',(-41.6680294881265,37.5764331053434,38.7166070074083));
#30645=CARTESIAN_POINT('Ctrl Pts',(-41.6897009399149,37.6058868482017,38.7369195579971));
#30646=CARTESIAN_POINT('Ctrl Pts',(-41.7111183353238,37.6357077451421,38.756957370435));
#30647=CARTESIAN_POINT('Ctrl Pts',(-41.7325357307328,37.6655286420825,38.776995182873));
#30648=CARTESIAN_POINT('Ctrl Pts',(-41.7536990694811,37.6957166927132,38.7967582568962));
#30649=CARTESIAN_POINT('Ctrl Pts',(-41.7746017087611,37.7262624274631,38.8162403908647));
#30650=CARTESIAN_POINT('Ctrl Pts',(-41.7955043480412,37.756808162213,38.8357225248331));
#30651=CARTESIAN_POINT('Ctrl Pts',(-41.8161462875785,37.7877115806809,38.8549237184903));
#30652=CARTESIAN_POINT('Ctrl Pts',(-41.836521047762,37.818962989265,38.8738379460623));
#30653=CARTESIAN_POINT('Ctrl Pts',(-41.8568958079455,37.850214397849,38.8927521736344));
#30654=CARTESIAN_POINT('Ctrl Pts',(-41.8770033885096,37.8818137961431,38.9113794348761));
#30655=CARTESIAN_POINT('Ctrl Pts',(-41.896837477091,37.91375127257,38.9297138836458));
#30656=CARTESIAN_POINT('Ctrl Pts',(-41.9166715656723,37.9456887489969,38.9480483324156));
#30657=CARTESIAN_POINT('Ctrl Pts',(-41.9362321620123,37.9779643031416,38.9660899684756));
#30658=CARTESIAN_POINT('Ctrl Pts',(-41.9555131249453,38.0105678116528,38.9838331289786));
#30659=CARTESIAN_POINT('Ctrl Pts',(-41.9747940878784,38.0431713201639,39.0015762894816));
#30660=CARTESIAN_POINT('Ctrl Pts',(-41.9937954171547,38.0761027826293,39.0190209742075));
#30661=CARTESIAN_POINT('Ctrl Pts',(-42.0125111466393,38.1093518702162,39.0361617071154));
#30662=CARTESIAN_POINT('Ctrl Pts',(-42.0312268761239,38.1426009578031,39.0533024400233));
#30663=CARTESIAN_POINT('Ctrl Pts',(-42.0496570055743,38.1761676700903,39.0701392209007));
#30664=CARTESIAN_POINT('Ctrl Pts',(-42.0677957476269,38.2100414792698,39.0866667639839));
#30665=CARTESIAN_POINT('Ctrl Pts',(-42.0859344896795,38.2439152884493,39.103194307067));
#30666=CARTESIAN_POINT('Ctrl Pts',(-42.1037818440966,38.2780961940786,39.1194126121397));
#30667=CARTESIAN_POINT('Ctrl Pts',(-42.1213322059,38.3125734759241,39.1353165869965));
#30668=CARTESIAN_POINT('Ctrl Pts',(-42.1388825677034,38.3470507577696,39.1512205618533));
#30669=CARTESIAN_POINT('Ctrl Pts',(-42.156135936661,38.3818244153648,39.1668102062735));
#30670=CARTESIAN_POINT('Ctrl Pts',(-42.1730868936895,38.4168835427789,39.1820806248188));
#30671=CARTESIAN_POINT('Ctrl Pts',(-42.1900378507179,38.451942670193,39.1973510433641));
#30672=CARTESIAN_POINT('Ctrl Pts',(-42.2066863955949,38.4872872669698,39.2123022358353));
#30673=CARTESIAN_POINT('Ctrl Pts',(-42.2230272985088,38.5229062481958,39.226929506547));
#30674=CARTESIAN_POINT('Ctrl Pts',(-42.2393682014227,38.5585252294219,39.2415567772586));
#30675=CARTESIAN_POINT('Ctrl Pts',(-42.2554014621614,38.594418594649,39.255860126032));
#30676=CARTESIAN_POINT('Ctrl Pts',(-42.2711220434691,38.6305750870061,39.2698350599482));
#30677=CARTESIAN_POINT('Ctrl Pts',(-42.2868426247767,38.6667315793631,39.2838099938643));
#30678=CARTESIAN_POINT('Ctrl Pts',(-42.3022505264471,38.7031511983778,39.2974565127401));
#30679=CARTESIAN_POINT('Ctrl Pts',(-42.3173409069274,38.7398225222183,39.3107703292074));
#30680=CARTESIAN_POINT('Ctrl Pts',(-42.3324446988724,38.7765264374284,39.3240959782312));
#30681=CARTESIAN_POINT('Ctrl Pts',(-42.3472304047882,38.8134825045594,39.3370883330176));
#30682=CARTESIAN_POINT('Ctrl Pts',(-42.3616933694662,38.8506791131029,39.3497433035812));
#30683=CARTESIAN_POINT('Ctrl Pts',(-41.4229709680434,37.2970365249204,38.5229512790095));
#30684=CARTESIAN_POINT('Ctrl Pts',(-41.4470380178747,37.3246634845394,38.5458600258535));
#30685=CARTESIAN_POINT('Ctrl Pts',(-41.4708638548674,37.3527203469931,38.5685037367787));
#30686=CARTESIAN_POINT('Ctrl Pts',(-41.4944404939676,37.3811977108283,38.5908748246234));
#30687=CARTESIAN_POINT('Ctrl Pts',(-41.5180171330677,37.4096750746636,38.6132459124681));
#30688=CARTESIAN_POINT('Ctrl Pts',(-41.5413445739236,37.438572939456,38.6353443768986));
#30689=CARTESIAN_POINT('Ctrl Pts',(-41.564414998132,37.4678816225096,38.6571628130699));
#30690=CARTESIAN_POINT('Ctrl Pts',(-41.5874854223405,37.4971903055632,38.6789812492413));
#30691=CARTESIAN_POINT('Ctrl Pts',(-41.6102988295575,37.5269098064413,38.7005196568283));
#30692=CARTESIAN_POINT('Ctrl Pts',(-41.6328475732494,37.5570301676657,38.7217708182439));
#30693=CARTESIAN_POINT('Ctrl Pts',(-41.6553963169414,37.5871505288901,38.7430219796596));
#30694=CARTESIAN_POINT('Ctrl Pts',(-41.677680396772,37.617671750012,38.7639858945871));
#30695=CARTESIAN_POINT('Ctrl Pts',(-41.6996923431815,37.648583605415,38.7846555375145));
#30696=CARTESIAN_POINT('Ctrl Pts',(-41.7217042895911,37.6794954608179,38.8053251804419));
#30697=CARTESIAN_POINT('Ctrl Pts',(-41.743444102251,37.7107979500415,38.8257005510608));
#30698=CARTESIAN_POINT('Ctrl Pts',(-41.7649044935619,37.7424805861532,38.8457748206228));
#30699=CARTESIAN_POINT('Ctrl Pts',(-41.7863648848728,37.7741632222648,38.8658490901848));
#30700=CARTESIAN_POINT('Ctrl Pts',(-41.8075458545143,37.8062260047926,38.8856222583904));
#30701=CARTESIAN_POINT('Ctrl Pts',(-41.828440301712,37.8386581924846,38.9050876978125));
#30702=CARTESIAN_POINT('Ctrl Pts',(-41.8493347489098,37.8710903801766,38.9245531372346));
#30703=CARTESIAN_POINT('Ctrl Pts',(-41.869942673352,37.9038919725495,38.9437108475828));
#30704=CARTESIAN_POINT('Ctrl Pts',(-41.8902571658307,37.9370519811976,38.962554407175));
#30705=CARTESIAN_POINT('Ctrl Pts',(-41.9105716583094,37.9702119898458,38.9813979667672));
#30706=CARTESIAN_POINT('Ctrl Pts',(-41.9305927185212,38.0037304142752,38.9999273753223));
#30707=CARTESIAN_POINT('Ctrl Pts',(-41.9503136334377,38.0375960262564,39.0181364211902));
#30708=CARTESIAN_POINT('Ctrl Pts',(-41.9700345483543,38.0714616382376,39.0363454670581));
#30709=CARTESIAN_POINT('Ctrl Pts',(-41.9894553176812,38.1056744372663,39.0542341499672));
#30710=CARTESIAN_POINT('Ctrl Pts',(-42.0085694290524,38.1402229627798,39.0717964724463));
#30711=CARTESIAN_POINT('Ctrl Pts',(-42.0276835404236,38.1747714882931,39.0893587949255));
#30712=CARTESIAN_POINT('Ctrl Pts',(-42.0464909935538,38.2096557397765,39.1065947567127));
#30713=CARTESIAN_POINT('Ctrl Pts',(-42.0649854810888,38.2448640319788,39.1234985785208));
#30714=CARTESIAN_POINT('Ctrl Pts',(-42.0834799686239,38.2800723241811,39.1404024003288));
#30715=CARTESIAN_POINT('Ctrl Pts',(-42.1016614902876,38.3156046565778,39.1569740819053));
#30716=CARTESIAN_POINT('Ctrl Pts',(-42.1195239479505,38.3514491270237,39.1732080660062));
#30717=CARTESIAN_POINT('Ctrl Pts',(-42.1373864056134,38.3872935974697,39.189442050107));
#30718=CARTESIAN_POINT('Ctrl Pts',(-42.1549297990088,38.4234502054309,39.2053383364899));
#30719=CARTESIAN_POINT('Ctrl Pts',(-42.1721482433057,38.4599068398074,39.2208915936653));
#30720=CARTESIAN_POINT('Ctrl Pts',(-42.1893666876025,38.496363474184,39.2364448508407));
#30721=CARTESIAN_POINT('Ctrl Pts',(-42.2062601825436,38.5331201344327,39.2516550785763));
#30722=CARTESIAN_POINT('Ctrl Pts',(-42.222823060528,38.5701645085773,39.266517174699));
#30723=CARTESIAN_POINT('Ctrl Pts',(-42.2393859385125,38.6072088827218,39.2813792708218));
#30724=CARTESIAN_POINT('Ctrl Pts',(-42.2556181992928,38.6445409702104,39.2958932351096));
#30725=CARTESIAN_POINT('Ctrl Pts',(-42.2715143962856,38.6821482664024,39.3100541981141));
#30726=CARTESIAN_POINT('Ctrl Pts',(-42.2874105932784,38.7197555625943,39.3242151611187));
#30727=CARTESIAN_POINT('Ctrl Pts',(-42.3029707262459,38.7576380669294,39.3380231226285));
#30728=CARTESIAN_POINT('Ctrl Pts',(-42.3181895732623,38.7957830904435,39.3514734491742));
#30729=CARTESIAN_POINT('Ctrl Pts',(-42.3334219459173,38.833962015067,39.3649357295989));
#30730=CARTESIAN_POINT('Ctrl Pts',(-42.3483124254927,38.8724039251315,39.3780397388846));
#30731=CARTESIAN_POINT('Ctrl Pts',(-42.3628560048845,38.9110959214823,39.3907810709114));
#30732=CARTESIAN_POINT('Ctrl Pts',(-41.4035576403252,37.2979765302231,38.5421443560826));
#30733=CARTESIAN_POINT('Ctrl Pts',(-41.428325003475,37.3264575328628,38.565801044497));
#30734=CARTESIAN_POINT('Ctrl Pts',(-41.4528358013829,37.3553958001794,38.5891758283308));
#30735=CARTESIAN_POINT('Ctrl Pts',(-41.4770812806816,37.3847809976551,38.6122603599134));
#30736=CARTESIAN_POINT('Ctrl Pts',(-41.5013267599803,37.4141661951307,38.6353448914959));
#30737=CARTESIAN_POINT('Ctrl Pts',(-41.5253069202575,37.4439983222656,38.6581391704346));
#30738=CARTESIAN_POINT('Ctrl Pts',(-41.5490131976487,37.4742667253239,38.6806350563704));
#30739=CARTESIAN_POINT('Ctrl Pts',(-41.5727194750401,37.5045351283822,38.7031309423063));
#30740=CARTESIAN_POINT('Ctrl Pts',(-41.5961518691422,37.5352398068492,38.7253284348567));
#30741=CARTESIAN_POINT('Ctrl Pts',(-41.6193020117108,37.566369795381,38.7472196067887));
#30742=CARTESIAN_POINT('Ctrl Pts',(-41.6424521542793,37.5974997839129,38.7691107787207));
#30743=CARTESIAN_POINT('Ctrl Pts',(-41.6653200449205,37.6290550819801,38.790695629662));
#30744=CARTESIAN_POINT('Ctrl Pts',(-41.6878975169869,37.6610244204632,38.811966451168));
#30745=CARTESIAN_POINT('Ctrl Pts',(-41.7104749890533,37.6929937589462,38.833237272674));
#30746=CARTESIAN_POINT('Ctrl Pts',(-41.7327620421608,37.7253771373014,38.854194064383));
#30747=CARTESIAN_POINT('Ctrl Pts',(-41.7547507170926,37.7581629906826,38.8748293421447));
#30748=CARTESIAN_POINT('Ctrl Pts',(-41.7767393920243,37.7909488440638,38.8954646199064));
#30749=CARTESIAN_POINT('Ctrl Pts',(-41.7984296884063,37.8241371719135,38.9157783833699));
#30750=CARTESIAN_POINT('Ctrl Pts',(-41.8198138601368,37.8577161219199,38.9357633780249));
#30751=CARTESIAN_POINT('Ctrl Pts',(-41.8411980318674,37.8912950719261,38.95574837268));
#30752=CARTESIAN_POINT('Ctrl Pts',(-41.8622760785829,37.925264643518,38.9754045981869));
#30753=CARTESIAN_POINT('Ctrl Pts',(-41.8830404728302,37.9596127053833,38.9947250348572));
#30754=CARTESIAN_POINT('Ctrl Pts',(-41.9038048670775,37.9939607672486,39.0140454715275));
#30755=CARTESIAN_POINT('Ctrl Pts',(-41.9242556085034,38.0286873188033,39.0330301190327));
#30756=CARTESIAN_POINT('Ctrl Pts',(-41.9443853936797,38.0637799584006,39.0516721975204));
#30757=CARTESIAN_POINT('Ctrl Pts',(-41.9645151788561,38.0988725979979,39.0703142760081));
#30758=CARTESIAN_POINT('Ctrl Pts',(-41.9843240074406,38.1343313250409,39.0886137851613));
#30759=CARTESIAN_POINT('Ctrl Pts',(-42.003804805247,38.1701434764062,39.1065641898061));
#30760=CARTESIAN_POINT('Ctrl Pts',(-42.0232856030534,38.2059556277714,39.1245145944509));
#30761=CARTESIAN_POINT('Ctrl Pts',(-42.0424383697503,38.2421212028499,39.142115894282));
#30762=CARTESIAN_POINT('Ctrl Pts',(-42.0612562654461,38.2786272860865,39.1593618034723));
#30763=CARTESIAN_POINT('Ctrl Pts',(-42.0800741611419,38.315133369323,39.1766077126626));
#30764=CARTESIAN_POINT('Ctrl Pts',(-42.0985571855166,38.3519799600968,39.1934982309186));
#30765=CARTESIAN_POINT('Ctrl Pts',(-42.1166987378588,38.3891538996466,39.2100273262496));
#30766=CARTESIAN_POINT('Ctrl Pts',(-42.1348402902011,38.4263278391962,39.2265564215806));
#30767=CARTESIAN_POINT('Ctrl Pts',(-42.1526403702024,38.4638291268896,39.2427240937055));
#30768=CARTESIAN_POINT('Ctrl Pts',(-42.1700926210466,38.5016443701579,39.2585245687782));
#30769=CARTESIAN_POINT('Ctrl Pts',(-42.1875448718908,38.5394596134262,39.2743250438509));
#30770=CARTESIAN_POINT('Ctrl Pts',(-42.204649293281,38.5775888116264,39.2897583216026));
#30771=CARTESIAN_POINT('Ctrl Pts',(-42.2213997768367,38.6160183479486,39.3048188904566));
#30772=CARTESIAN_POINT('Ctrl Pts',(-42.2381502603923,38.6544478842708,39.3198794593106));
#30773=CARTESIAN_POINT('Ctrl Pts',(-42.2545468058286,38.6931777580614,39.3345673190107));
#30774=CARTESIAN_POINT('Ctrl Pts',(-42.2705835575636,38.7321941379955,39.3488772241858));
#30775=CARTESIAN_POINT('Ctrl Pts',(-42.2866203092985,38.7712105179296,39.3631871293609));
#30776=CARTESIAN_POINT('Ctrl Pts',(-42.3022972670594,38.8105134033437,39.3771190797676));
#30777=CARTESIAN_POINT('Ctrl Pts',(-42.3176088322457,38.8500887582774,39.3906680999874));
#30778=CARTESIAN_POINT('Ctrl Pts',(-42.332934005473,38.8896992855169,39.4042291617993));
#30779=CARTESIAN_POINT('Ctrl Pts',(-42.3478931360962,38.9295827661274,39.4174066122383));
#30780=CARTESIAN_POINT('Ctrl Pts',(-42.3624808722509,38.9697249315629,39.4301957368445));
#30781=CARTESIAN_POINT('Ctrl Pts',(-41.3841443126071,37.2989165355258,38.5613374331557));
#30782=CARTESIAN_POINT('Ctrl Pts',(-41.4096119890754,37.3282515811861,38.5857420631406));
#30783=CARTESIAN_POINT('Ctrl Pts',(-41.4348077478983,37.3580712533658,38.6098479198828));
#30784=CARTESIAN_POINT('Ctrl Pts',(-41.4597220673956,37.3883642844818,38.6336458952033));
#30785=CARTESIAN_POINT('Ctrl Pts',(-41.4846363868929,37.4186573155978,38.6574438705238));
#30786=CARTESIAN_POINT('Ctrl Pts',(-41.5092692665914,37.4494237050751,38.6809339639707));
#30787=CARTESIAN_POINT('Ctrl Pts',(-41.5336113971655,37.4806518281381,38.704107299671));
#30788=CARTESIAN_POINT('Ctrl Pts',(-41.5579535277396,37.5118799512011,38.7272806353713));
#30789=CARTESIAN_POINT('Ctrl Pts',(-41.582004908727,37.5435698072571,38.7501372128852));
#30790=CARTESIAN_POINT('Ctrl Pts',(-41.6057564501721,37.5757094230964,38.7726683953334));
#30791=CARTESIAN_POINT('Ctrl Pts',(-41.6295079916173,37.6078490389357,38.7951995777818));
#30792=CARTESIAN_POINT('Ctrl Pts',(-41.652959693069,37.6404384139483,38.8174053647368));
#30793=CARTESIAN_POINT('Ctrl Pts',(-41.6761026907923,37.6734652355113,38.8392773648215));
#30794=CARTESIAN_POINT('Ctrl Pts',(-41.6992456885155,37.7064920570744,38.8611493649062));
#30795=CARTESIAN_POINT('Ctrl Pts',(-41.7220799820707,37.7399563245612,38.8826875777052));
#30796=CARTESIAN_POINT('Ctrl Pts',(-41.7445969406233,37.7738453952121,38.9038838636666));
#30797=CARTESIAN_POINT('Ctrl Pts',(-41.7671138991759,37.8077344658628,38.925080149628));
#30798=CARTESIAN_POINT('Ctrl Pts',(-41.7893135222983,37.8420483390345,38.9459345083493));
#30799=CARTESIAN_POINT('Ctrl Pts',(-41.8111874185617,37.8767740513551,38.9664390582374));
#30800=CARTESIAN_POINT('Ctrl Pts',(-41.833061314825,37.9114997636757,38.9869436081255));
#30801=CARTESIAN_POINT('Ctrl Pts',(-41.8546094838138,37.9466373144864,39.0070983487909));
#30802=CARTESIAN_POINT('Ctrl Pts',(-41.8758237798296,37.9821734295689,39.0268956625394));
#30803=CARTESIAN_POINT('Ctrl Pts',(-41.8970380758455,38.0177095446515,39.0466929762878));
#30804=CARTESIAN_POINT('Ctrl Pts',(-41.9179184984855,38.0536442233315,39.0661328627431));
#30805=CARTESIAN_POINT('Ctrl Pts',(-41.9384571539217,38.0899638905448,39.0852079738506));
#30806=CARTESIAN_POINT('Ctrl Pts',(-41.9589958093579,38.1262835577581,39.1042830849581));
#30807=CARTESIAN_POINT('Ctrl Pts',(-41.9791926972001,38.1629882128155,39.1229934203554));
#30808=CARTESIAN_POINT('Ctrl Pts',(-41.9990401814417,38.2000639900327,39.1413319071658));
#30809=CARTESIAN_POINT('Ctrl Pts',(-42.0188876656832,38.2371397672498,39.1596703939762));
#30810=CARTESIAN_POINT('Ctrl Pts',(-42.0383857459468,38.2745866659233,39.1776370318513));
#30811=CARTESIAN_POINT('Ctrl Pts',(-42.0575270498033,38.3123905401941,39.1952250284238));
#30812=CARTESIAN_POINT('Ctrl Pts',(-42.0766683536599,38.350194414465,39.2128130249963));
#30813=CARTESIAN_POINT('Ctrl Pts',(-42.0954528807456,38.3883552636159,39.2300223799319));
#30814=CARTESIAN_POINT('Ctrl Pts',(-42.1138735277671,38.4268586722694,39.2468465864931));
#30815=CARTESIAN_POINT('Ctrl Pts',(-42.1322941747887,38.4653620809229,39.2636707930542));
#30816=CARTESIAN_POINT('Ctrl Pts',(-42.150350941396,38.5042080483483,39.2801098509211));
#30817=CARTESIAN_POINT('Ctrl Pts',(-42.1680369987875,38.5433819005085,39.296157543891));
#30818=CARTESIAN_POINT('Ctrl Pts',(-42.1857230561791,38.5825557526686,39.312205236861));
#30819=CARTESIAN_POINT('Ctrl Pts',(-42.2030384040184,38.6220574888201,39.3278615646289));
#30820=CARTESIAN_POINT('Ctrl Pts',(-42.2199764931453,38.6618721873199,39.3431206062142));
#30821=CARTESIAN_POINT('Ctrl Pts',(-42.2369145822722,38.7016868858197,39.3583796477995));
#30822=CARTESIAN_POINT('Ctrl Pts',(-42.2534754123644,38.7418145459123,39.3732414029119));
#30823=CARTESIAN_POINT('Ctrl Pts',(-42.2696527188415,38.7822400095886,39.3877002502575));
#30824=CARTESIAN_POINT('Ctrl Pts',(-42.2858300253186,38.8226654732649,39.402159097603));
#30825=CARTESIAN_POINT('Ctrl Pts',(-42.3016238078729,38.863388739758,39.4162150369067));
#30826=CARTESIAN_POINT('Ctrl Pts',(-42.317028091229,38.9043944261112,39.4298627508005));
#30827=CARTESIAN_POINT('Ctrl Pts',(-42.3324460650287,38.9454365559668,39.4435225939999));
#30828=CARTESIAN_POINT('Ctrl Pts',(-42.3474738466997,38.9867616071232,39.4567734855919));
#30829=CARTESIAN_POINT('Ctrl Pts',(-42.3621057396173,39.0283539416435,39.4696104027777));
#30830=CARTESIAN_POINT('Ctrl Pts',(-41.3647023344627,37.2998230939851,38.5805023326933));
#30831=CARTESIAN_POINT('Ctrl Pts',(-41.3908423574775,37.3299783140399,38.6056254203547));
#30832=CARTESIAN_POINT('Ctrl Pts',(-41.4166950335924,37.3606456594132,38.6304327816703));
#30833=CARTESIAN_POINT('Ctrl Pts',(-41.4422500364264,37.3918128820555,38.6549145092738));
#30834=CARTESIAN_POINT('Ctrl Pts',(-41.4678050392604,37.4229801046978,38.6793962368773));
#30835=CARTESIAN_POINT('Ctrl Pts',(-41.4930623682715,37.4546472039489,38.7035523302504));
#30836=CARTESIAN_POINT('Ctrl Pts',(-41.5180119344913,37.4868015330437,38.7273731417376));
#30837=CARTESIAN_POINT('Ctrl Pts',(-41.5429615007111,37.5189558621386,38.7511939532247));
#30838=CARTESIAN_POINT('Ctrl Pts',(-41.5676033036101,37.5515974203945,38.77467948232));
#30839=CARTESIAN_POINT('Ctrl Pts',(-41.5919274996662,37.5847131724031,38.797820348766));
#30840=CARTESIAN_POINT('Ctrl Pts',(-41.6162516957224,37.6178289244116,38.8209612152119));
#30841=CARTESIAN_POINT('Ctrl Pts',(-41.6402582844198,37.6514188694715,38.8437574185185));
#30842=CARTESIAN_POINT('Ctrl Pts',(-41.6639376755246,37.6854695939044,38.8661998532878));
#30843=CARTESIAN_POINT('Ctrl Pts',(-41.6876170666294,37.7195203183375,38.888642288057));
#30844=CARTESIAN_POINT('Ctrl Pts',(-41.7109692596392,37.7540318214229,38.9107309538146));
#30845=CARTESIAN_POINT('Ctrl Pts',(-41.7339849252473,37.7889903219007,38.9324570272832));
#30846=CARTESIAN_POINT('Ctrl Pts',(-41.7570005908553,37.8239488223784,38.9541831007517));
#30847=CARTESIAN_POINT('Ctrl Pts',(-41.7796797285733,37.8593543195073,38.9755465814704));
#30848=CARTESIAN_POINT('Ctrl Pts',(-41.8020132774537,37.8951926754153,38.9965389353068));
#30849=CARTESIAN_POINT('Ctrl Pts',(-41.8243468263341,37.9310310313234,39.0175312891431));
#30850=CARTESIAN_POINT('Ctrl Pts',(-41.846334785903,37.9673022452508,39.0381525156518));
#30851=CARTESIAN_POINT('Ctrl Pts',(-41.8679683707908,38.0039918339702,39.0583943766432));
#30852=CARTESIAN_POINT('Ctrl Pts',(-41.8896019556786,38.0406814226895,39.0786362376347));
#30853=CARTESIAN_POINT('Ctrl Pts',(-41.910881165426,38.0777893854232,39.0984987326795));
#30854=CARTESIAN_POINT('Ctrl Pts',(-41.931797497241,38.1153009051195,39.1179739260933));
#30855=CARTESIAN_POINT('Ctrl Pts',(-41.9527138290561,38.1528124248159,39.1374491195071));
#30856=CARTESIAN_POINT('Ctrl Pts',(-41.973267282494,38.190727500674,39.1565370108716));
#30857=CARTESIAN_POINT('Ctrl Pts',(-41.9934496441163,38.2290309936264,39.1752299733406));
#30858=CARTESIAN_POINT('Ctrl Pts',(-42.0136320057387,38.2673344865787,39.1939229358096));
#30859=CARTESIAN_POINT('Ctrl Pts',(-42.0334432751162,38.3060263958077,39.2122209689812));
#30860=CARTESIAN_POINT('Ctrl Pts',(-42.0528755347069,38.34509127226,39.2301167609037));
#30861=CARTESIAN_POINT('Ctrl Pts',(-42.0723077942975,38.3841561487124,39.2480125528261));
#30862=CARTESIAN_POINT('Ctrl Pts',(-42.0913610436888,38.4235939915674,39.2655061031254));
#30863=CARTESIAN_POINT('Ctrl Pts',(-42.1100276675451,38.4633890540822,39.2825904205687));
#30864=CARTESIAN_POINT('Ctrl Pts',(-42.1286942914013,38.503184116597,39.2996747380119));
#30865=CARTESIAN_POINT('Ctrl Pts',(-42.146974289326,38.543336397925,39.316349822234));
#30866=CARTESIAN_POINT('Ctrl Pts',(-42.164860354262,38.583829866219,39.3326090083328));
#30867=CARTESIAN_POINT('Ctrl Pts',(-42.182746419198,38.6243233345131,39.3488681944315));
#30868=CARTESIAN_POINT('Ctrl Pts',(-42.200238550765,38.6651579889162,39.3647114820621));
#30869=CARTESIAN_POINT('Ctrl Pts',(-42.2173297560061,38.7063175251639,39.3801325379038));
#30870=CARTESIAN_POINT('Ctrl Pts',(-42.2344209612472,38.7474770614115,39.3955535937456));
#30871=CARTESIAN_POINT('Ctrl Pts',(-42.2511112397995,38.7889614786422,39.4105524174792));
#30872=CARTESIAN_POINT('Ctrl Pts',(-42.267393918383,38.8307542132177,39.4251230124646));
#30873=CARTESIAN_POINT('Ctrl Pts',(-42.2836765969667,38.8725469477931,39.43969360745));
#30874=CARTESIAN_POINT('Ctrl Pts',(-42.2995516752353,38.9146479988278,39.4538359733773));
#30875=CARTESIAN_POINT('Ctrl Pts',(-42.3150128049069,38.9570405564743,39.467544455051));
#30876=CARTESIAN_POINT('Ctrl Pts',(-42.3304876755439,38.9994707901951,39.481265120037));
#30877=CARTESIAN_POINT('Ctrl Pts',(-42.3455478611398,39.0421930480067,39.4945511289116));
#30878=CARTESIAN_POINT('Ctrl Pts',(-42.3601873274122,39.0851902417554,39.5073971582654));
#30879=CARTESIAN_POINT('Ctrl Pts',(-41.3452377207148,37.3007032273757,38.5996449702406));
#30880=CARTESIAN_POINT('Ctrl Pts',(-41.3720280192526,37.3316517033458,38.6254629394162));
#30881=CARTESIAN_POINT('Ctrl Pts',(-41.3985154762073,37.3631399200295,38.6509481572531));
#30882=CARTESIAN_POINT('Ctrl Pts',(-41.424688926481,37.3951546043889,38.6760898811217));
#30883=CARTESIAN_POINT('Ctrl Pts',(-41.4508623767548,37.4271692887483,38.7012316049902));
#30884=CARTESIAN_POINT('Ctrl Pts',(-41.4767218197276,37.4597104400256,38.7260298342954));
#30885=CARTESIAN_POINT('Ctrl Pts',(-41.502256355026,37.4927643413466,38.7504741159893));
#30886=CARTESIAN_POINT('Ctrl Pts',(-41.5277908903244,37.5258182426675,38.7749183976833));
#30887=CARTESIAN_POINT('Ctrl Pts',(-41.5530005173431,37.5593848932482,38.7990087311859));
#30888=CARTESIAN_POINT('Ctrl Pts',(-41.5778746096208,37.5934501439432,38.8227349618473));
#30889=CARTESIAN_POINT('Ctrl Pts',(-41.6027487018984,37.6275153946382,38.8464611925086));
#30890=CARTESIAN_POINT('Ctrl Pts',(-41.6272872588458,37.6620792446412,38.8698233197672));
#30891=CARTESIAN_POINT('Ctrl Pts',(-41.6514799368739,37.6971271244599,38.892811495924));
#30892=CARTESIAN_POINT('Ctrl Pts',(-41.675672614902,37.7321750042785,38.9157996720809));
#30893=CARTESIAN_POINT('Ctrl Pts',(-41.6995194134375,37.7677069130834,38.9384138965928));
#30894=CARTESIAN_POINT('Ctrl Pts',(-41.7230102804842,37.8037078733246,38.960644637023));
#30895=CARTESIAN_POINT('Ctrl Pts',(-41.7465011475309,37.8397088335659,38.9828753774532));
#30896=CARTESIAN_POINT('Ctrl Pts',(-41.7696360825321,37.8761788443904,39.0047226332749));
#30897=CARTESIAN_POINT('Ctrl Pts',(-41.792405333559,37.913102532816,39.0261771953468));
#30898=CARTESIAN_POINT('Ctrl Pts',(-41.815174584586,37.9500262212414,39.0476317574188));
#30899=CARTESIAN_POINT('Ctrl Pts',(-41.8375781510992,37.9874035863929,39.0686936252327));
#30900=CARTESIAN_POINT('Ctrl Pts',(-41.8596065894592,38.0252188728165,39.0893539207072));
#30901=CARTESIAN_POINT('Ctrl Pts',(-41.8816350278192,38.0630341592401,39.1100142161817));
#30902=CARTESIAN_POINT('Ctrl Pts',(-41.903288337504,38.1012873660397,39.1302729388273));
#30903=CARTESIAN_POINT('Ctrl Pts',(-41.9245573911254,38.1399623685732,39.1501215491074));
#30904=CARTESIAN_POINT('Ctrl Pts',(-41.9458264447468,38.1786373711068,39.1699701593876));
#30905=CARTESIAN_POINT('Ctrl Pts',(-41.9667112418003,38.2177341684525,39.1894086568271));
#30906=CARTESIAN_POINT('Ctrl Pts',(-41.9872029788452,38.257236280385,39.2084288476439));
#30907=CARTESIAN_POINT('Ctrl Pts',(-42.00769471589,38.2967383923175,39.2274490384606));
#30908=CARTESIAN_POINT('Ctrl Pts',(-42.0277933924401,38.3366458178957,39.2460509221991));
#30909=CARTESIAN_POINT('Ctrl Pts',(-42.0474905364223,38.3769417351846,39.2642266577201));
#30910=CARTESIAN_POINT('Ctrl Pts',(-42.0671876804046,38.4172376524736,39.2824023932411));
#30911=CARTESIAN_POINT('Ctrl Pts',(-42.0864832913524,38.4579220605255,39.3001519801198));
#30912=CARTESIAN_POINT('Ctrl Pts',(-42.1053692357035,38.498977809875,39.3174679364691));
#30913=CARTESIAN_POINT('Ctrl Pts',(-42.1242551800547,38.5400335592245,39.3347838928183));
#30914=CARTESIAN_POINT('Ctrl Pts',(-42.1427314573616,38.5814606488959,39.3516662182258));
#30915=CARTESIAN_POINT('Ctrl Pts',(-42.1607902794319,38.6232416163983,39.3681077964026));
#30916=CARTESIAN_POINT('Ctrl Pts',(-42.1788491015022,38.6650225839007,39.3845493745794));
#30917=CARTESIAN_POINT('Ctrl Pts',(-42.1964904679075,38.7071574282453,39.4005502051364));
#30918=CARTESIAN_POINT('Ctrl Pts',(-42.2137069423898,38.7496283885661,39.4161035433246));
#30919=CARTESIAN_POINT('Ctrl Pts',(-42.2309234168721,38.7920993488871,39.4316568815127));
#30920=CARTESIAN_POINT('Ctrl Pts',(-42.2477149990234,38.834906424188,39.4467627269715));
#30921=CARTESIAN_POINT('Ctrl Pts',(-42.2640746107899,38.8780315702624,39.4614147122255));
#30922=CARTESIAN_POINT('Ctrl Pts',(-42.2804342225564,38.9211567163368,39.4760666974795));
#30923=CARTESIAN_POINT('Ctrl Pts',(-42.2963618635506,38.9645999321627,39.4902648221815));
#30924=CARTESIAN_POINT('Ctrl Pts',(-42.3118508198906,39.008342905385,39.5040031014822));
#30925=CARTESIAN_POINT('Ctrl Pts',(-42.3273535419267,39.0521247548533,39.5177535905777));
#30926=CARTESIAN_POINT('Ctrl Pts',(-42.3424167988389,39.0962068937307,39.531043416214));
#30927=CARTESIAN_POINT('Ctrl Pts',(-42.3570342296479,39.1405707074102,39.5438669662772));
#30928=CARTESIAN_POINT('Ctrl Pts',(-41.325773106967,37.3015833607663,38.6187876077879));
#30929=CARTESIAN_POINT('Ctrl Pts',(-41.3532136810277,37.3333250926518,38.6453004584778));
#30930=CARTESIAN_POINT('Ctrl Pts',(-41.3803359188222,37.3656341806458,38.6714635328359));
#30931=CARTESIAN_POINT('Ctrl Pts',(-41.4071278165357,37.3984963267223,38.6972652529695));
#30932=CARTESIAN_POINT('Ctrl Pts',(-41.4339197142492,37.4313584727989,38.723066973103));
#30933=CARTESIAN_POINT('Ctrl Pts',(-41.4603812711837,37.4647736761024,38.7485073383404));
#30934=CARTESIAN_POINT('Ctrl Pts',(-41.4865007755607,37.4987271496494,38.7735750902411));
#30935=CARTESIAN_POINT('Ctrl Pts',(-41.5126202799377,37.5326806231965,38.7986428421418));
#30936=CARTESIAN_POINT('Ctrl Pts',(-41.5383977310762,37.5671723661017,38.8233379800519));
#30937=CARTESIAN_POINT('Ctrl Pts',(-41.5638217195754,37.6021871154832,38.8476495749286));
#30938=CARTESIAN_POINT('Ctrl Pts',(-41.5892457080746,37.6372018648648,38.8719611698053));
#30939=CARTESIAN_POINT('Ctrl Pts',(-41.6143162332718,37.6727396198109,38.8958892210159));
#30940=CARTESIAN_POINT('Ctrl Pts',(-41.6390221982231,37.7087846550152,38.9194231385604));
#30941=CARTESIAN_POINT('Ctrl Pts',(-41.6637281631745,37.7448296902195,38.9429570561048));
#30942=CARTESIAN_POINT('Ctrl Pts',(-41.6880695672358,37.7813820047439,38.966096839371));
#30943=CARTESIAN_POINT('Ctrl Pts',(-41.7120356357211,37.8184254247486,38.9888322467629));
#30944=CARTESIAN_POINT('Ctrl Pts',(-41.7360017042064,37.8554688447534,39.0115676541547));
#30945=CARTESIAN_POINT('Ctrl Pts',(-41.7595924364909,37.8930033692735,39.0338986850794));
#30946=CARTESIAN_POINT('Ctrl Pts',(-41.7827973896644,37.9310123902165,39.0558154553869));
#30947=CARTESIAN_POINT('Ctrl Pts',(-41.8060023428379,37.9690214111595,39.0777322256945));
#30948=CARTESIAN_POINT('Ctrl Pts',(-41.8288215162954,38.007504927535,39.0992347348136));
#30949=CARTESIAN_POINT('Ctrl Pts',(-41.8512448081276,38.0464459116628,39.1203134647711));
#30950=CARTESIAN_POINT('Ctrl Pts',(-41.8736680999599,38.0853868957906,39.1413921947287));
#30951=CARTESIAN_POINT('Ctrl Pts',(-41.895695509582,38.1247853466562,39.1620471449751));
#30952=CARTESIAN_POINT('Ctrl Pts',(-41.9173172850097,38.164623832027,39.1822691721216));
#30953=CARTESIAN_POINT('Ctrl Pts',(-41.9389390604375,38.2044623173978,39.202491199268));
#30954=CARTESIAN_POINT('Ctrl Pts',(-41.9601552011066,38.2447408362309,39.2222803027826));
#30955=CARTESIAN_POINT('Ctrl Pts',(-41.980956313574,38.2854415671435,39.2416277219471));
#30956=CARTESIAN_POINT('Ctrl Pts',(-42.0017574260413,38.3261422980563,39.2609751411116));
#30957=CARTESIAN_POINT('Ctrl Pts',(-42.0221435097639,38.3672652399837,39.2798808754169));
#30958=CARTESIAN_POINT('Ctrl Pts',(-42.0421055381378,38.4087921981093,39.2983365545365));
#30959=CARTESIAN_POINT('Ctrl Pts',(-42.0620675665116,38.450319156235,39.3167922336561));
#30960=CARTESIAN_POINT('Ctrl Pts',(-42.081605539016,38.4922501294836,39.3347978571142));
#30961=CARTESIAN_POINT('Ctrl Pts',(-42.100710803862,38.5345665656678,39.3523454523695));
#30962=CARTESIAN_POINT('Ctrl Pts',(-42.119816068708,38.5768830018521,39.3698930476248));
#30963=CARTESIAN_POINT('Ctrl Pts',(-42.1384886253973,38.6195848998668,39.3869826142177));
#30964=CARTESIAN_POINT('Ctrl Pts',(-42.1567202046019,38.6626533665775,39.4036065844725));
#30965=CARTESIAN_POINT('Ctrl Pts',(-42.1749517838064,38.7057218332882,39.4202305547273));
#30966=CARTESIAN_POINT('Ctrl Pts',(-42.1927423850501,38.7491568675743,39.4363889282107));
#30967=CARTESIAN_POINT('Ctrl Pts',(-42.2100841287736,38.7929392519684,39.4520745487453));
#30968=CARTESIAN_POINT('Ctrl Pts',(-42.2274258724969,38.8367216363625,39.4677601692799));
#30969=CARTESIAN_POINT('Ctrl Pts',(-42.2443187582472,38.8808513697338,39.4829730364638));
#30970=CARTESIAN_POINT('Ctrl Pts',(-42.2607553031968,38.925308927307,39.4977064119864));
#30971=CARTESIAN_POINT('Ctrl Pts',(-42.2771918481463,38.9697664848803,39.512439787509));
#30972=CARTESIAN_POINT('Ctrl Pts',(-42.2931720518659,39.0145518654976,39.5266936709857));
#30973=CARTESIAN_POINT('Ctrl Pts',(-42.3086888348743,39.0596452542956,39.5404617479134));
#30974=CARTESIAN_POINT('Ctrl Pts',(-42.3242194083095,39.1047787195115,39.5542420611184));
#30975=CARTESIAN_POINT('Ctrl Pts',(-42.339285736538,39.1502207394548,39.5675357035164));
#30976=CARTESIAN_POINT('Ctrl Pts',(-42.3538811318835,39.1959511730649,39.5803367742889));
#30977=CARTESIAN_POINT('Ctrl Pts',(-41.3062858049163,37.3024370075663,38.6379079315151));
#30978=CARTESIAN_POINT('Ctrl Pts',(-41.3343545286771,37.3349450157083,38.665092038194));
#30979=CARTESIAN_POINT('Ctrl Pts',(-41.3620893558469,37.3680481123285,38.6919092714245));
#30980=CARTESIAN_POINT('Ctrl Pts',(-41.389477409864,37.4017309298736,38.7183471819599));
#30981=CARTESIAN_POINT('Ctrl Pts',(-41.416865463881,37.4354137474188,38.7447850924952));
#30982=CARTESIAN_POINT('Ctrl Pts',(-41.4439067439596,37.469676284923,38.7708436795772));
#30983=CARTESIAN_POINT('Ctrl Pts',(-41.4705886951389,37.5045026371562,38.7965108457472));
#30984=CARTESIAN_POINT('Ctrl Pts',(-41.4972706463182,37.5393289893894,38.8221780119171));
#30985=CARTESIAN_POINT('Ctrl Pts',(-41.5235932678327,37.574719155353,38.8474537564389));
#30986=CARTESIAN_POINT('Ctrl Pts',(-41.5495443379544,37.6106567068741,38.8723263448488));
#30987=CARTESIAN_POINT('Ctrl Pts',(-41.5754954080762,37.6465942583951,38.8971989332587));
#30988=CARTESIAN_POINT('Ctrl Pts',(-41.6010749260608,37.6830791944433,38.9216683648434));
#30989=CARTESIAN_POINT('Ctrl Pts',(-41.6262710147375,37.7200945791203,38.9457232790054));
#30990=CARTESIAN_POINT('Ctrl Pts',(-41.6514671034143,37.7571099637973,38.9697781931674));
#30991=CARTESIAN_POINT('Ctrl Pts',(-41.6762797620602,37.794655796042,38.9934185892169));
#30992=CARTESIAN_POINT('Ctrl Pts',(-41.7006974690671,37.8327146479188,39.0166334909482));
#30993=CARTESIAN_POINT('Ctrl Pts',(-41.725115176074,37.8707734997956,39.0398483926795));
#30994=CARTESIAN_POINT('Ctrl Pts',(-41.7491379307412,37.9093453702133,39.0626377994268));
#30995=CARTESIAN_POINT('Ctrl Pts',(-41.7727545776992,37.9484123553418,39.0849911295462));
#30996=CARTESIAN_POINT('Ctrl Pts',(-41.7963712246572,37.9874793404703,39.1073444596656));
#30997=CARTESIAN_POINT('Ctrl Pts',(-41.8195817632284,38.0270414391895,39.1292617125159));
#30998=CARTESIAN_POINT('Ctrl Pts',(-41.8423754146195,38.0670802883583,39.1507327108198));
#30999=CARTESIAN_POINT('Ctrl Pts',(-41.8651690660106,38.107119137527,39.1722037091237));
#31000=CARTESIAN_POINT('Ctrl Pts',(-41.8875458295674,38.1476347359975,39.193228452265));
#31001=CARTESIAN_POINT('Ctrl Pts',(-41.9094953130622,38.1886082783258,39.213797176764));
#31002=CARTESIAN_POINT('Ctrl Pts',(-41.931444796557,38.2295818206541,39.2343659012629));
#31003=CARTESIAN_POINT('Ctrl Pts',(-41.9529669993598,38.2710133056656,39.2544786065292));
#31004=CARTESIAN_POINT('Ctrl Pts',(-41.9740519254398,38.3128835030316,39.274125951928));
#31005=CARTESIAN_POINT('Ctrl Pts',(-41.9951368515198,38.3547537003978,39.2937732973269));
#31006=CARTESIAN_POINT('Ctrl Pts',(-42.0157845002718,38.3970626089183,39.3129552822944));
#31007=CARTESIAN_POINT('Ctrl Pts',(-42.035985281127,38.439790591191,39.3316629976981));
#31008=CARTESIAN_POINT('Ctrl Pts',(-42.0561860619822,38.4825185734638,39.3503707131017));
#31009=CARTESIAN_POINT('Ctrl Pts',(-42.0759399743606,38.5256656282641,39.3686041584044));
#31010=CARTESIAN_POINT('Ctrl Pts',(-42.0952378420455,38.5692117293042,39.3863548642333));
#31011=CARTESIAN_POINT('Ctrl Pts',(-42.1145357097305,38.6127578303443,39.4041055700621));
#31012=CARTESIAN_POINT('Ctrl Pts',(-42.1333775321678,38.6567029763761,39.4213735359074));
#31013=CARTESIAN_POINT('Ctrl Pts',(-42.1517545559995,38.7010267707748,39.438150740007));
#31014=CARTESIAN_POINT('Ctrl Pts',(-42.1701315798312,38.7453505651734,39.4549279441066));
#31015=CARTESIAN_POINT('Ctrl Pts',(-42.1880438045295,38.7900530066685,39.4712143859786));
#31016=CARTESIAN_POINT('Ctrl Pts',(-42.2054829077106,38.8351133471886,39.487002498908));
#31017=CARTESIAN_POINT('Ctrl Pts',(-42.2229220108917,38.8801736877088,39.5027906118375));
#31018=CARTESIAN_POINT('Ctrl Pts',(-42.2398879920545,38.9255919259625,39.5180803953709));
#31019=CARTESIAN_POINT('Ctrl Pts',(-42.2563729675066,38.9713469816487,39.5328647448567));
#31020=CARTESIAN_POINT('Ctrl Pts',(-42.2728579429587,39.0171020373349,39.5476490943425));
#31021=CARTESIAN_POINT('Ctrl Pts',(-42.2888619122262,39.0631939091422,39.5619280093558));
#31022=CARTESIAN_POINT('Ctrl Pts',(-42.3043774376187,39.1096012040638,39.5756948538967));
#31023=CARTESIAN_POINT('Ctrl Pts',(-42.3199067523203,39.1560497431279,39.5894739336195));
#31024=CARTESIAN_POINT('Ctrl Pts',(-42.3349467541126,39.2028142648828,39.6027400318712));
#31025=CARTESIAN_POINT('Ctrl Pts',(-42.3494904395659,39.2498730255593,39.6154869710169));
#31026=CARTESIAN_POINT('Ctrl Pts',(-41.2867801198513,37.3032691938199,38.6570101756496));
#31027=CARTESIAN_POINT('Ctrl Pts',(-41.3154590259865,37.3365214462081,38.6848461534539));
#31028=CARTESIAN_POINT('Ctrl Pts',(-41.3437884160841,37.3703966248004,38.7122980957319));
#31029=CARTESIAN_POINT('Ctrl Pts',(-41.3717545086029,37.4048782501681,38.739352647799));
#31030=CARTESIAN_POINT('Ctrl Pts',(-41.3997206011217,37.4393598755357,38.7664071998661));
#31031=CARTESIAN_POINT('Ctrl Pts',(-41.4273233951791,37.4744479465903,38.7930643608684));
#31032=CARTESIAN_POINT('Ctrl Pts',(-41.4545494627047,37.510125393861,38.8193111627622));
#31033=CARTESIAN_POINT('Ctrl Pts',(-41.4817755302303,37.5458028411317,38.8455579646562));
#31034=CARTESIAN_POINT('Ctrl Pts',(-41.5086248703647,37.5820696634925,38.8713944066132));
#31035=CARTESIAN_POINT('Ctrl Pts',(-41.5350844215741,37.6189082180394,38.8968079198494));
#31036=CARTESIAN_POINT('Ctrl Pts',(-41.5615439727835,37.6557467725863,38.9222214330856));
#31037=CARTESIAN_POINT('Ctrl Pts',(-41.5876137342328,37.6931570581567,38.9472120167988));
#31038=CARTESIAN_POINT('Ctrl Pts',(-41.6132810236338,37.7311208755803,38.9717675136936));
#31039=CARTESIAN_POINT('Ctrl Pts',(-41.6389483130347,37.7690846930039,38.9963230105884));
#31040=CARTESIAN_POINT('Ctrl Pts',(-41.6642131295771,37.8076020410825,39.02044341989));
#31041=CARTESIAN_POINT('Ctrl Pts',(-41.6890631825583,37.8466541820877,39.0441170076211));
#31042=CARTESIAN_POINT('Ctrl Pts',(-41.7139132355395,37.8857063230928,39.0677905953522));
#31043=CARTESIAN_POINT('Ctrl Pts',(-41.7383485241752,37.9252932557919,39.0910173607657));
#31044=CARTESIAN_POINT('Ctrl Pts',(-41.7623571613074,37.9653957221302,39.1137860046199));
#31045=CARTESIAN_POINT('Ctrl Pts',(-41.7863657984395,38.0054981884685,39.1365546484741));
#31046=CARTESIAN_POINT('Ctrl Pts',(-41.8099477833104,38.0461161871802,39.1588651700504));
#31047=CARTESIAN_POINT('Ctrl Pts',(-41.8330916438728,38.0872299586229,39.1807067158369));
#31048=CARTESIAN_POINT('Ctrl Pts',(-41.8562355044352,38.1283437300656,39.2025482616234));
#31049=CARTESIAN_POINT('Ctrl Pts',(-41.8789412399588,38.1699532729415,39.2239208309306));
#31050=CARTESIAN_POINT('Ctrl Pts',(-41.9011978046699,38.2120383452466,39.2448140265372));
#31051=CARTESIAN_POINT('Ctrl Pts',(-41.923454369381,38.2541234175516,39.2657072221438));
#31052=CARTESIAN_POINT('Ctrl Pts',(-41.9452617625771,38.2966840179575,39.2861210433902));
#31053=CARTESIAN_POINT('Ctrl Pts',(-41.9666093755058,38.3396994417945,39.3060455594619));
#31054=CARTESIAN_POINT('Ctrl Pts',(-41.9879569884345,38.3827148656314,39.3259700755336));
#31055=CARTESIAN_POINT('Ctrl Pts',(-42.0088448204219,38.4261851115417,39.3454052858018));
#31056=CARTESIAN_POINT('Ctrl Pts',(-42.0292627100592,38.4700890323357,39.3643417355216));
#31057=CARTESIAN_POINT('Ctrl Pts',(-42.0496805996965,38.5139929531297,39.3832781852415));
#31058=CARTESIAN_POINT('Ctrl Pts',(-42.0696285463391,38.5583305474217,39.4017158738155));
#31059=CARTESIAN_POINT('Ctrl Pts',(-42.089096845809,38.6030802460786,39.4196458317682));
#31060=CARTESIAN_POINT('Ctrl Pts',(-42.1085651452789,38.6478299447355,39.4375757897208));
#31061=CARTESIAN_POINT('Ctrl Pts',(-42.1275537969615,38.6929917463449,39.4549980164863));
#31062=CARTESIAN_POINT('Ctrl Pts',(-42.1460535633518,38.7385436808176,39.4719040365861));
#31063=CARTESIAN_POINT('Ctrl Pts',(-42.1645533297421,38.7840956152903,39.4888100566859));
#31064=CARTESIAN_POINT('Ctrl Pts',(-42.1825642102562,38.8300376811886,39.5051998695865));
#31065=CARTESIAN_POINT('Ctrl Pts',(-42.2000774430502,38.8763475288439,39.521065502053));
#31066=CARTESIAN_POINT('Ctrl Pts',(-42.2175906758442,38.9226573764992,39.5369311345194));
#31067=CARTESIAN_POINT('Ctrl Pts',(-42.2346062603653,38.9693350044501,39.5522725860509));
#31068=CARTESIAN_POINT('Ctrl Pts',(-42.2511159189565,39.0163577051954,39.5670823934142));
#31069=CARTESIAN_POINT('Ctrl Pts',(-42.2676255775476,39.0633804059407,39.5818922007775));
#31070=CARTESIAN_POINT('Ctrl Pts',(-42.2836293096875,39.1107481779964,39.5961703635052));
#31071=CARTESIAN_POINT('Ctrl Pts',(-42.2991193299602,39.1584379781235,39.6099099356275));
#31072=CARTESIAN_POINT('Ctrl Pts',(-42.3146231168746,39.2061701622101,39.6236617186936));
#31073=CARTESIAN_POINT('Ctrl Pts',(-42.3296122779107,39.2542249455147,39.6368739529574));
#31074=CARTESIAN_POINT('Ctrl Pts',(-42.3440795080264,39.302578909153,39.6495401993338));
#31075=CARTESIAN_POINT('Ctrl Pts',(-41.2672744347863,37.3041013800735,38.6761124197842));
#31076=CARTESIAN_POINT('Ctrl Pts',(-41.2965635232959,37.3380978767079,38.7046002687137));
#31077=CARTESIAN_POINT('Ctrl Pts',(-41.3254874763212,37.3727451372724,38.7326869200393));
#31078=CARTESIAN_POINT('Ctrl Pts',(-41.3540316073419,37.4080255704625,38.7603581136382));
#31079=CARTESIAN_POINT('Ctrl Pts',(-41.3825757383625,37.4433060036527,38.7880293072371));
#31080=CARTESIAN_POINT('Ctrl Pts',(-41.4107400463986,37.4792196082576,38.8152850421596));
#31081=CARTESIAN_POINT('Ctrl Pts',(-41.4385102302705,37.5157481505658,38.8421114797774));
#31082=CARTESIAN_POINT('Ctrl Pts',(-41.4662804141424,37.552276692874,38.8689379173952));
#31083=CARTESIAN_POINT('Ctrl Pts',(-41.4936564728967,37.5894201716319,38.8953350567876));
#31084=CARTESIAN_POINT('Ctrl Pts',(-41.5206245051938,37.6271597292047,38.92128949485));
#31085=CARTESIAN_POINT('Ctrl Pts',(-41.5475925374909,37.6648992867775,38.9472439329125));
#31086=CARTESIAN_POINT('Ctrl Pts',(-41.5741525424049,37.7032349218701,38.9727556687541));
#31087=CARTESIAN_POINT('Ctrl Pts',(-41.60029103253,37.7421471720403,38.9978117483818));
#31088=CARTESIAN_POINT('Ctrl Pts',(-41.6264295226551,37.7810594222105,39.0228678280095));
#31089=CARTESIAN_POINT('Ctrl Pts',(-41.6521464970939,37.820548286123,39.0474682505631));
#31090=CARTESIAN_POINT('Ctrl Pts',(-41.6774288960495,37.8605937162565,39.071600524294));
#31091=CARTESIAN_POINT('Ctrl Pts',(-41.702711295005,37.90063914639,39.0957327980249));
#31092=CARTESIAN_POINT('Ctrl Pts',(-41.7275591176092,37.9412411413704,39.1193969221046));
#31093=CARTESIAN_POINT('Ctrl Pts',(-41.7519597449155,37.9823790889186,39.1425808796936));
#31094=CARTESIAN_POINT('Ctrl Pts',(-41.7763603722218,38.0235170364667,39.1657648372826));
#31095=CARTESIAN_POINT('Ctrl Pts',(-41.8003138033923,38.0651909351709,39.1884686275849));
#31096=CARTESIAN_POINT('Ctrl Pts',(-41.8238078731261,38.1073796288875,39.210680720854));
#31097=CARTESIAN_POINT('Ctrl Pts',(-41.8473019428599,38.1495683226041,39.2328928141231));
#31098=CARTESIAN_POINT('Ctrl Pts',(-41.8703366503502,38.1922718098854,39.2546132095963));
#31099=CARTESIAN_POINT('Ctrl Pts',(-41.8929002962776,38.2354684121674,39.2758308763104));
#31100=CARTESIAN_POINT('Ctrl Pts',(-41.9154639422049,38.2786650144493,39.2970485430246));
#31101=CARTESIAN_POINT('Ctrl Pts',(-41.9375565257944,38.3223547302496,39.3177634802512));
#31102=CARTESIAN_POINT('Ctrl Pts',(-41.9591668255718,38.3665153805573,39.3379651669958));
#31103=CARTESIAN_POINT('Ctrl Pts',(-41.9807771253491,38.4106760308652,39.3581668537404));
#31104=CARTESIAN_POINT('Ctrl Pts',(-42.001905140572,38.4553076141653,39.3778552893091));
#31105=CARTESIAN_POINT('Ctrl Pts',(-42.0225401389914,38.5003874734805,39.3970204733452));
#31106=CARTESIAN_POINT('Ctrl Pts',(-42.0431751374107,38.5454673327957,39.4161856573814));
#31107=CARTESIAN_POINT('Ctrl Pts',(-42.0633171183177,38.5909954665794,39.4348275892266));
#31108=CARTESIAN_POINT('Ctrl Pts',(-42.0829558495725,38.636948762853,39.4529367993031));
#31109=CARTESIAN_POINT('Ctrl Pts',(-42.1025945808273,38.6829020591267,39.4710460093795));
#31110=CARTESIAN_POINT('Ctrl Pts',(-42.1217300617553,38.7292805163137,39.4886224970651));
#31111=CARTESIAN_POINT('Ctrl Pts',(-42.1403525707042,38.7760605908604,39.5056573331652));
#31112=CARTESIAN_POINT('Ctrl Pts',(-42.1589750796531,38.8228406654072,39.5226921692653));
#31113=CARTESIAN_POINT('Ctrl Pts',(-42.1770846159829,38.8700223557087,39.5391853531945));
#31114=CARTESIAN_POINT('Ctrl Pts',(-42.1946719783898,38.9175817104993,39.5551285051979));
#31115=CARTESIAN_POINT('Ctrl Pts',(-42.2122593407967,38.9651410652898,39.5710716572012));
#31116=CARTESIAN_POINT('Ctrl Pts',(-42.2293245286761,39.0130780829377,39.5864647767308));
#31117=CARTESIAN_POINT('Ctrl Pts',(-42.2458588704062,39.0613684287422,39.6013000419716));
#31118=CARTESIAN_POINT('Ctrl Pts',(-42.2623932121364,39.1096587745465,39.6161353072125));
#31119=CARTESIAN_POINT('Ctrl Pts',(-42.2783967071489,39.1583024468505,39.6304127176547));
#31120=CARTESIAN_POINT('Ctrl Pts',(-42.2938612223017,39.2072747521832,39.6441250173583));
#31121=CARTESIAN_POINT('Ctrl Pts',(-42.3093394814288,39.2562905812924,39.6578495037676));
#31122=CARTESIAN_POINT('Ctrl Pts',(-42.3242778017089,39.3056356261468,39.6710078740436));
#31123=CARTESIAN_POINT('Ctrl Pts',(-42.3386685764868,39.3552847927467,39.6835934276506));
#31124=CARTESIAN_POINT('Ctrl Pts',(-41.2477503364942,37.30491207051,38.695196554612));
#31125=CARTESIAN_POINT('Ctrl Pts',(-41.2776316088372,37.3396307438627,38.7243168606012));
#31126=CARTESIAN_POINT('Ctrl Pts',(-41.3071320670255,37.3750281244084,38.7530187418362));
#31127=CARTESIAN_POINT('Ctrl Pts',(-41.3362360873192,37.4110854666086,38.7812869986631));
#31128=CARTESIAN_POINT('Ctrl Pts',(-41.3653401076128,37.4471428088089,38.8095552554899));
#31129=CARTESIAN_POINT('Ctrl Pts',(-41.3940476889249,37.4838601113176,38.8373898868531));
#31130=CARTESIAN_POINT('Ctrl Pts',(-41.4223436270301,37.5212179301777,38.8647761519648));
#31131=CARTESIAN_POINT('Ctrl Pts',(-41.4506395651352,37.5585757490378,38.8921624170764));
#31132=CARTESIAN_POINT('Ctrl Pts',(-41.4785238589767,37.5965740828547,38.919100314914));
#31133=CARTESIAN_POINT('Ctrl Pts',(-41.5059817399214,37.6351928098112,38.9455755791419));
#31134=CARTESIAN_POINT('Ctrl Pts',(-41.5334396208661,37.6738115367676,38.9720508433698));
#31135=CARTESIAN_POINT('Ctrl Pts',(-41.5604710878885,37.7130506554219,38.9980634729996));
#31136=CARTESIAN_POINT('Ctrl Pts',(-41.5870618235653,37.7528893873707,39.0235996912331));
#31137=CARTESIAN_POINT('Ctrl Pts',(-41.6136525592421,37.7927281193195,39.0491359094667));
#31138=CARTESIAN_POINT('Ctrl Pts',(-41.6398025625802,37.8331664630757,39.0741957153506));
#31139=CARTESIAN_POINT('Ctrl Pts',(-41.665497982507,37.8741830056177,39.0987658361924));
#31140=CARTESIAN_POINT('Ctrl Pts',(-41.6911934024338,37.9151995481598,39.1233359570343));
#31141=CARTESIAN_POINT('Ctrl Pts',(-41.7164342379895,37.9567942879567,39.1474163919165));
#31142=CARTESIAN_POINT('Ctrl Pts',(-41.7412071191007,37.9989452000071,39.1709943862882));
#31143=CARTESIAN_POINT('Ctrl Pts',(-41.7659800002119,38.0410961120575,39.1945723806599));
#31144=CARTESIAN_POINT('Ctrl Pts',(-41.790284925953,38.083803194786,39.2176479336384));
#31145=CARTESIAN_POINT('Ctrl Pts',(-41.8141090213905,38.1270438345005,39.2402088223063));
#31146=CARTESIAN_POINT('Ctrl Pts',(-41.8379331168278,38.1702844742152,39.2627697109742));
#31147=CARTESIAN_POINT('Ctrl Pts',(-41.8612763810714,38.2140586693022,39.284815934489));
#31148=CARTESIAN_POINT('Ctrl Pts',(-41.8841264479437,38.2583432412732,39.3063358144816));
#31149=CARTESIAN_POINT('Ctrl Pts',(-41.9069765148161,38.3026278132442,39.3278556944743));
#31150=CARTESIAN_POINT('Ctrl Pts',(-41.9293333834634,38.3474227604456,39.3488492301403));
#31151=CARTESIAN_POINT('Ctrl Pts',(-41.9511852095457,38.3927043641151,39.3693053000282));
#31152=CARTESIAN_POINT('Ctrl Pts',(-41.9730370356281,38.4379859677846,39.3897613699161));
#31153=CARTESIAN_POINT('Ctrl Pts',(-41.9943838183286,38.4837542262293,39.409679973259));
#31154=CARTESIAN_POINT('Ctrl Pts',(-42.015214247673,38.5299849054721,39.4290505572722));
#31155=CARTESIAN_POINT('Ctrl Pts',(-42.0360446770173,38.5762155847148,39.4484211412853));
#31156=CARTESIAN_POINT('Ctrl Pts',(-42.0563587522268,38.6229086830301,39.4672437052448));
#31157=CARTESIAN_POINT('Ctrl Pts',(-42.0761457096572,38.6700394768505,39.4855082762004));
#31158=CARTESIAN_POINT('Ctrl Pts',(-42.0959326670877,38.7171702706709,39.503772847156));
#31159=CARTESIAN_POINT('Ctrl Pts',(-42.1151925059993,38.7647387582413,39.521479424428));
#31160=CARTESIAN_POINT('Ctrl Pts',(-42.1339150204658,38.8127197525332,39.5386186254455));
#31161=CARTESIAN_POINT('Ctrl Pts',(-42.1526375349323,38.8607007468251,39.555757826463));
#31162=CARTESIAN_POINT('Ctrl Pts',(-42.1708227242539,38.9090942460473,39.572329650585));
#31163=CARTESIAN_POINT('Ctrl Pts',(-42.1884609510199,38.9578746263604,39.5883253155651));
#31164=CARTESIAN_POINT('Ctrl Pts',(-42.2060991777859,39.0066550066736,39.6043209805452));
#31165=CARTESIAN_POINT('Ctrl Pts',(-42.2231904413368,39.0558222662528,39.6197404857819));
#31166=CARTESIAN_POINT('Ctrl Pts',(-42.2397256829768,39.1053503715122,39.6345756586278));
#31167=CARTESIAN_POINT('Ctrl Pts',(-42.2562609246168,39.1548784767715,39.6494108314737));
#31168=CARTESIAN_POINT('Ctrl Pts',(-42.2722401437274,39.2047674258621,39.6636616713738));
#31169=CARTESIAN_POINT('Ctrl Pts',(-42.2876548699138,39.254990802981,39.6773206239347));
#31170=CARTESIAN_POINT('Ctrl Pts',(-42.3030832958249,39.3052588157572,39.6909917157894));
#31171=CARTESIAN_POINT('Ctrl Pts',(-42.3179462244095,39.3558618493942,39.7040698672579));
#31172=CARTESIAN_POINT('Ctrl Pts',(-42.3322357615307,39.4067730623479,39.716548131702));
#31173=CARTESIAN_POINT('Ctrl Pts',(-41.2282110280907,37.3057050044843,38.7142657303796));
#31174=CARTESIAN_POINT('Ctrl Pts',(-41.2586695369814,37.3411274416385,38.7440022303608));
#31175=CARTESIAN_POINT('Ctrl Pts',(-41.2887314977015,37.3772566278719,38.7733030176263));
#31176=CARTESIAN_POINT('Ctrl Pts',(-41.3183803184579,37.4140726227688,38.8021519204898));
#31177=CARTESIAN_POINT('Ctrl Pts',(-41.3480291392142,37.4508886176657,38.8310008233533));
#31178=CARTESIAN_POINT('Ctrl Pts',(-41.3772648188021,37.4883914197305,38.8593978406427));
#31179=CARTESIAN_POINT('Ctrl Pts',(-41.4060712214694,37.5265603304216,38.88732729948));
#31180=CARTESIAN_POINT('Ctrl Pts',(-41.4348776241367,37.5647292411127,38.9152567583173));
#31181=CARTESIAN_POINT('Ctrl Pts',(-41.463254748713,37.6035642588794,38.9427186575678));
#31182=CARTESIAN_POINT('Ctrl Pts',(-41.4911869332995,37.6430439499042,38.9696978404639));
#31183=CARTESIAN_POINT('Ctrl Pts',(-41.519119117886,37.6825236409288,38.9966770233599));
#31184=CARTESIAN_POINT('Ctrl Pts',(-41.5466063613479,37.7226480036075,39.0231734888054));
#31185=CARTESIAN_POINT('Ctrl Pts',(-41.5736334929296,37.7633948925073,39.0491726128747));
#31186=CARTESIAN_POINT('Ctrl Pts',(-41.6006606245112,37.8041417814072,39.075171736944));
#31187=CARTESIAN_POINT('Ctrl Pts',(-41.6272276431146,37.8455111948727,39.1006735185808));
#31188=CARTESIAN_POINT('Ctrl Pts',(-41.6533198858744,37.8874803003029,39.1256638828453));
#31189=CARTESIAN_POINT('Ctrl Pts',(-41.6794121286342,37.9294494057331,39.1506542471098));
#31190=CARTESIAN_POINT('Ctrl Pts',(-41.7050295944903,37.9720182014228,39.1751331929866));
#31191=CARTESIAN_POINT('Ctrl Pts',(-41.7301581446544,38.0151631928082,39.1990872100594));
#31192=CARTESIAN_POINT('Ctrl Pts',(-41.7552866948186,38.0583081841935,39.2230412271322));
#31193=CARTESIAN_POINT('Ctrl Pts',(-41.7799263282698,38.1020293695198,39.2464703144257));
#31194=CARTESIAN_POINT('Ctrl Pts',(-41.8040634459051,38.1463026181998,39.269361540965));
#31195=CARTESIAN_POINT('Ctrl Pts',(-41.8282005635404,38.1905758668799,39.2922527675044));
#31196=CARTESIAN_POINT('Ctrl Pts',(-41.8518351643792,38.2354011771156,39.31460613236));
#31197=CARTESIAN_POINT('Ctrl Pts',(-41.8749542040155,38.2807538089233,39.3364092982614));
#31198=CARTESIAN_POINT('Ctrl Pts',(-41.8980732436519,38.326106440731,39.3582124641628));
#31199=CARTESIAN_POINT('Ctrl Pts',(-41.9206767211466,38.3719863922678,39.3794654302238));
#31200=CARTESIAN_POINT('Ctrl Pts',(-41.9427521611915,38.4183683414821,39.4001564665152));
#31201=CARTESIAN_POINT('Ctrl Pts',(-41.9648276012364,38.4647502906964,39.4208475028065));
#31202=CARTESIAN_POINT('Ctrl Pts',(-41.9863750029347,38.5116342357014,39.4409766084852));
#31203=CARTESIAN_POINT('Ctrl Pts',(-42.0073824738472,38.5589943003163,39.460532673898));
#31204=CARTESIAN_POINT('Ctrl Pts',(-42.0283899447598,38.6063543649314,39.4800887393107));
#31205=CARTESIAN_POINT('Ctrl Pts',(-42.0488574840331,38.6541905472324,39.499071763663));
#31206=CARTESIAN_POINT('Ctrl Pts',(-42.0687737952257,38.70247644548,39.5174712698466));
#31207=CARTESIAN_POINT('Ctrl Pts',(-42.0886901064184,38.7507623437277,39.5358707760302));
#31208=CARTESIAN_POINT('Ctrl Pts',(-42.108055188721,38.799497955964,39.5536867633005));
#31209=CARTESIAN_POINT('Ctrl Pts',(-42.1268583541603,38.8486563840293,39.5709093986544));
#31210=CARTESIAN_POINT('Ctrl Pts',(-42.1456615195996,38.8978148120945,39.5881320340084));
#31211=CARTESIAN_POINT('Ctrl Pts',(-42.1639027674119,38.947396053991,39.6047613167461));
#31212=CARTESIAN_POINT('Ctrl Pts',(-42.1815720298895,38.9973727448544,39.6207880688421));
#31213=CARTESIAN_POINT('Ctrl Pts',(-42.199241292367,39.0473494357178,39.6368148209381));
#31214=CARTESIAN_POINT('Ctrl Pts',(-42.2163385687924,39.0977215735138,39.6522390417384));
#31215=CARTESIAN_POINT('Ctrl Pts',(-42.232854422839,39.1484613568588,39.667052218309));
#31216=CARTESIAN_POINT('Ctrl Pts',(-42.2493702768857,39.1992011402039,39.6818653948796));
#31217=CARTESIAN_POINT('Ctrl Pts',(-42.2653047078826,39.2503085670367,39.6960675266187));
#31218=CARTESIAN_POINT('Ctrl Pts',(-42.2806489213008,39.301755430153,39.7096507750877));
#31219=CARTESIAN_POINT('Ctrl Pts',(-42.2960067717759,39.3532480162909,39.723246095569));
#31220=CARTESIAN_POINT('Ctrl Pts',(-42.3107733544778,39.4050806402349,39.7362214316859));
#31221=CARTESIAN_POINT('Ctrl Pts',(-42.3249405046544,39.4572246438149,39.7485696090469));
#31222=CARTESIAN_POINT('Ctrl Pts',(-41.2086717196872,37.3064979384586,38.7333349061473));
#31223=CARTESIAN_POINT('Ctrl Pts',(-41.2397074651256,37.3426241394144,38.7636876001203));
#31224=CARTESIAN_POINT('Ctrl Pts',(-41.2703309283775,37.3794851313355,38.7935872934165));
#31225=CARTESIAN_POINT('Ctrl Pts',(-41.3005245495965,37.417059778929,38.8230168423166));
#31226=CARTESIAN_POINT('Ctrl Pts',(-41.3307181708155,37.4546344265226,38.8524463912167));
#31227=CARTESIAN_POINT('Ctrl Pts',(-41.3604819486794,37.4929227281434,38.8814057944323));
#31228=CARTESIAN_POINT('Ctrl Pts',(-41.3897988159087,37.5319027306655,38.9098784469952));
#31229=CARTESIAN_POINT('Ctrl Pts',(-41.4191156831381,37.5708827331875,38.9383510995581));
#31230=CARTESIAN_POINT('Ctrl Pts',(-41.4479856384492,37.6105544349041,38.9663370002217));
#31231=CARTESIAN_POINT('Ctrl Pts',(-41.4763921266775,37.6508950899971,38.9938201017858));
#31232=CARTESIAN_POINT('Ctrl Pts',(-41.5047986149058,37.69123574509,39.02130320335));
#31233=CARTESIAN_POINT('Ctrl Pts',(-41.5327416348073,37.7322453517931,39.0482835046113));
#31234=CARTESIAN_POINT('Ctrl Pts',(-41.5602051622938,37.7739003976439,39.0747455345162));
#31235=CARTESIAN_POINT('Ctrl Pts',(-41.5876686897804,37.8155554434947,39.1012075644212));
#31236=CARTESIAN_POINT('Ctrl Pts',(-41.614652723649,37.8578559266697,39.127151321811));
#31237=CARTESIAN_POINT('Ctrl Pts',(-41.6411417892418,37.900777594988,39.1525619294982));
#31238=CARTESIAN_POINT('Ctrl Pts',(-41.6676308548345,37.9436992633064,39.1779725371852));
#31239=CARTESIAN_POINT('Ctrl Pts',(-41.6936249509911,37.987242114889,39.2028499940568));
#31240=CARTESIAN_POINT('Ctrl Pts',(-41.7191091702082,38.0313811856093,39.2271800338306));
#31241=CARTESIAN_POINT('Ctrl Pts',(-41.7445933894253,38.0755202563297,39.2515100736044));
#31242=CARTESIAN_POINT('Ctrl Pts',(-41.7695677305865,38.1202555442535,39.2752926952129));
#31243=CARTESIAN_POINT('Ctrl Pts',(-41.7940178704198,38.165561401899,39.2985142596238));
#31244=CARTESIAN_POINT('Ctrl Pts',(-41.818468010253,38.2108672595447,39.3217358240347));
#31245=CARTESIAN_POINT('Ctrl Pts',(-41.842393947687,38.256743684929,39.344396330231));
#31246=CARTESIAN_POINT('Ctrl Pts',(-41.8657819600873,38.3031643765735,39.3664827820411));
#31247=CARTESIAN_POINT('Ctrl Pts',(-41.8891699724877,38.349585068218,39.3885692338512));
#31248=CARTESIAN_POINT('Ctrl Pts',(-41.9120200588297,38.39655002409,39.4100816303073));
#31249=CARTESIAN_POINT('Ctrl Pts',(-41.9343191128372,38.4440323188491,39.4310076330021));
#31250=CARTESIAN_POINT('Ctrl Pts',(-41.9566181668448,38.4915146136082,39.4519336356969));
#31251=CARTESIAN_POINT('Ctrl Pts',(-41.9783661875408,38.5395142451733,39.4722732437114));
#31252=CARTESIAN_POINT('Ctrl Pts',(-41.9995507000215,38.5880036951607,39.4920147905237));
#31253=CARTESIAN_POINT('Ctrl Pts',(-42.0207352125022,38.6364931451479,39.511756337336));
#31254=CARTESIAN_POINT('Ctrl Pts',(-42.0413562158394,38.6854724114346,39.5308998220812));
#31255=CARTESIAN_POINT('Ctrl Pts',(-42.0614018807942,38.7349134141096,39.5494342634928));
#31256=CARTESIAN_POINT('Ctrl Pts',(-42.081447545749,38.7843544167844,39.5679687049045));
#31257=CARTESIAN_POINT('Ctrl Pts',(-42.1009178714426,38.8342571536868,39.585894102173));
#31258=CARTESIAN_POINT('Ctrl Pts',(-42.1198016878547,38.8845930155253,39.6032001718634));
#31259=CARTESIAN_POINT('Ctrl Pts',(-42.1386855042668,38.9349288773639,39.6205062415537));
#31260=CARTESIAN_POINT('Ctrl Pts',(-42.1569828105698,38.9856978619347,39.6371929829072));
#31261=CARTESIAN_POINT('Ctrl Pts',(-42.174683108759,39.0368708633483,39.6532508221192));
#31262=CARTESIAN_POINT('Ctrl Pts',(-42.1923834069483,39.088043864762,39.6693086613312));
#31263=CARTESIAN_POINT('Ctrl Pts',(-42.2094866962481,39.1396208807746,39.6847375976949));
#31264=CARTESIAN_POINT('Ctrl Pts',(-42.2259831627013,39.1915723422055,39.6995287779901));
#31265=CARTESIAN_POINT('Ctrl Pts',(-42.2424796291546,39.2435238036363,39.7143199582854));
#31266=CARTESIAN_POINT('Ctrl Pts',(-42.2583692720378,39.2958497082112,39.7284733818636));
#31267=CARTESIAN_POINT('Ctrl Pts',(-42.2736429726878,39.348520057325,39.7419809262407));
#31268=CARTESIAN_POINT('Ctrl Pts',(-42.2889302477269,39.4012372168246,39.7555004753485));
#31269=CARTESIAN_POINT('Ctrl Pts',(-42.3036004845462,39.4542994310756,39.768372996114));
#31270=CARTESIAN_POINT('Ctrl Pts',(-42.3176452477781,39.5076762252817,39.7805910863918));
#31271=CARTESIAN_POINT('Ctrl Pts',(-41.1891171828089,37.3072730945328,38.7523891047943));
#31272=CARTESIAN_POINT('Ctrl Pts',(-41.2207151987186,37.3440846246979,38.7833417116339));
#31273=CARTESIAN_POINT('Ctrl Pts',(-41.2518851430282,37.3816590864308,38.8138239689665));
#31274=CARTESIAN_POINT('Ctrl Pts',(-41.2826084569984,37.4199741089117,38.8438177285332));
#31275=CARTESIAN_POINT('Ctrl Pts',(-41.3133317709687,37.4582891313924,38.8738114880999));
#31276=CARTESIAN_POINT('Ctrl Pts',(-41.343608453149,37.4973447128122,38.9033167484847));
#31277=CARTESIAN_POINT('Ctrl Pts',(-41.3734204762462,37.5371176011145,38.9323159426931));
#31278=CARTESIAN_POINT('Ctrl Pts',(-41.4032324993435,37.5768904894166,38.9613151369015));
#31279=CARTESIAN_POINT('Ctrl Pts',(-41.43257986195,37.6173806827237,38.9898082635645));
#31280=CARTESIAN_POINT('Ctrl Pts',(-41.4614450896576,37.658564075392,39.0177783578423));
#31281=CARTESIAN_POINT('Ctrl Pts',(-41.4903103173653,37.6997474680603,39.0457484521201));
#31282=CARTESIAN_POINT('Ctrl Pts',(-41.5186934088111,37.7416240581456,39.0731955126921));
#31283=CARTESIAN_POINT('Ctrl Pts',(-41.5465774632538,37.7841689150809,39.1001031970481));
#31284=CARTESIAN_POINT('Ctrl Pts',(-41.5744615176964,37.8267137720161,39.1270108814041));
#31285=CARTESIAN_POINT('Ctrl Pts',(-41.6018465338191,37.869926893793,39.1533791882735));
#31286=CARTESIAN_POINT('Ctrl Pts',(-41.6287162046479,37.9137825545649,39.179192416911));
#31287=CARTESIAN_POINT('Ctrl Pts',(-41.6555858754767,37.9576382153368,39.2050056455483));
#31288=CARTESIAN_POINT('Ctrl Pts',(-41.6819401997425,38.0021364130336,39.2302637947347));
#31289=CARTESIAN_POINT('Ctrl Pts',(-41.7077634836333,38.0472506571184,39.2549518241621));
#31290=CARTESIAN_POINT('Ctrl Pts',(-41.7335867675241,38.0923649012032,39.2796398535895));
#31291=CARTESIAN_POINT('Ctrl Pts',(-41.7588790098202,38.1380951895466,39.3037577620919));
#31292=CARTESIAN_POINT('Ctrl Pts',(-41.783625148538,38.1844142984193,39.3272911876869));
#31293=CARTESIAN_POINT('Ctrl Pts',(-41.8083712872557,38.2307334072919,39.3508246132818));
#31294=CARTESIAN_POINT('Ctrl Pts',(-41.8325713212261,38.2776413345075,39.373773554858));
#31295=CARTESIAN_POINT('Ctrl Pts',(-41.8562108382094,38.325110155514,39.3961243458403));
#31296=CARTESIAN_POINT('Ctrl Pts',(-41.8798503551926,38.3725789765204,39.4184751368226));
#31297=CARTESIAN_POINT('Ctrl Pts',(-41.902929354072,38.4206086890771,39.4402277761556));
#31298=CARTESIAN_POINT('Ctrl Pts',(-41.9254340894953,38.469170701011,39.4613693089278));
#31299=CARTESIAN_POINT('Ctrl Pts',(-41.9479388249185,38.5177327129449,39.4825108417001));
#31300=CARTESIAN_POINT('Ctrl Pts',(-41.9698692958223,38.5668270219641,39.5030412669129));
#31301=CARTESIAN_POINT('Ctrl Pts',(-41.9912124400932,38.6164244022708,39.5229483567292));
#31302=CARTESIAN_POINT('Ctrl Pts',(-42.0125555843642,38.6660217825775,39.5428554465454));
#31303=CARTESIAN_POINT('Ctrl Pts',(-42.0333114009938,38.7161222318307,39.5621392000245));
#31304=CARTESIAN_POINT('Ctrl Pts',(-42.0534675266471,38.7666959253572,39.5807881309497));
#31305=CARTESIAN_POINT('Ctrl Pts',(-42.0736236523004,38.8172696188837,39.599437061875));
#31306=CARTESIAN_POINT('Ctrl Pts',(-42.0931800860248,38.8683165542964,39.6174511693651));
#31307=CARTESIAN_POINT('Ctrl Pts',(-42.1121251779732,38.9198063435073,39.6348197224895));
#31308=CARTESIAN_POINT('Ctrl Pts',(-42.1310702699216,38.9712961327183,39.6521882756139));
#31309=CARTESIAN_POINT('Ctrl Pts',(-42.1494040191985,39.0232287732974,39.6689112735516));
#31310=CARTESIAN_POINT('Ctrl Pts',(-42.1671155033061,39.0755733498729,39.6849787534261));
#31311=CARTESIAN_POINT('Ctrl Pts',(-42.1848269874139,39.1279179264482,39.7010462333006));
#31312=CARTESIAN_POINT('Ctrl Pts',(-42.201916205515,39.1806744365496,39.7164581943523));
#31313=CARTESIAN_POINT('Ctrl Pts',(-42.2183729754589,39.2338114742793,39.7312054536145));
#31314=CARTESIAN_POINT('Ctrl Pts',(-42.2348297454029,39.286948512009,39.7459527128766));
#31315=CARTESIAN_POINT('Ctrl Pts',(-42.2506540664114,39.3404660748592,39.7600352696516));
#31316=CARTESIAN_POINT('Ctrl Pts',(-42.2658365087988,39.3943323037477,39.7734447318117));
#31317=CARTESIAN_POINT('Ctrl Pts',(-42.2810324444704,39.4482464058514,39.7868661115327));
#31318=CARTESIAN_POINT('Ctrl Pts',(-42.2955853593645,39.5025097914708,39.7996131990557));
#31319=CARTESIAN_POINT('Ctrl Pts',(-42.3094865643585,39.557090100092,39.8116783828227));
#31320=CARTESIAN_POINT('Ctrl Pts',(-41.1695498758672,37.3080333426854,38.7714307441548));
#31321=CARTESIAN_POINT('Ctrl Pts',(-41.2016975079946,37.3455145501839,38.8029693924383));
#31322=CARTESIAN_POINT('Ctrl Pts',(-41.2334012260665,37.3837869243692,38.8340202841051));
#31323=CARTESIAN_POINT('Ctrl Pts',(-41.2646414427327,37.422826819611,38.8645642351373));
#31324=CARTESIAN_POINT('Ctrl Pts',(-41.2958816593989,37.4618667148527,38.8951081861696));
#31325=CARTESIAN_POINT('Ctrl Pts',(-41.3266583730689,37.5016741291636,38.9251451950123));
#31326=CARTESIAN_POINT('Ctrl Pts',(-41.3569525691191,37.542224468527,38.95465670405));
#31327=CARTESIAN_POINT('Ctrl Pts',(-41.3872467651694,37.5827748078904,38.9841682130878));
#31328=CARTESIAN_POINT('Ctrl Pts',(-41.4170584420575,37.6240680702419,39.0131542208182));
#31329=CARTESIAN_POINT('Ctrl Pts',(-41.4463691813837,37.6660787435711,39.0415968189604));
#31330=CARTESIAN_POINT('Ctrl Pts',(-41.4756799207099,37.7080894169003,39.0700394171026));
#31331=CARTESIAN_POINT('Ctrl Pts',(-41.504489720982,37.7508174990684,39.0979386042086));
#31332=CARTESIAN_POINT('Ctrl Pts',(-41.5327807827847,37.7942365915972,39.1252771434628));
#31333=CARTESIAN_POINT('Ctrl Pts',(-41.5610718445874,37.837655684126,39.1526156827169));
#31334=CARTESIAN_POINT('Ctrl Pts',(-41.5888441664803,37.8817657848052,39.1793935727274));
#31335=CARTESIAN_POINT('Ctrl Pts',(-41.6160805900283,37.9265396413109,39.2055942694438));
#31336=CARTESIAN_POINT('Ctrl Pts',(-41.6433170135763,37.9713134978166,39.2317949661601));
#31337=CARTESIAN_POINT('Ctrl Pts',(-41.6700175373926,38.0167511078695,39.2574184682485));
#31338=CARTESIAN_POINT('Ctrl Pts',(-41.6961656652258,38.0628243989772,39.2824489448684));
#31339=CARTESIAN_POINT('Ctrl Pts',(-41.7223137930589,38.1088976900851,39.3074794214883));
#31340=CARTESIAN_POINT('Ctrl Pts',(-41.7479095235777,38.1556066599023,39.3319168713652));
#31341=CARTESIAN_POINT('Ctrl Pts',(-41.7729370430994,38.2029224504587,39.3557461964314));
#31342=CARTESIAN_POINT('Ctrl Pts',(-41.7979645626212,38.2502382410151,39.3795755214976));
#31343=CARTESIAN_POINT('Ctrl Pts',(-41.8224238698717,38.2981608499019,39.40279672054));
#31344=CARTESIAN_POINT('Ctrl Pts',(-41.8462998532791,38.3466606693325,39.4253954469206));
#31345=CARTESIAN_POINT('Ctrl Pts',(-41.8701758366865,38.3951604887631,39.4479941733013));
#31346=CARTESIAN_POINT('Ctrl Pts',(-41.8934684950353,38.4442375162683,39.4699704258699));
#31347=CARTESIAN_POINT('Ctrl Pts',(-41.9161634375384,38.4938614308328,39.4913106271477));
#31348=CARTESIAN_POINT('Ctrl Pts',(-41.9388583800415,38.5434853453973,39.5126508284255));
#31349=CARTESIAN_POINT('Ctrl Pts',(-41.9609556055435,38.5936561444947,39.5333549773262));
#31350=CARTESIAN_POINT('Ctrl Pts',(-41.9824414618257,38.6443428313502,39.5534102823086));
#31351=CARTESIAN_POINT('Ctrl Pts',(-42.003927318108,38.6950295182057,39.5734655872909));
#31352=CARTESIAN_POINT('Ctrl Pts',(-42.0248018040765,38.7462320902388,39.592872047334));
#31353=CARTESIAN_POINT('Ctrl Pts',(-42.0450520229517,38.7979189132196,39.6116176726411));
#31354=CARTESIAN_POINT('Ctrl Pts',(-42.065302241827,38.8496057362004,39.6303632979483));
#31355=CARTESIAN_POINT('Ctrl Pts',(-42.0849281925779,38.9017768074975,39.6484480875653));
#31356=CARTESIAN_POINT('Ctrl Pts',(-42.1039177498013,38.9543998945179,39.6658608682567));
#31357=CARTESIAN_POINT('Ctrl Pts',(-42.1229073070247,39.0070229815383,39.683273648948));
#31358=CARTESIAN_POINT('Ctrl Pts',(-42.1412604697537,39.0600980816029,39.7000144198273));
#31359=CARTESIAN_POINT('Ctrl Pts',(-42.1589658989453,39.1135924035872,39.7160728380273));
#31360=CARTESIAN_POINT('Ctrl Pts',(-42.1766713281368,39.1670867255715,39.7321312562274));
#31361=CARTESIAN_POINT('Ctrl Pts',(-42.1937290228895,39.2210002667519,39.7475073209307));
#31362=CARTESIAN_POINT('Ctrl Pts',(-42.2101284445329,39.2752997179941,39.7621915324199));
#31363=CARTESIAN_POINT('Ctrl Pts',(-42.2265278661762,39.3295991692364,39.776875743909));
#31364=CARTESIAN_POINT('Ctrl Pts',(-42.2422690138752,39.384284527776,39.7908681014365));
#31365=CARTESIAN_POINT('Ctrl Pts',(-42.2573421623552,39.4393220076303,39.8041599601737));
#31366=CARTESIAN_POINT('Ctrl Pts',(-42.272428706985,39.4944084016404,39.8174636319526));
#31367=CARTESIAN_POINT('Ctrl Pts',(-42.2868460637406,39.5498475403269,39.8300655585839));
#31368=CARTESIAN_POINT('Ctrl Pts',(-42.3005853090107,39.605605111288,39.8419579400509));
#31369=CARTESIAN_POINT('Ctrl Pts',(-41.1499825689254,37.308793590838,38.7904723835153));
#31370=CARTESIAN_POINT('Ctrl Pts',(-41.1826798172707,37.3469444756699,38.8225970732428));
#31371=CARTESIAN_POINT('Ctrl Pts',(-41.2149173091049,37.3859147623074,38.8542165992436));
#31372=CARTESIAN_POINT('Ctrl Pts',(-41.2466744284671,37.4256795303103,38.8853107417414));
#31373=CARTESIAN_POINT('Ctrl Pts',(-41.2784315478292,37.4654442983132,38.9164048842392));
#31374=CARTESIAN_POINT('Ctrl Pts',(-41.3097082929889,37.506003545515,38.9469736415399));
#31375=CARTESIAN_POINT('Ctrl Pts',(-41.3404846619921,37.5473313359395,38.976997465407));
#31376=CARTESIAN_POINT('Ctrl Pts',(-41.3712610309953,37.5886591263641,39.0070212892741));
#31377=CARTESIAN_POINT('Ctrl Pts',(-41.401537022165,37.6307554577601,39.0365001780718));
#31378=CARTESIAN_POINT('Ctrl Pts',(-41.4312932731097,37.6735934117502,39.0654152800785));
#31379=CARTESIAN_POINT('Ctrl Pts',(-41.4610495240545,37.7164313657403,39.0943303820851));
#31380=CARTESIAN_POINT('Ctrl Pts',(-41.490286033153,37.7600109399911,39.1226816957252));
#31381=CARTESIAN_POINT('Ctrl Pts',(-41.5189841023157,37.8043042681135,39.1504510898775));
#31382=CARTESIAN_POINT('Ctrl Pts',(-41.5476821714784,37.8485975962359,39.1782204840298));
#31383=CARTESIAN_POINT('Ctrl Pts',(-41.5758417991416,37.8936046758173,39.2054079571812));
#31384=CARTESIAN_POINT('Ctrl Pts',(-41.6034449754087,37.9392967280569,39.2319961219765));
#31385=CARTESIAN_POINT('Ctrl Pts',(-41.6310481516758,37.9849887802964,39.2585842867719));
#31386=CARTESIAN_POINT('Ctrl Pts',(-41.6580948750427,38.0313658027053,39.2845731417624));
#31387=CARTESIAN_POINT('Ctrl Pts',(-41.6845678468182,38.0783981408362,39.3099460655747));
#31388=CARTESIAN_POINT('Ctrl Pts',(-41.7110408185938,38.125430478967,39.335318989387));
#31389=CARTESIAN_POINT('Ctrl Pts',(-41.7369400373351,38.1731181302579,39.3600759806385));
#31390=CARTESIAN_POINT('Ctrl Pts',(-41.7622489376609,38.2214306024981,39.384201205176));
#31391=CARTESIAN_POINT('Ctrl Pts',(-41.7875578379866,38.2697430747382,39.4083264297134));
#31392=CARTESIAN_POINT('Ctrl Pts',(-41.8122764185173,38.3186803652963,39.4318198862219));
#31393=CARTESIAN_POINT('Ctrl Pts',(-41.8363888683489,38.368211183151,39.4546665480009));
#31394=CARTESIAN_POINT('Ctrl Pts',(-41.8605013181804,38.4177420010058,39.4775132097799));
#31395=CARTESIAN_POINT('Ctrl Pts',(-41.8840076359986,38.4678663434596,39.4997130755842));
#31396=CARTESIAN_POINT('Ctrl Pts',(-41.9068927855816,38.5185521606546,39.5212519453676));
#31397=CARTESIAN_POINT('Ctrl Pts',(-41.9297779351646,38.5692379778496,39.542790815151));
#31398=CARTESIAN_POINT('Ctrl Pts',(-41.9520419152648,38.6204852670253,39.5636686877395));
#31399=CARTESIAN_POINT('Ctrl Pts',(-41.9736704835583,38.6722612604296,39.583872207888));
#31400=CARTESIAN_POINT('Ctrl Pts',(-41.9952990518517,38.7240372538339,39.6040757280365));
#31401=CARTESIAN_POINT('Ctrl Pts',(-42.0162922071592,38.7763419486468,39.6236048946434));
#31402=CARTESIAN_POINT('Ctrl Pts',(-42.0366365192564,38.829141901082,39.6424472143325));
#31403=CARTESIAN_POINT('Ctrl Pts',(-42.0569808313535,38.8819418535171,39.6612895340217));
#31404=CARTESIAN_POINT('Ctrl Pts',(-42.0766762991311,38.9352370606986,39.6794450057655));
#31405=CARTESIAN_POINT('Ctrl Pts',(-42.0957103216294,38.9889934455284,39.6969020140239));
#31406=CARTESIAN_POINT('Ctrl Pts',(-42.1147443441278,39.0427498303582,39.7143590222822));
#31407=CARTESIAN_POINT('Ctrl Pts',(-42.1331169203089,39.0969673899085,39.7311175661029));
#31408=CARTESIAN_POINT('Ctrl Pts',(-42.1508162945843,39.1516114573015,39.7471669226285));
#31409=CARTESIAN_POINT('Ctrl Pts',(-42.1685156688598,39.2062555246946,39.7632162791541));
#31410=CARTESIAN_POINT('Ctrl Pts',(-42.185541840264,39.2613260969543,39.778556447509));
#31411=CARTESIAN_POINT('Ctrl Pts',(-42.2018839136068,39.3167879617091,39.7931776112253));
#31412=CARTESIAN_POINT('Ctrl Pts',(-42.2182259869495,39.3722498264638,39.8077987749415));
#31413=CARTESIAN_POINT('Ctrl Pts',(-42.2338839613391,39.4281029806927,39.8217009332214));
#31414=CARTESIAN_POINT('Ctrl Pts',(-42.2488478159115,39.4843117115128,39.8348751885357));
#31415=CARTESIAN_POINT('Ctrl Pts',(-42.2638249694997,39.5405703974295,39.8480611523726));
#31416=CARTESIAN_POINT('Ctrl Pts',(-42.2781067681167,39.5971852891831,39.8605179181121));
#31417=CARTESIAN_POINT('Ctrl Pts',(-42.2916840536628,39.654120122484,39.872237497279));
#31418=CARTESIAN_POINT('Ctrl Pts',(-41.1304024802123,37.3095389174009,38.8095014520746));
#31419=CARTESIAN_POINT('Ctrl Pts',(-41.1636366786685,37.3483438138742,38.8421983002006));
#31420=CARTESIAN_POINT('Ctrl Pts',(-41.1963952250877,37.3879964418396,38.8743725191787));
#31421=CARTESIAN_POINT('Ctrl Pts',(-41.2286564451757,37.4284705667593,38.9060028222506));
#31422=CARTESIAN_POINT('Ctrl Pts',(-41.2609176652637,37.4689446916788,38.9376331253226));
#31423=CARTESIAN_POINT('Ctrl Pts',(-41.292681557139,37.5102403111923,38.968719510644));
#31424=CARTESIAN_POINT('Ctrl Pts',(-41.3239271041963,37.5523301043298,38.9992414107585));
#31425=CARTESIAN_POINT('Ctrl Pts',(-41.3551726512535,37.5944198974674,39.0297633108729));
#31426=CARTESIAN_POINT('Ctrl Pts',(-41.3858998516704,37.6373038617746,39.0597207240003));
#31427=CARTESIAN_POINT('Ctrl Pts',(-41.416088374312,37.6809536259616,39.0890938291726));
#31428=CARTESIAN_POINT('Ctrl Pts',(-41.4462768969536,37.7246033901487,39.1184669343448));
#31429=CARTESIAN_POINT('Ctrl Pts',(-41.4759267400592,37.7690189516703,39.1472557298488));
#31430=CARTESIAN_POINT('Ctrl Pts',(-41.5050182848403,37.8141709264161,39.1754411674048));
#31431=CARTESIAN_POINT('Ctrl Pts',(-41.5341098296213,37.859322901162,39.2036266049609));
#31432=CARTESIAN_POINT('Ctrl Pts',(-41.5626430743809,37.9052112864981,39.2312086829236));
#31433=CARTESIAN_POINT('Ctrl Pts',(-41.5905991386123,37.9518057243334,39.2581691508848));
#31434=CARTESIAN_POINT('Ctrl Pts',(-41.6185552028437,37.9984001621687,39.285129618846));
#31435=CARTESIAN_POINT('Ctrl Pts',(-41.6459340849161,38.0457006497853,39.3114684752316));
#31436=CARTESIAN_POINT('Ctrl Pts',(-41.6727176675642,38.093675895231,39.337168291625));
#31437=CARTESIAN_POINT('Ctrl Pts',(-41.6995012502123,38.1416511406767,39.3628681080184));
#31438=CARTESIAN_POINT('Ctrl Pts',(-41.7256895318736,38.1903011411542,39.3879288829204));
#31439=CARTESIAN_POINT('Ctrl Pts',(-41.7512651824761,38.2395937122107,39.412334032949));
#31440=CARTESIAN_POINT('Ctrl Pts',(-41.7768408330786,38.2888862832671,39.4367391829776));
#31441=CARTESIAN_POINT('Ctrl Pts',(-41.8018038511301,38.3388214220307,39.460488706711));
#31442=CARTESIAN_POINT('Ctrl Pts',(-41.826137716664,38.3893660940808,39.4835668877218));
#31443=CARTESIAN_POINT('Ctrl Pts',(-41.8504715821979,38.4399107661308,39.5066450687327));
#31444=CARTESIAN_POINT('Ctrl Pts',(-41.8741762937945,38.4910649685201,39.5290519056741));
#31445=CARTESIAN_POINT('Ctrl Pts',(-41.8972361634342,38.5427948605339,39.5507725698646));
#31446=CARTESIAN_POINT('Ctrl Pts',(-41.9202960330739,38.5945247525476,39.5724932340552));
#31447=CARTESIAN_POINT('Ctrl Pts',(-41.942711059411,38.6468303311674,39.5935277242253));
#31448=CARTESIAN_POINT('Ctrl Pts',(-41.9644664071168,38.6996769940964,39.613862119033));
#31449=CARTESIAN_POINT('Ctrl Pts',(-41.9862217548225,38.7525236570254,39.6341965138405));
#31450=CARTESIAN_POINT('Ctrl Pts',(-42.0073174226271,38.8059114011827,39.653830812099));
#31451=CARTESIAN_POINT('Ctrl Pts',(-42.0277394475087,38.8598049084259,39.6727520182178));
#31452=CARTESIAN_POINT('Ctrl Pts',(-42.0481614723905,38.913698415669,39.6916732243367));
#31453=CARTESIAN_POINT('Ctrl Pts',(-42.0679098531573,38.9680976828559,39.7098813372114));
#31454=CARTESIAN_POINT('Ctrl Pts',(-42.0869715175592,39.0229667226778,39.7273643041888));
#31455=CARTESIAN_POINT('Ctrl Pts',(-42.1060331819613,39.0778357624995,39.7448472711662));
#31456=CARTESIAN_POINT('Ctrl Pts',(-42.1244081288856,39.1331745717573,39.7616050912256));
#31457=CARTESIAN_POINT('Ctrl Pts',(-42.1420841941426,39.1889465415369,39.7776266705897));
#31458=CARTESIAN_POINT('Ctrl Pts',(-42.1597602593996,39.2447185113166,39.7936482499537));
#31459=CARTESIAN_POINT('Ctrl Pts',(-42.176737441957,39.3009236383667,39.808933587687));
#31460=CARTESIAN_POINT('Ctrl Pts',(-42.1930045017737,39.3575247405534,39.8234725635622));
#31461=CARTESIAN_POINT('Ctrl Pts',(-42.2092715615904,39.4141258427401,39.8380115394373));
#31462=CARTESIAN_POINT('Ctrl Pts',(-42.2248284977163,39.4711229167633,39.851804152605));
#31463=CARTESIAN_POINT('Ctrl Pts',(-42.2396650091271,39.5284782564109,39.8648412697745));
#31464=CARTESIAN_POINT('Ctrl Pts',(-42.2545147063783,39.5858845701953,39.8778899735862));
#31465=CARTESIAN_POINT('Ctrl Pts',(-42.2686426969318,39.6436497833537,39.8901818371599));
#31466=CARTESIAN_POINT('Ctrl Pts',(-42.2820396074624,39.7017356135328,39.9017087045122));
#31467=CARTESIAN_POINT('Ctrl Pts',(-41.1108115454791,37.3102715821929,38.8285198536332));
#31468=CARTESIAN_POINT('Ctrl Pts',(-41.1445718264716,37.3497169975554,38.8617768648758));
#31469=CARTESIAN_POINT('Ctrl Pts',(-41.1778405082576,37.3900385661193,38.8944937248055));
#31470=CARTESIAN_POINT('Ctrl Pts',(-41.2105948293949,37.4312087010667,38.9266480495201));
#31471=CARTESIAN_POINT('Ctrl Pts',(-41.2433491505323,37.4723788360139,38.9588023742347));
#31472=CARTESIAN_POINT('Ctrl Pts',(-41.2755891089758,37.5143975347744,38.9903941617266));
#31473=CARTESIAN_POINT('Ctrl Pts',(-41.307292647105,37.5572360494041,39.0214017978346));
#31474=CARTESIAN_POINT('Ctrl Pts',(-41.3389961852342,37.6000745640338,39.0524094339426));
#31475=CARTESIAN_POINT('Ctrl Pts',(-41.3701633010698,37.6437328918582,39.0828329167309));
#31476=CARTESIAN_POINT('Ctrl Pts',(-41.4007726709981,37.6881811631482,39.1126514313572));
#31477=CARTESIAN_POINT('Ctrl Pts',(-41.4313820409265,37.7326294344381,39.1424699459836));
#31478=CARTESIAN_POINT('Ctrl Pts',(-41.4614336630366,37.7778676464184,39.1716834905866));
#31479=CARTESIAN_POINT('Ctrl Pts',(-41.4909069769024,37.8238648484503,39.2002720781278));
#31480=CARTESIAN_POINT('Ctrl Pts',(-41.5203802907683,37.8698620504821,39.2288606656691));
#31481=CARTESIAN_POINT('Ctrl Pts',(-41.5492752945498,37.9166182396925,39.2568242943625));
#31482=CARTESIAN_POINT('Ctrl Pts',(-41.5775722191449,37.9641014268898,39.2841438323276));
#31483=CARTESIAN_POINT('Ctrl Pts',(-41.6058691437401,38.0115846140871,39.3114633702927));
#31484=CARTESIAN_POINT('Ctrl Pts',(-41.6335679873822,38.0597947963058,39.3381388158227));
#31485=CARTESIAN_POINT('Ctrl Pts',(-41.6606497993463,38.1086989895731,39.3641519183711));
#31486=CARTESIAN_POINT('Ctrl Pts',(-41.6877316113105,38.1576031828404,39.3901650209196));
#31487=CARTESIAN_POINT('Ctrl Pts',(-41.7141963899058,38.2072013841032,39.4155157788624));
#31488=CARTESIAN_POINT('Ctrl Pts',(-41.7400260287181,38.2574596597474,39.4401868479652));
#31489=CARTESIAN_POINT('Ctrl Pts',(-41.7658556675304,38.3077179353917,39.464857917068));
#31490=CARTESIAN_POINT('Ctrl Pts',(-41.791050164947,38.3586362822818,39.4888492957924));
#31491=CARTESIAN_POINT('Ctrl Pts',(-41.8155922836422,38.4101798635953,39.5121445699468));
#31492=CARTESIAN_POINT('Ctrl Pts',(-41.8401344023374,38.4617234449088,39.5354398441012));
#31493=CARTESIAN_POINT('Ctrl Pts',(-41.8640241407791,38.5138922574272,39.558039012231));
#31494=CARTESIAN_POINT('Ctrl Pts',(-41.8872451543187,38.5666506088055,39.5799266126618));
#31495=CARTESIAN_POINT('Ctrl Pts',(-41.9104661678583,38.6194089601839,39.6018142130926));
#31496=CARTESIAN_POINT('Ctrl Pts',(-41.933018455046,38.672756847126,39.6229902444558));
#31497=CARTESIAN_POINT('Ctrl Pts',(-41.9548865862779,38.7266577705944,39.6434402187408));
#31498=CARTESIAN_POINT('Ctrl Pts',(-41.9767547175098,38.780558694063,39.6638901930257));
#31499=CARTESIAN_POINT('Ctrl Pts',(-41.9979386914205,38.8350126506927,39.6836141089556));
#31500=CARTESIAN_POINT('Ctrl Pts',(-42.0184240145653,38.8899823847063,39.7025984720138));
#31501=CARTESIAN_POINT('Ctrl Pts',(-42.03890933771,38.9449521187198,39.721582835072));
#31502=CARTESIAN_POINT('Ctrl Pts',(-42.0586960088098,39.0004376266851,39.739827644073));
#31503=CARTESIAN_POINT('Ctrl Pts',(-42.0777704904129,39.0564009470683,39.7573204164618));
#31504=CARTESIAN_POINT('Ctrl Pts',(-42.0968449720159,39.1123642674515,39.7748131888505));
#31505=CARTESIAN_POINT('Ctrl Pts',(-42.1152072629313,39.1688053967588,39.7915539235346));
#31506=CARTESIAN_POINT('Ctrl Pts',(-42.1328448002259,39.2256857196479,39.8075311670013));
#31507=CARTESIAN_POINT('Ctrl Pts',(-42.1504823375205,39.2825660425371,39.823508410468));
#31508=CARTESIAN_POINT('Ctrl Pts',(-42.167395120093,39.339885555457,39.8387221617199));
#31509=CARTESIAN_POINT('Ctrl Pts',(-42.1835715767208,39.3976050421022,39.8531620119607));
#31510=CARTESIAN_POINT('Ctrl Pts',(-42.1997480333486,39.4553245287473,39.8676018622016));
#31511=CARTESIAN_POINT('Ctrl Pts',(-42.2151881630216,39.5134439855139,39.88126781053));
#31512=CARTESIAN_POINT('Ctrl Pts',(-42.2298814020625,39.5719236487986,39.8941505071107));
#31513=CARTESIAN_POINT('Ctrl Pts',(-42.2445876996116,39.6304552854542,39.9070446530932));
#31514=CARTESIAN_POINT('Ctrl Pts',(-42.2585457774315,39.6893477655214,39.919154153688));
#31515=CARTESIAN_POINT('Ctrl Pts',(-42.2717460683851,39.7485607250761,39.9304707087187));
#31516=CARTESIAN_POINT('Ctrl Pts',(-41.0716296760129,37.3117369117769,38.8665566567506));
#31517=CARTESIAN_POINT('Ctrl Pts',(-41.1064421220777,37.352463364918,38.900933994226));
#31518=CARTESIAN_POINT('Ctrl Pts',(-41.1407310745976,37.3941228146786,38.9347361360592));
#31519=CARTESIAN_POINT('Ctrl Pts',(-41.1744715978335,37.4366849696814,38.967938504059));
#31520=CARTESIAN_POINT('Ctrl Pts',(-41.2082121210694,37.4792471246843,39.0011408720588));
#31521=CARTESIAN_POINT('Ctrl Pts',(-41.2414042126494,37.5227119819385,39.0337434638919));
#31522=CARTESIAN_POINT('Ctrl Pts',(-41.2740237329226,37.5670479395526,39.065722571987));
#31523=CARTESIAN_POINT('Ctrl Pts',(-41.3066432531957,37.6113838971666,39.0977016800822));
#31524=CARTESIAN_POINT('Ctrl Pts',(-41.3386901998686,37.6565909520255,39.1290573021918));
#31525=CARTESIAN_POINT('Ctrl Pts',(-41.3701412643704,37.7026362375212,39.1597666357266));
#31526=CARTESIAN_POINT('Ctrl Pts',(-41.4015923288721,37.748681523017,39.1904759692612));
#31527=CARTESIAN_POINT('Ctrl Pts',(-41.4324475089912,37.7955650359149,39.2205390120622));
#31528=CARTESIAN_POINT('Ctrl Pts',(-41.4626843610267,37.8432526925187,39.2499338995739));
#31529=CARTESIAN_POINT('Ctrl Pts',(-41.4929212130622,37.8909403491225,39.2793287870856));
#31530=CARTESIAN_POINT('Ctrl Pts',(-41.5225397348876,37.9394321460814,39.3080555172401));
#31531=CARTESIAN_POINT('Ctrl Pts',(-41.5515183802102,37.9886928320026,39.3360931952132));
#31532=CARTESIAN_POINT('Ctrl Pts',(-41.5804970255328,38.037953517924,39.3641308731862));
#31533=CARTESIAN_POINT('Ctrl Pts',(-41.6088357923143,38.0879830893467,39.3914794970048));
#31534=CARTESIAN_POINT('Ctrl Pts',(-41.6365140629105,38.1387451782573,39.4181191718634));
#31535=CARTESIAN_POINT('Ctrl Pts',(-41.6641923335067,38.1895072671679,39.4447588467219));
#31536=CARTESIAN_POINT('Ctrl Pts',(-41.6912101059702,38.2410018700011,39.4706895707464));
#31537=CARTESIAN_POINT('Ctrl Pts',(-41.7175477212022,38.2931915548211,39.4958924779976));
#31538=CARTESIAN_POINT('Ctrl Pts',(-41.7438853364341,38.345381239641,39.5210953852488));
#31539=CARTESIAN_POINT('Ctrl Pts',(-41.7695427925807,38.398266002784,39.5455704739551));
#31540=CARTESIAN_POINT('Ctrl Pts',(-41.7945014175986,38.4518074026242,39.5692999343967));
#31541=CARTESIAN_POINT('Ctrl Pts',(-41.8194600426163,38.5053488024645,39.5930293948383));
#31542=CARTESIAN_POINT('Ctrl Pts',(-41.8437198347484,38.5595468352414,39.6160132253448));
#31543=CARTESIAN_POINT('Ctrl Pts',(-41.8672631360878,38.6143621053489,39.6382346982561));
#31544=CARTESIAN_POINT('Ctrl Pts',(-41.8908064374271,38.6691773754566,39.6604561711674));
#31545=CARTESIAN_POINT('Ctrl Pts',(-41.913633246316,38.7246098790432,39.6819152849169));
#31546=CARTESIAN_POINT('Ctrl Pts',(-41.9357269446002,38.7806193235906,39.7025964181565));
#31547=CARTESIAN_POINT('Ctrl Pts',(-41.9578206428844,38.8366287681381,39.7232775513959));
#31548=CARTESIAN_POINT('Ctrl Pts',(-41.9791812290074,38.8932151497128,39.7431807026688));
#31549=CARTESIAN_POINT('Ctrl Pts',(-41.9997931486782,38.9503373372671,39.7622913796056));
#31550=CARTESIAN_POINT('Ctrl Pts',(-42.020405068349,39.0074595248213,39.7814020565424));
#31551=CARTESIAN_POINT('Ctrl Pts',(-42.0402683201149,39.0651175143432,39.7997202577963));
#31552=CARTESIAN_POINT('Ctrl Pts',(-42.0593684361201,39.1232693958493,39.8172326410076));
#31553=CARTESIAN_POINT('Ctrl Pts',(-42.0784685521253,39.1814212773554,39.834745024219));
#31554=CARTESIAN_POINT('Ctrl Pts',(-42.0968055310227,39.2400670467618,39.8514515881527));
#31555=CARTESIAN_POINT('Ctrl Pts',(-42.1143660123925,39.2991640758699,39.8673401598247));
#31556=CARTESIAN_POINT('Ctrl Pts',(-42.1319264937623,39.358261104978,39.8832287314966));
#31557=CARTESIAN_POINT('Ctrl Pts',(-42.1487104763651,39.4178093896378,39.8982993097854));
#31558=CARTESIAN_POINT('Ctrl Pts',(-42.164705726615,39.4777656451997,39.9125409087579));
#31559=CARTESIAN_POINT('Ctrl Pts',(-42.1807009768649,39.5377219007617,39.9267825077303));
#31560=CARTESIAN_POINT('Ctrl Pts',(-42.1959074936322,39.5980861230151,39.9401951263803));
#31561=CARTESIAN_POINT('Ctrl Pts',(-42.2103141879332,39.6588144335738,39.952768981783));
#31562=CARTESIAN_POINT('Ctrl Pts',(-42.224733686078,39.7195967159722,39.9653540121073));
#31563=CARTESIAN_POINT('Ctrl Pts',(-42.2383519384309,39.7807437298567,39.9770987867444));
#31564=CARTESIAN_POINT('Ctrl Pts',(-42.2511589902305,39.8422109481628,39.9879947171316));
#31565=CARTESIAN_POINT('Ctrl Pts',(-41.032404678088,37.313151892693,38.9045510432682));
#31566=CARTESIAN_POINT('Ctrl Pts',(-41.0682260642792,37.3551057079579,38.9400009816298));
#31567=CARTESIAN_POINT('Ctrl Pts',(-41.1034918563529,37.3980497307461,38.9748404534198));
#31568=CARTESIAN_POINT('Ctrl Pts',(-41.138174829136,37.4419508125435,39.0090425656379));
#31569=CARTESIAN_POINT('Ctrl Pts',(-41.1728578019191,37.4858518943408,39.0432446778559));
#31570=CARTESIAN_POINT('Ctrl Pts',(-41.206957952664,37.5307100316709,39.0768094277934));
#31571=CARTESIAN_POINT('Ctrl Pts',(-41.240448954355,37.5764906009263,39.1097109046596));
#31572=CARTESIAN_POINT('Ctrl Pts',(-41.2739399560461,37.6222711701815,39.1426123815259));
#31573=CARTESIAN_POINT('Ctrl Pts',(-41.3068218060297,37.6689741677376,39.1748505827146));
#31574=CARTESIAN_POINT('Ctrl Pts',(-41.3390691159587,37.7165635481547,39.2064006195102));
#31575=CARTESIAN_POINT('Ctrl Pts',(-41.3713164258876,37.7641529285719,39.2379506563058));
#31576=CARTESIAN_POINT('Ctrl Pts',(-41.4029291932065,37.8126286880828,39.2688125262086));
#31577=CARTESIAN_POINT('Ctrl Pts',(-41.4338830073062,37.8619534148612,39.2989624008741));
#31578=CARTESIAN_POINT('Ctrl Pts',(-41.4648368214059,37.9112781416396,39.3291122755395));
#31579=CARTESIAN_POINT('Ctrl Pts',(-41.495131679833,37.9614518317811,39.3585501525783));
#31580=CARTESIAN_POINT('Ctrl Pts',(-41.5247441872853,38.0124357646158,39.3872533006856));
#31581=CARTESIAN_POINT('Ctrl Pts',(-41.5543566947377,38.0634196974505,39.4159564487929));
#31582=CARTESIAN_POINT('Ctrl Pts',(-41.5832868488677,38.1152138689433,39.4439248656935));
#31583=CARTESIAN_POINT('Ctrl Pts',(-41.6115123056906,38.1677783091347,39.4711369521065));
#31584=CARTESIAN_POINT('Ctrl Pts',(-41.6397377625135,38.2203427493262,39.4983490385196));
#31585=CARTESIAN_POINT('Ctrl Pts',(-41.667258519791,38.2736774540562,39.5248047922876));
#31586=CARTESIAN_POINT('Ctrl Pts',(-41.6940533192522,38.3277412655495,39.5504837794006));
#31587=CARTESIAN_POINT('Ctrl Pts',(-41.7208481187134,38.3818050770429,39.5761627665136));
#31588=CARTESIAN_POINT('Ctrl Pts',(-41.746916958233,38.4365979910208,39.601064984935));
#31589=CARTESIAN_POINT('Ctrl Pts',(-41.7722396979839,38.4920777251902,39.625171197384));
#31590=CARTESIAN_POINT('Ctrl Pts',(-41.7975624377349,38.5475574593596,39.649277409833));
#31591=CARTESIAN_POINT('Ctrl Pts',(-41.8221390757079,38.6037240093296,39.672587614397));
#31592=CARTESIAN_POINT('Ctrl Pts',(-41.8459506215336,38.6605340333161,39.6950838001461));
#31593=CARTESIAN_POINT('Ctrl Pts',(-41.8697621673592,38.7173440573026,39.7175799858952));
#31594=CARTESIAN_POINT('Ctrl Pts',(-41.8928086191474,38.7747975508094,39.7392621510436));
#31595=CARTESIAN_POINT('Ctrl Pts',(-41.9150721652353,38.8328501792156,39.7601135387513));
#31596=CARTESIAN_POINT('Ctrl Pts',(-41.9373357113232,38.8909028076218,39.7809649264589));
#31597=CARTESIAN_POINT('Ctrl Pts',(-41.9588163499428,38.9495545663332,39.8009855350698));
#31598=CARTESIAN_POINT('Ctrl Pts',(-41.9794974755781,39.0087601960735,39.8201598876478));
#31599=CARTESIAN_POINT('Ctrl Pts',(-42.0001786012135,39.0679658258137,39.8393342402259));
#31600=CARTESIAN_POINT('Ctrl Pts',(-42.0200602122213,39.1277253218975,39.8576623352476));
#31601=CARTESIAN_POINT('Ctrl Pts',(-42.0391269348214,39.1879925699966,39.8751299995309));
#31602=CARTESIAN_POINT('Ctrl Pts',(-42.0581936574215,39.2482598180956,39.8925976638143));
#31603=CARTESIAN_POINT('Ctrl Pts',(-42.076445490098,39.3090348134404,39.9092048959701));
#31604=CARTESIAN_POINT('Ctrl Pts',(-42.0938683145047,39.37027065757,39.9249388484198));
#31605=CARTESIAN_POINT('Ctrl Pts',(-42.1112911389115,39.4315065016996,39.9406728008696));
#31606=CARTESIAN_POINT('Ctrl Pts',(-42.1278849536622,39.4932031897676,39.9555334723607));
#31607=CARTESIAN_POINT('Ctrl Pts',(-42.1436369176166,39.5553131113054,39.9695093607319));
#31608=CARTESIAN_POINT('Ctrl Pts',(-42.159388881571,39.6174230328432,39.9834852491031));
#31609=CARTESIAN_POINT('Ctrl Pts',(-42.1742989934744,39.6799461829352,39.9965763532405));
#31610=CARTESIAN_POINT('Ctrl Pts',(-42.1883557092036,39.742834312327,40.0087725341494));
#31611=CARTESIAN_POINT('Ctrl Pts',(-42.2024249177355,39.8057783330818,40.0209795543245));
#31612=CARTESIAN_POINT('Ctrl Pts',(-42.2156392113969,39.8690879771839,40.0322900588763));
#31613=CARTESIAN_POINT('Ctrl Pts',(-42.2279883336041,39.9327143005348,40.042695264256));
#31614=CARTESIAN_POINT('Ctrl Pts',(-40.9931478523898,37.3145297174934,38.942514127347));
#31615=CARTESIAN_POINT('Ctrl Pts',(-41.0299452813326,37.3576697439994,38.9789998578758));
#31616=CARTESIAN_POINT('Ctrl Pts',(-41.0661548143688,37.4018575474671,39.0148396298158));
#31617=CARTESIAN_POINT('Ctrl Pts',(-41.101746827141,37.447056976221,39.0500041213249));
#31618=CARTESIAN_POINT('Ctrl Pts',(-41.1373388399133,37.492256404975,39.085168612834));
#31619=CARTESIAN_POINT('Ctrl Pts',(-41.1723133292438,37.5384674549797,39.1196578207726));
#31620=CARTESIAN_POINT('Ctrl Pts',(-41.2066416812102,37.5856523192672,39.1534435282449));
#31621=CARTESIAN_POINT('Ctrl Pts',(-41.2409700331766,37.6328371835547,39.1872292357172));
#31622=CARTESIAN_POINT('Ctrl Pts',(-41.2746522447139,37.6809958579121,39.2203114397068));
#31623=CARTESIAN_POINT('Ctrl Pts',(-41.3076607591598,37.7300889419479,39.2526630744396));
#31624=CARTESIAN_POINT('Ctrl Pts',(-41.3406692736057,37.7791820259837,39.2850147091724));
#31625=CARTESIAN_POINT('Ctrl Pts',(-41.3730040880132,37.8292095153147,39.3166357717601));
#31626=CARTESIAN_POINT('Ctrl Pts',(-41.4046387480755,37.8801304806027,39.3475003918427));
#31627=CARTESIAN_POINT('Ctrl Pts',(-41.4362734081378,37.9310514458908,39.3783650119252));
#31628=CARTESIAN_POINT('Ctrl Pts',(-41.4672079110304,37.9828658825895,39.4084731867469));
#31629=CARTESIAN_POINT('Ctrl Pts',(-41.497416948093,38.035531399393,39.4378002836969));
#31630=CARTESIAN_POINT('Ctrl Pts',(-41.5276259851557,38.0881969161966,39.467127380647));
#31631=CARTESIAN_POINT('Ctrl Pts',(-41.5571095536913,38.1417135084029,39.4956733971071));
#31632=CARTESIAN_POINT('Ctrl Pts',(-41.5858435321026,38.1960373921097,39.523414978526));
#31633=CARTESIAN_POINT('Ctrl Pts',(-41.6145775105139,38.2503612758166,39.5511565599449));
#31634=CARTESIAN_POINT('Ctrl Pts',(-41.6425618962356,38.3054924461737,39.5780937038458));
#31635=CARTESIAN_POINT('Ctrl Pts',(-41.6697737942072,38.3613857983331,39.6042043719556));
#31636=CARTESIAN_POINT('Ctrl Pts',(-41.6969856921787,38.4172791504924,39.6303150400654));
#31637=CARTESIAN_POINT('Ctrl Pts',(-41.7234250999708,38.4739346794634,39.6555992300529));
#31638=CARTESIAN_POINT('Ctrl Pts',(-41.7490703865264,38.5313060332639,39.6800362559877));
#31639=CARTESIAN_POINT('Ctrl Pts',(-41.774715673082,38.5886773870644,39.7044732819225));
#31640=CARTESIAN_POINT('Ctrl Pts',(-41.7995668361116,38.646764560572,39.7280631416226));
#31641=CARTESIAN_POINT('Ctrl Pts',(-41.8236035439601,38.7055200305232,39.7507865353521));
#31642=CARTESIAN_POINT('Ctrl Pts',(-41.8476402518086,38.7642755004743,39.7735099290817));
#31643=CARTESIAN_POINT('Ctrl Pts',(-41.8708625023299,38.823699261623,39.7953668548117));
#31644=CARTESIAN_POINT('Ctrl Pts',(-41.8932512965426,38.8837426971939,39.8163394305834));
#31645=CARTESIAN_POINT('Ctrl Pts',(-41.9156400907553,38.9437861327649,39.8373120063552));
#31646=CARTESIAN_POINT('Ctrl Pts',(-41.9371954266605,39.0044492373971,39.8574002302962));
#31647=CARTESIAN_POINT('Ctrl Pts',(-41.957899669041,39.0656823803626,39.8765876674877));
#31648=CARTESIAN_POINT('Ctrl Pts',(-41.9786039114215,39.126915523328,39.8957751046793));
#31649=CARTESIAN_POINT('Ctrl Pts',(-41.9984570584289,39.1887186991596,39.9140617534086));
#31650=CARTESIAN_POINT('Ctrl Pts',(-42.0174428674697,39.2510413443948,39.9314326526921));
#31651=CARTESIAN_POINT('Ctrl Pts',(-42.0364286765105,39.3133639896299,39.9488035519757));
#31652=CARTESIAN_POINT('Ctrl Pts',(-42.0545471458897,39.3762060987042,39.9652587002625));
#31653=CARTESIAN_POINT('Ctrl Pts',(-42.0717834522178,39.4395162581656,39.9807846349878));
#31654=CARTESIAN_POINT('Ctrl Pts',(-42.0890197585458,39.5028264176271,39.9963105697131));
#31655=CARTESIAN_POINT('Ctrl Pts',(-42.1053739002838,39.566604621823,40.0109072894906));
#31656=CARTESIAN_POINT('Ctrl Pts',(-42.1208324975039,39.6307986914473,40.0245628522043));
#31657=CARTESIAN_POINT('Ctrl Pts',(-42.136291094724,39.6949927610715,40.038218414918));
#31658=CARTESIAN_POINT('Ctrl Pts',(-42.1508541460461,39.7596026903925,40.0509328193486));
#31659=CARTESIAN_POINT('Ctrl Pts',(-42.1645097368995,39.8245756196391,40.0626956633721));
#31660=CARTESIAN_POINT('Ctrl Pts',(-42.1781774640589,39.8896062930991,40.0744689615368));
#31661=CARTESIAN_POINT('Ctrl Pts',(-42.1909361158139,39.9550006061874,40.0852890061059));
#31662=CARTESIAN_POINT('Ctrl Pts',(-42.202775234616,40.0207049625231,40.0951469283655));
#31663=CARTESIAN_POINT('Ctrl Pts',(-40.9538910266915,37.3159075422938,38.9804772114259));
#31664=CARTESIAN_POINT('Ctrl Pts',(-40.991664498386,37.3602337800409,39.0179987341218));
#31665=CARTESIAN_POINT('Ctrl Pts',(-41.0288177723846,37.405665364188,39.0548388062119));
#31666=CARTESIAN_POINT('Ctrl Pts',(-41.0653188251461,37.4521631398986,39.090965677012));
#31667=CARTESIAN_POINT('Ctrl Pts',(-41.1018198779075,37.4986609156093,39.1270925478121));
#31668=CARTESIAN_POINT('Ctrl Pts',(-41.1376687058236,37.5462248782887,39.1625062137518));
#31669=CARTESIAN_POINT('Ctrl Pts',(-41.1728344080653,37.5948140376083,39.1971761518302));
#31670=CARTESIAN_POINT('Ctrl Pts',(-41.2080001103071,37.6434031969279,39.2318460899087));
#31671=CARTESIAN_POINT('Ctrl Pts',(-41.242482683398,37.6930175480867,39.2657722966988));
#31672=CARTESIAN_POINT('Ctrl Pts',(-41.2762524023609,37.7436143357411,39.2989255293689));
#31673=CARTESIAN_POINT('Ctrl Pts',(-41.3100221213238,37.7942111233955,39.332078762039));
#31674=CARTESIAN_POINT('Ctrl Pts',(-41.3430789828199,37.8457903425465,39.3644590173116));
#31675=CARTESIAN_POINT('Ctrl Pts',(-41.3753944888448,37.8983075463442,39.3960383828113));
#31676=CARTESIAN_POINT('Ctrl Pts',(-41.4077099948697,37.9508247501419,39.427617748311));
#31677=CARTESIAN_POINT('Ctrl Pts',(-41.4392841422278,38.0042799333979,39.4583962209154));
#31678=CARTESIAN_POINT('Ctrl Pts',(-41.4700897089007,38.0586270341703,39.4883472667082));
#31679=CARTESIAN_POINT('Ctrl Pts',(-41.5008952755737,38.1129741349427,39.5182983125011));
#31680=CARTESIAN_POINT('Ctrl Pts',(-41.5309322585149,38.1682131478626,39.5474219285207));
#31681=CARTESIAN_POINT('Ctrl Pts',(-41.5601747585147,38.2242964750848,39.5756930049455));
#31682=CARTESIAN_POINT('Ctrl Pts',(-41.5894172585144,38.280379802307,39.6039640813703));
#31683=CARTESIAN_POINT('Ctrl Pts',(-41.6178652726802,38.3373074382913,39.6313826154041));
#31684=CARTESIAN_POINT('Ctrl Pts',(-41.6454942691621,38.3950303311166,39.6579249645107));
#31685=CARTESIAN_POINT('Ctrl Pts',(-41.6731232656441,38.4527532239419,39.6844673136173));
#31686=CARTESIAN_POINT('Ctrl Pts',(-41.6999332417085,38.5112713679061,39.7101334751709));
#31687=CARTESIAN_POINT('Ctrl Pts',(-41.7259010750688,38.5705343413378,39.7349013145914));
#31688=CARTESIAN_POINT('Ctrl Pts',(-41.7518689084292,38.6297973147694,39.7596691540119));
#31689=CARTESIAN_POINT('Ctrl Pts',(-41.7769945965153,38.6898051118144,39.7835386688482));
#31690=CARTESIAN_POINT('Ctrl Pts',(-41.8012564663866,38.7505060277302,39.8064892705582));
#31691=CARTESIAN_POINT('Ctrl Pts',(-41.825518336258,38.811206943646,39.8294398722682));
#31692=CARTESIAN_POINT('Ctrl Pts',(-41.8489163855125,38.8726009724366,39.8514715585798));
#31693=CARTESIAN_POINT('Ctrl Pts',(-41.87143042785,38.9346352151722,39.8725653224156));
#31694=CARTESIAN_POINT('Ctrl Pts',(-41.8939444701875,38.9966694579078,39.8936590862515));
#31695=CARTESIAN_POINT('Ctrl Pts',(-41.9155745033782,39.059343908461,39.9138149255225));
#31696=CARTESIAN_POINT('Ctrl Pts',(-41.9363018625039,39.1226045646516,39.9330154473277));
#31697=CARTESIAN_POINT('Ctrl Pts',(-41.9570292216295,39.1858652208423,39.9522159691328));
#31698=CARTESIAN_POINT('Ctrl Pts',(-41.9768539046365,39.2497120764218,39.9704611715696));
#31699=CARTESIAN_POINT('Ctrl Pts',(-41.995758800118,39.3140901187931,39.9877353058533));
#31700=CARTESIAN_POINT('Ctrl Pts',(-42.0146636955995,39.3784681611643,40.005009440137));
#31701=CARTESIAN_POINT('Ctrl Pts',(-42.0326488016815,39.4433773839681,40.0213125045549));
#31702=CARTESIAN_POINT('Ctrl Pts',(-42.0496985899308,39.5087618587613,40.0366304215558));
#31703=CARTESIAN_POINT('Ctrl Pts',(-42.0667483781801,39.5741463335546,40.0519483385566));
#31704=CARTESIAN_POINT('Ctrl Pts',(-42.0828628469054,39.6400060538784,40.0662811066205));
#31705=CARTESIAN_POINT('Ctrl Pts',(-42.0980280773912,39.7062842715891,40.0796163436766));
#31706=CARTESIAN_POINT('Ctrl Pts',(-42.1131933078771,39.7725624892997,40.0929515807328));
#31707=CARTESIAN_POINT('Ctrl Pts',(-42.1274092986177,39.8392591978499,40.1052892854568));
#31708=CARTESIAN_POINT('Ctrl Pts',(-42.1406637645954,39.9063169269512,40.1166187925947));
#31709=CARTESIAN_POINT('Ctrl Pts',(-42.1539300103823,39.9734342531166,40.1279583687489));
#31710=CARTESIAN_POINT('Ctrl Pts',(-42.1662330202308,40.0409132351909,40.1382879533356));
#31711=CARTESIAN_POINT('Ctrl Pts',(-42.1775621356279,40.1086956245114,40.1475985924751));
#31712=CARTESIAN_POINT('Ctrl Pts',(-40.914602250515,37.3172480677314,39.0184088723865));
#31713=CARTESIAN_POINT('Ctrl Pts',(-40.9533187469713,37.3627192224956,39.0569292557962));
#31714=CARTESIAN_POINT('Ctrl Pts',(-40.9913825425138,37.4093536520098,39.0947324752628));
#31715=CARTESIAN_POINT('Ctrl Pts',(-41.0287591046217,37.4571090521964,39.1317842371774));
#31716=CARTESIAN_POINT('Ctrl Pts',(-41.0661356667296,37.5048644523831,39.168835999092));
#31717=CARTESIAN_POINT('Ctrl Pts',(-41.1028249913097,37.5537408180141,39.2051362993978));
#31718=CARTESIAN_POINT('Ctrl Pts',(-41.1387937910383,37.6036938137,39.2406522060533));
#31719=CARTESIAN_POINT('Ctrl Pts',(-41.1747625907669,37.6536468093859,39.2761681127087));
#31720=CARTESIAN_POINT('Ctrl Pts',(-41.2100108617045,37.7046764296586,39.3108996218247));
#31721=CARTESIAN_POINT('Ctrl Pts',(-41.2445066219746,37.7567363880459,39.3448152225293));
#31722=CARTESIAN_POINT('Ctrl Pts',(-41.2790023822446,37.8087963464333,39.378730823234));
#31723=CARTESIAN_POINT('Ctrl Pts',(-41.3127456280685,37.861886637237,39.4118305118128));
#31724=CARTESIAN_POINT('Ctrl Pts',(-41.3457057409081,37.9159591066578,39.4440842555981));
#31725=CARTESIAN_POINT('Ctrl Pts',(-41.3786658537476,37.9700315760786,39.4763379993834));
#31726=CARTESIAN_POINT('Ctrl Pts',(-41.4108428299918,38.0250862181985,39.5077457948421));
#31727=CARTESIAN_POINT('Ctrl Pts',(-41.4422074698689,38.0810730990221,39.5382791418741));
#31728=CARTESIAN_POINT('Ctrl Pts',(-41.473572109746,38.1370599798457,39.5688124889061));
#31729=CARTESIAN_POINT('Ctrl Pts',(-41.5041244098191,38.1939790932459,39.5984713841659));
#31730=CARTESIAN_POINT('Ctrl Pts',(-41.5338366419473,38.2517788153802,39.6272289117157));
#31731=CARTESIAN_POINT('Ctrl Pts',(-41.5635488740755,38.3095785375145,39.6559864392654));
#31732=CARTESIAN_POINT('Ctrl Pts',(-41.5924210350022,38.3682588620578,39.6838425959535));
#31733=CARTESIAN_POINT('Ctrl Pts',(-41.620426918423,38.4277665687249,39.7107720987361));
#31734=CARTESIAN_POINT('Ctrl Pts',(-41.6484328018438,38.4872742753919,39.7377016015187));
#31735=CARTESIAN_POINT('Ctrl Pts',(-41.6755724046885,38.5476093576708,39.7637044474438));
#31736=CARTESIAN_POINT('Ctrl Pts',(-41.7018210899449,38.6087170951247,39.7887570321441));
#31737=CARTESIAN_POINT('Ctrl Pts',(-41.7280697752014,38.6698248325786,39.8138096168443));
#31738=CARTESIAN_POINT('Ctrl Pts',(-41.7534275399913,38.7317052185206,39.8379119375725));
#31739=CARTESIAN_POINT('Ctrl Pts',(-41.7778713612163,38.7943021313656,39.8610421113869));
#31740=CARTESIAN_POINT('Ctrl Pts',(-41.8023151824413,38.8568990442106,39.8841722852013));
#31741=CARTESIAN_POINT('Ctrl Pts',(-41.8258450574193,38.9202124771122,39.9063303095674));
#31742=CARTESIAN_POINT('Ctrl Pts',(-41.8484396186719,38.9841850088691,39.9274960626028));
#31743=CARTESIAN_POINT('Ctrl Pts',(-41.8710341799246,39.048157540626,39.9486618156382));
#31744=CARTESIAN_POINT('Ctrl Pts',(-41.8926934249723,39.1127891642374,39.9688352950196));
#31745=CARTESIAN_POINT('Ctrl Pts',(-41.9133976806671,39.1780212627951,39.9879981763989));
#31746=CARTESIAN_POINT('Ctrl Pts',(-41.934101936362,39.2432533613527,40.0071610577782));
#31747=CARTESIAN_POINT('Ctrl Pts',(-41.9538512004312,39.3090859277148,40.0253133390478));
#31748=CARTESIAN_POINT('Ctrl Pts',(-41.9726275297141,39.3754592552988,40.0424385265866));
#31749=CARTESIAN_POINT('Ctrl Pts',(-41.9914038589971,39.4418325828827,40.0595637141254));
#31750=CARTESIAN_POINT('Ctrl Pts',(-42.0092072514307,39.5087466644251,40.0756618060513));
#31751=CARTESIAN_POINT('Ctrl Pts',(-42.0260215263681,39.5761408117013,40.0907181693781));
#31752=CARTESIAN_POINT('Ctrl Pts',(-42.0428358013054,39.6435349589775,40.1057745327049));
#31753=CARTESIAN_POINT('Ctrl Pts',(-42.0586609568976,39.7114091646121,40.1197891657764));
#31754=CARTESIAN_POINT('Ctrl Pts',(-42.0734826043543,39.7797018685422,40.1327493227831));
#31755=CARTESIAN_POINT('Ctrl Pts',(-42.0883042518111,39.8479945724722,40.1457094797898));
#31756=CARTESIAN_POINT('Ctrl Pts',(-42.102122389501,39.9167057672238,40.1576151593043));
#31757=CARTESIAN_POINT('Ctrl Pts',(-42.1149244465968,39.9857731322772,40.1684555258249));
#31758=CARTESIAN_POINT('Ctrl Pts',(-42.1277378814269,40.0549018804439,40.1793055266415));
#31759=CARTESIAN_POINT('Ctrl Pts',(-42.1395334273784,40.1243874247088,40.1890883188462));
#31760=CARTESIAN_POINT('Ctrl Pts',(-42.1503003257741,40.1941666288214,40.1977949731605));
#31761=CARTESIAN_POINT('Ctrl Pts',(-40.8752893413701,37.3185604200591,39.0563167987067));
#31762=CARTESIAN_POINT('Ctrl Pts',(-40.9149228371848,37.3651437030407,39.0958065436101));
#31763=CARTESIAN_POINT('Ctrl Pts',(-40.9538709279309,37.4129485471481,39.1345431904534));
#31764=CARTESIAN_POINT('Ctrl Pts',(-40.992096465966,37.4619293574053,39.1724897932637));
#31765=CARTESIAN_POINT('Ctrl Pts',(-41.030322004001,37.5109101676627,39.2104363960739));
#31766=CARTESIAN_POINT('Ctrl Pts',(-41.0678249846864,37.5610669381261,39.2475929502463));
#31767=CARTESIAN_POINT('Ctrl Pts',(-41.1045696386867,37.6123518306155,39.2839240168577));
#31768=CARTESIAN_POINT('Ctrl Pts',(-41.1413142926869,37.6636367231049,39.3202550834691));
#31769=CARTESIAN_POINT('Ctrl Pts',(-41.1773006155432,37.7160497313968,39.3557606581107));
#31770=CARTESIAN_POINT('Ctrl Pts',(-41.2124942844676,37.7695408653723,39.3904068765195));
#31771=CARTESIAN_POINT('Ctrl Pts',(-41.2476879533919,37.8230319993478,39.4250530949283));
#31772=CARTESIAN_POINT('Ctrl Pts',(-41.2820889641137,37.8776012525156,39.4588399529));
#31773=CARTESIAN_POINT('Ctrl Pts',(-41.315664505873,37.9331965781883,39.491735225437));
#31774=CARTESIAN_POINT('Ctrl Pts',(-41.3492400476323,37.988791903861,39.5246304979741));
#31775=CARTESIAN_POINT('Ctrl Pts',(-41.3819901163548,38.045413295292,39.5566341810848));
#31776=CARTESIAN_POINT('Ctrl Pts',(-41.4138834759049,38.1030067485194,39.5877157505161));
#31777=CARTESIAN_POINT('Ctrl Pts',(-41.445776835455,38.160600201747,39.6187973199473));
#31778=CARTESIAN_POINT('Ctrl Pts',(-41.4768134819625,38.219165709782,39.6489567719273));
#31779=CARTESIAN_POINT('Ctrl Pts',(-41.5069638135077,38.2786474144165,39.6781653411812));
#31780=CARTESIAN_POINT('Ctrl Pts',(-41.5371141450529,38.338129119051,39.707373910435));
#31781=CARTESIAN_POINT('Ctrl Pts',(-41.5663781579772,38.398527013067,39.7356315934182));
#31782=CARTESIAN_POINT('Ctrl Pts',(-41.5947279410512,38.4597834905756,39.7629114387119));
#31783=CARTESIAN_POINT('Ctrl Pts',(-41.6230777241252,38.5210399680844,39.7901912840056));
#31784=CARTESIAN_POINT('Ctrl Pts',(-41.6505132739087,38.5831550216525,39.8164932882995));
#31785=CARTESIAN_POINT('Ctrl Pts',(-41.6770084231115,38.6460694076107,39.8417923654484));
#31786=CARTESIAN_POINT('Ctrl Pts',(-41.7035035723143,38.7089837935689,39.8670914425974));
#31787=CARTESIAN_POINT('Ctrl Pts',(-41.7290583177212,38.7726975042826,39.8913875895315));
#31788=CARTESIAN_POINT('Ctrl Pts',(-41.7536482859026,38.8371497713265,39.9146576332384));
#31789=CARTESIAN_POINT('Ctrl Pts',(-41.778238254084,38.9016020383702,39.9379276769454));
#31790=CARTESIAN_POINT('Ctrl Pts',(-41.8018634420553,38.966792853926,39.9601716146042));
#31791=CARTESIAN_POINT('Ctrl Pts',(-41.8245013167481,39.0326600407391,39.9813682305393));
#31792=CARTESIAN_POINT('Ctrl Pts',(-41.847139191441,39.0985272275523,40.0025648464744));
#31793=CARTESIAN_POINT('Ctrl Pts',(-41.8687897501085,39.1650707776294,40.0227141381135));
#31794=CARTESIAN_POINT('Ctrl Pts',(-41.889432343028,39.2322272235272,40.0417968876091));
#31795=CARTESIAN_POINT('Ctrl Pts',(-41.9100749359475,39.2993836694249,40.0608796371047));
#31796=CARTESIAN_POINT('Ctrl Pts',(-41.9297095606148,39.3671530029904,40.0788958421384));
#31797=CARTESIAN_POINT('Ctrl Pts',(-41.9483174900524,39.4354705876543,40.0958283193379));
#31798=CARTESIAN_POINT('Ctrl Pts',(-41.9669254194899,39.5037881723181,40.1127607965374));
#31799=CARTESIAN_POINT('Ctrl Pts',(-41.9845066514397,39.5726539997901,40.1286095438481));
#31800=CARTESIAN_POINT('Ctrl Pts',(-42.001044417395,39.6420023876939,40.1433594451603));
#31801=CARTESIAN_POINT('Ctrl Pts',(-42.0175821833503,39.7113507755977,40.1581093464725));
#31802=CARTESIAN_POINT('Ctrl Pts',(-42.0330764813043,39.7811817155179,40.1717603999964));
#31803=CARTESIAN_POINT('Ctrl Pts',(-42.0475125332119,39.8514286045806,40.1842995857241));
#31804=CARTESIAN_POINT('Ctrl Pts',(-42.0619485851195,39.9216754936432,40.1968387714518));
#31805=CARTESIAN_POINT('Ctrl Pts',(-42.0753263892288,39.9923383233238,40.2082660878617));
#31806=CARTESIAN_POINT('Ctrl Pts',(-42.0876331861499,40.0633496973136,40.2185706358861));
#31807=CARTESIAN_POINT('Ctrl Pts',(-42.0999509206462,40.1344241821404,40.2288843420019));
#31808=CARTESIAN_POINT('Ctrl Pts',(-42.1111957419127,40.2058478224516,40.2380732818885));
#31809=CARTESIAN_POINT('Ctrl Pts',(-42.1213569049585,40.2775523754548,40.2461286748427));
#31810=CARTESIAN_POINT('Ctrl Pts',(-40.8359764322253,37.3198727723867,39.0942247250269));
#31811=CARTESIAN_POINT('Ctrl Pts',(-40.8765269273983,37.3675681835857,39.134683831424));
#31812=CARTESIAN_POINT('Ctrl Pts',(-40.916359313348,37.4165434422864,39.1743539056441));
#31813=CARTESIAN_POINT('Ctrl Pts',(-40.9554338273102,37.4667496626143,39.21319534935));
#31814=CARTESIAN_POINT('Ctrl Pts',(-40.9945083412725,37.5169558829423,39.2520367930559));
#31815=CARTESIAN_POINT('Ctrl Pts',(-41.0328249780631,37.568393058238,39.2900496010948));
#31816=CARTESIAN_POINT('Ctrl Pts',(-41.0703454863351,37.6210098475309,39.3271958276621));
#31817=CARTESIAN_POINT('Ctrl Pts',(-41.1078659946071,37.6736266368238,39.3643420542294));
#31818=CARTESIAN_POINT('Ctrl Pts',(-41.1445903693819,37.727423033135,39.4006216943967));
#31819=CARTESIAN_POINT('Ctrl Pts',(-41.1804819469606,37.7823453426986,39.4359985305097));
#31820=CARTESIAN_POINT('Ctrl Pts',(-41.2163735245393,37.8372676522623,39.4713753666227));
#31821=CARTESIAN_POINT('Ctrl Pts',(-41.2514323001588,37.8933158677943,39.505849393987));
#31822=CARTESIAN_POINT('Ctrl Pts',(-41.2856232708379,37.9504340497188,39.5393861952759));
#31823=CARTESIAN_POINT('Ctrl Pts',(-41.319814241517,38.0075522316433,39.5729229965647));
#31824=CARTESIAN_POINT('Ctrl Pts',(-41.3531374027178,38.0657403723855,39.6055225673275));
#31825=CARTESIAN_POINT('Ctrl Pts',(-41.3855594819409,38.1249403980169,39.637152359158));
#31826=CARTESIAN_POINT('Ctrl Pts',(-41.4179815611641,38.1841404236482,39.6687821509885));
#31827=CARTESIAN_POINT('Ctrl Pts',(-41.4495025541058,38.2443523263182,39.6994421596887));
#31828=CARTESIAN_POINT('Ctrl Pts',(-41.4800909850681,38.3055160134528,39.7291017706466));
#31829=CARTESIAN_POINT('Ctrl Pts',(-41.5106794160303,38.3666797005875,39.7587613816045));
#31830=CARTESIAN_POINT('Ctrl Pts',(-41.5403352809521,38.4287951640761,39.7874205908828));
#31831=CARTESIAN_POINT('Ctrl Pts',(-41.5690289636793,38.4918004124265,39.8150507786877));
#31832=CARTESIAN_POINT('Ctrl Pts',(-41.5977226464065,38.5548056607768,39.8426809664925));
#31833=CARTESIAN_POINT('Ctrl Pts',(-41.6254541431291,38.618700685634,39.8692821291552));
#31834=CARTESIAN_POINT('Ctrl Pts',(-41.6521957562781,38.6834217200966,39.8948276987528));
#31835=CARTESIAN_POINT('Ctrl Pts',(-41.6789373694272,38.7481427545592,39.9203732683505));
#31836=CARTESIAN_POINT('Ctrl Pts',(-41.7046890954511,38.8136897900448,39.9448632414905));
#31837=CARTESIAN_POINT('Ctrl Pts',(-41.7294252105889,38.8799974112873,39.96827315509));
#31838=CARTESIAN_POINT('Ctrl Pts',(-41.7541613257267,38.9463050325299,39.9916830686895));
#31839=CARTESIAN_POINT('Ctrl Pts',(-41.7778818266912,39.0133732307397,40.014012919641));
#31840=CARTESIAN_POINT('Ctrl Pts',(-41.8005630148243,39.0811350726091,40.0352403984758));
#31841=CARTESIAN_POINT('Ctrl Pts',(-41.8232442029574,39.1488969144785,40.0564678773107));
#31842=CARTESIAN_POINT('Ctrl Pts',(-41.8448860752447,39.2173523910215,40.0765929812073));
#31843=CARTESIAN_POINT('Ctrl Pts',(-41.8654670053889,39.2864331842592,40.0955955988193));
#31844=CARTESIAN_POINT('Ctrl Pts',(-41.8860479355331,39.3555139774971,40.1145982164313));
#31845=CARTESIAN_POINT('Ctrl Pts',(-41.9055679207984,39.4252200782661,40.1324783452289));
#31846=CARTESIAN_POINT('Ctrl Pts',(-41.9240074503906,39.4954819200098,40.1492181120892));
#31847=CARTESIAN_POINT('Ctrl Pts',(-41.9424469799828,39.5657437617536,40.1659578789494));
#31848=CARTESIAN_POINT('Ctrl Pts',(-41.9598060514486,39.636561335155,40.1815572816448));
#31849=CARTESIAN_POINT('Ctrl Pts',(-41.9760673084219,39.7078639636864,40.1960007209425));
#31850=CARTESIAN_POINT('Ctrl Pts',(-41.9923285653951,39.7791665922179,40.2104441602401));
#31851=CARTESIAN_POINT('Ctrl Pts',(-42.007492005711,39.8509542664238,40.2237316342165));
#31852=CARTESIAN_POINT('Ctrl Pts',(-42.0215424620695,39.923155340619,40.2358498486652));
#31853=CARTESIAN_POINT('Ctrl Pts',(-42.0355929184279,39.9953564148142,40.2479680631138));
#31854=CARTESIAN_POINT('Ctrl Pts',(-42.0485303889566,40.0679708794239,40.258917016419));
#31855=CARTESIAN_POINT('Ctrl Pts',(-42.0603419257029,40.14092626235,40.2686857459474));
#31856=CARTESIAN_POINT('Ctrl Pts',(-42.0721639598656,40.2139464838368,40.2784631573623));
#31857=CARTESIAN_POINT('Ctrl Pts',(-42.0828580564471,40.2873082201942,40.2870582449307));
#31858=CARTESIAN_POINT('Ctrl Pts',(-42.092413484143,40.3609381220883,40.2944623765249));
#31859=CARTESIAN_POINT('Ctrl Pts',(-40.7966393248313,37.3211568753947,39.1321088525032));
#31860=CARTESIAN_POINT('Ctrl Pts',(-40.8380807309094,37.3699315504519,39.1735077559943));
#31861=CARTESIAN_POINT('Ctrl Pts',(-40.8787711225811,37.4200447175752,39.2140814723113));
#31862=CARTESIAN_POINT('Ctrl Pts',(-40.9186680157922,37.4714440583024,39.2537876412842));
#31863=CARTESIAN_POINT('Ctrl Pts',(-40.9585649090031,37.5228433990297,39.293493810257));
#31864=CARTESIAN_POINT('Ctrl Pts',(-40.997668297963,37.5755289059027,39.3323324261235));
#31865=CARTESIAN_POINT('Ctrl Pts',(-41.0359373537698,37.6294455773984,39.3702629383271));
#31866=CARTESIAN_POINT('Ctrl Pts',(-41.0742064095767,37.6833622488941,39.4081934505307));
#31867=CARTESIAN_POINT('Ctrl Pts',(-41.1116411266758,37.7385100771898,39.4452158535664));
#31868=CARTESIAN_POINT('Ctrl Pts',(-41.1482024164183,37.7948314923221,39.4812914910072));
#31869=CARTESIAN_POINT('Ctrl Pts',(-41.1847637061608,37.8511529074543,39.5173671284481));
#31870=CARTESIAN_POINT('Ctrl Pts',(-41.2204515632392,37.9086479012521,39.5524959950575));
#31871=CARTESIAN_POINT('Ctrl Pts',(-41.2552287207357,37.9672564552801,39.5866414091118));
#31872=CARTESIAN_POINT('Ctrl Pts',(-41.2900058782322,38.0258650093081,39.620786823166));
#31873=CARTESIAN_POINT('Ctrl Pts',(-41.3238723310975,38.0855871150639,39.6539487797078));
#31874=CARTESIAN_POINT('Ctrl Pts',(-41.3567927118309,38.1463604307069,39.686092648179));
#31875=CARTESIAN_POINT('Ctrl Pts',(-41.3897130925642,38.2071337463499,39.7182365166501));
#31876=CARTESIAN_POINT('Ctrl Pts',(-41.4216873963851,38.2689582630641,39.7493622923831));
#31877=CARTESIAN_POINT('Ctrl Pts',(-41.452682228942,38.3317694455081,39.7794374681786));
#31878=CARTESIAN_POINT('Ctrl Pts',(-41.4836770614989,38.3945806279522,39.809512643974));
#31879=CARTESIAN_POINT('Ctrl Pts',(-41.5136924182901,38.458378467015,39.8385372154639));
#31880=CARTESIAN_POINT('Ctrl Pts',(-41.5426969477387,38.5230963683275,39.8664808665812));
#31881=CARTESIAN_POINT('Ctrl Pts',(-41.5717014771873,38.5878142696401,39.8944245176985));
#31882=CARTESIAN_POINT('Ctrl Pts',(-41.5996951750797,38.6534522238148,39.9212872443838));
#31883=CARTESIAN_POINT('Ctrl Pts',(-41.6266487979873,38.7199417162167,39.9470409849153));
#31884=CARTESIAN_POINT('Ctrl Pts',(-41.6536024208948,38.7864312086186,39.9727947254468));
#31885=CARTESIAN_POINT('Ctrl Pts',(-41.6795159649007,38.853772229603,39.997439476082));
#31886=CARTESIAN_POINT('Ctrl Pts',(-41.7043623557101,38.9218944870306,40.0209494879652));
#31887=CARTESIAN_POINT('Ctrl Pts',(-41.7292087465196,38.9900167444581,40.0444594998485));
#31888=CARTESIAN_POINT('Ctrl Pts',(-41.7529879805209,39.0589202284475,40.0668347695621));
#31889=CARTESIAN_POINT('Ctrl Pts',(-41.775675209024,39.1285330158191,40.088051914823));
#31890=CARTESIAN_POINT('Ctrl Pts',(-41.7983624375271,39.1981458031907,40.1092690600839));
#31891=CARTESIAN_POINT('Ctrl Pts',(-41.8199576572337,39.2684678838435,40.1293280778035));
#31892=CARTESIAN_POINT('Ctrl Pts',(-41.8404382968954,39.3394258534289,40.1482080010584));
#31893=CARTESIAN_POINT('Ctrl Pts',(-41.8609189365571,39.4103838230143,40.1670879243132));
#31894=CARTESIAN_POINT('Ctrl Pts',(-41.8802849931938,39.4819776712398,40.184788750356));
#31895=CARTESIAN_POINT('Ctrl Pts',(-41.898516220103,39.5541326655168,40.2012919713592));
#31896=CARTESIAN_POINT('Ctrl Pts',(-41.9167474470122,39.6262876597936,40.2177951923624));
#31897=CARTESIAN_POINT('Ctrl Pts',(-41.9338438415398,39.6990037896545,40.2331008059224));
#31898=CARTESIAN_POINT('Ctrl Pts',(-41.9497875237805,39.7722051500215,40.2471928019667));
#31899=CARTESIAN_POINT('Ctrl Pts',(-41.9657312060212,39.8454065103885,40.261284798011));
#31900=CARTESIAN_POINT('Ctrl Pts',(-41.9805221736516,39.9190930906431,40.2741631744854));
#31901=CARTESIAN_POINT('Ctrl Pts',(-41.9941449509075,39.9931879713497,40.2858144524841));
#31902=CARTESIAN_POINT('Ctrl Pts',(-42.0077677281635,40.0672828520561,40.2974657304829));
#31903=CARTESIAN_POINT('Ctrl Pts',(-42.0202223130583,40.1417860224648,40.307889908305));
#31904=CARTESIAN_POINT('Ctrl Pts',(-42.0314956662869,40.2166197091016,40.3170760664048));
#31905=CARTESIAN_POINT('Ctrl Pts',(-42.0427790386252,40.2915199036276,40.326270388635));
#31906=CARTESIAN_POINT('Ctrl Pts',(-42.0528790770922,40.3667511912548,40.3342244882568));
#31907=CARTESIAN_POINT('Ctrl Pts',(-42.061785177892,40.4422348971029,40.3409300056503));
#31908=CARTESIAN_POINT('Ctrl Pts',(-40.7572837211926,37.3224193856698,39.1699747890253));
#31909=CARTESIAN_POINT('Ctrl Pts',(-40.7995949415344,37.3722465378174,39.2122892402931));
#31910=CARTESIAN_POINT('Ctrl Pts',(-40.8411220393881,37.4234711881076,39.2537421264551));
#31911=CARTESIAN_POINT('Ctrl Pts',(-40.8818197056895,37.4760374467455,39.2942882194172));
#31912=CARTESIAN_POINT('Ctrl Pts',(-40.9225173719909,37.5286037053833,39.3348343123792));
#31913=CARTESIAN_POINT('Ctrl Pts',(-40.9623856002765,37.5825115640208,39.3744736057022));
#31914=CARTESIAN_POINT('Ctrl Pts',(-41.0013808914287,37.6377022052889,39.4131628500528));
#31915=CARTESIAN_POINT('Ctrl Pts',(-41.0403761825809,37.6928928465569,39.4518520944035));
#31916=CARTESIAN_POINT('Ctrl Pts',(-41.0784985304068,37.7493662616906,39.4895912836375));
#31917=CARTESIAN_POINT('Ctrl Pts',(-41.1157063406701,37.8070608341135,39.5263392415726));
#31918=CARTESIAN_POINT('Ctrl Pts',(-41.1529141509335,37.8647554065364,39.5630871995076));
#31919=CARTESIAN_POINT('Ctrl Pts',(-41.1892074177253,37.9236711270859,39.5988439203076));
#31920=CARTESIAN_POINT('Ctrl Pts',(-41.2245465424691,37.9837437144538,39.6335703908066));
#31921=CARTESIAN_POINT('Ctrl Pts',(-41.2598856672129,38.0438163018217,39.6682968613056));
#31922=CARTESIAN_POINT('Ctrl Pts',(-41.2942706442964,38.1050457464678,39.7019930759885));
#31923=CARTESIAN_POINT('Ctrl Pts',(-41.3276639572251,38.1673652426437,39.7346222698504));
#31924=CARTESIAN_POINT('Ctrl Pts',(-41.3610572701538,38.2296847388195,39.7672514637123));
#31925=CARTESIAN_POINT('Ctrl Pts',(-41.3934589136244,38.2930942766282,39.7988136315712));
#31926=CARTESIAN_POINT('Ctrl Pts',(-41.4248335351027,38.3575246716821,39.8292743368216));
#31927=CARTESIAN_POINT('Ctrl Pts',(-41.4562081565809,38.4219550667359,39.8597350420719));
#31928=CARTESIAN_POINT('Ctrl Pts',(-41.4865557510842,38.4874063088027,39.889094279876));
#31929=CARTESIAN_POINT('Ctrl Pts',(-41.515843207194,38.5538069858481,39.9173200171841));
#31930=CARTESIAN_POINT('Ctrl Pts',(-41.5451306633038,38.6202076628934,39.9455457544922));
#31931=CARTESIAN_POINT('Ctrl Pts',(-41.573357976369,38.687557764372,39.9726379868217));
#31932=CARTESIAN_POINT('Ctrl Pts',(-41.6004943483514,38.7557838064568,39.9985671545895));
#31933=CARTESIAN_POINT('Ctrl Pts',(-41.6276307203338,38.8240098485415,40.0244963223574));
#31934=CARTESIAN_POINT('Ctrl Pts',(-41.6536761469238,38.8931118203972,40.0492624214457));
#31935=CARTESIAN_POINT('Ctrl Pts',(-41.678602210679,38.9630143267796,40.0728384302508));
#31936=CARTESIAN_POINT('Ctrl Pts',(-41.7035282744343,39.032916833162,40.096414439056));
#31937=CARTESIAN_POINT('Ctrl Pts',(-41.7273349713962,39.1036198629696,40.1188003538339));
#31938=CARTESIAN_POINT('Ctrl Pts',(-41.7499963267383,39.1750462740882,40.1399717499339));
#31939=CARTESIAN_POINT('Ctrl Pts',(-41.7726576820804,39.2464726852068,40.1611431460339));
#31940=CARTESIAN_POINT('Ctrl Pts',(-41.7941736922047,39.3186224662897,40.1811000200909));
#31941=CARTESIAN_POINT('Ctrl Pts',(-41.8145208815876,39.3914168967189,40.199820597719));
#31942=CARTESIAN_POINT('Ctrl Pts',(-41.8348680709705,39.4642113271482,40.2185411753471));
#31943=CARTESIAN_POINT('Ctrl Pts',(-41.8540464363803,39.5376503953638,40.2360254535732));
#31944=CARTESIAN_POINT('Ctrl Pts',(-41.872035052837,39.6116539740283,40.2522543557809));
#31945=CARTESIAN_POINT('Ctrl Pts',(-41.8900236692937,39.6856575526928,40.2684832579885));
#31946=CARTESIAN_POINT('Ctrl Pts',(-41.9068225339406,39.7602256300532,40.2834567816001));
#31947=CARTESIAN_POINT('Ctrl Pts',(-41.922413318,39.8352768469571,40.2971585894254));
#31948=CARTESIAN_POINT('Ctrl Pts',(-41.9380041020594,39.910328063861,40.3108603972508));
#31949=CARTESIAN_POINT('Ctrl Pts',(-41.9523868030549,39.98586240839,40.3232904871139));
#31950=CARTESIAN_POINT('Ctrl Pts',(-41.9655457284236,40.0617974671075,40.3344352968825));
#31951=CARTESIAN_POINT('Ctrl Pts',(-41.9787046537923,40.1377325258248,40.3455801066511));
#31952=CARTESIAN_POINT('Ctrl Pts',(-41.9906398014448,40.2140682866706,40.3554396345553));
#31953=CARTESIAN_POINT('Ctrl Pts',(-42.001338149269,40.2907214618238,40.3640031231439));
#31954=CARTESIAN_POINT('Ctrl Pts',(-42.0120460051711,40.3674427619232,40.37257422247));
#31955=CARTESIAN_POINT('Ctrl Pts',(-42.0215148601722,40.4444820285852,40.3798469764035));
#31956=CARTESIAN_POINT('Ctrl Pts',(-42.0297343634969,40.5217550572279,40.3858134344673));
#31957=CARTESIAN_POINT('Ctrl Pts',(-40.7179281175539,37.3236818959449,39.2078407255475));
#31958=CARTESIAN_POINT('Ctrl Pts',(-40.7611091521593,37.374561525183,39.251070724592));
#31959=CARTESIAN_POINT('Ctrl Pts',(-40.8034729561951,37.4268976586399,39.2934027805989));
#31960=CARTESIAN_POINT('Ctrl Pts',(-40.8449713955868,37.4806308351885,39.3347887975501));
#31961=CARTESIAN_POINT('Ctrl Pts',(-40.8864698349786,37.534364011737,39.3761748145014));
#31962=CARTESIAN_POINT('Ctrl Pts',(-40.9271029025901,37.5894942221389,39.4166147852808));
#31963=CARTESIAN_POINT('Ctrl Pts',(-40.9668244290877,37.6459588331793,39.4560627617786));
#31964=CARTESIAN_POINT('Ctrl Pts',(-41.0065459555852,37.7024234442197,39.4955107382762));
#31965=CARTESIAN_POINT('Ctrl Pts',(-41.0453559341377,37.7602224461914,39.5339667137086));
#31966=CARTESIAN_POINT('Ctrl Pts',(-41.0832102649219,37.8192901759049,39.5713869921379));
#31967=CARTESIAN_POINT('Ctrl Pts',(-41.1210645957061,37.8783579056185,39.6088072705671));
#31968=CARTESIAN_POINT('Ctrl Pts',(-41.1579632722114,37.9386943529196,39.6451918455577));
#31969=CARTESIAN_POINT('Ctrl Pts',(-41.1938643642025,38.0002309736275,39.6804993725014));
#31970=CARTESIAN_POINT('Ctrl Pts',(-41.2297654561936,38.0617675943353,39.7158068994451));
#31971=CARTESIAN_POINT('Ctrl Pts',(-41.2646689574953,38.1245043778716,39.7500373722691));
#31972=CARTESIAN_POINT('Ctrl Pts',(-41.2985352026194,38.1883700545804,39.7831518915218));
#31973=CARTESIAN_POINT('Ctrl Pts',(-41.3324014477434,38.2522357312893,39.8162664107745));
#31974=CARTESIAN_POINT('Ctrl Pts',(-41.3652304308637,38.3172302901924,39.8482649707593));
#31975=CARTESIAN_POINT('Ctrl Pts',(-41.3969848412633,38.383279897856,39.8791112054645));
#31976=CARTESIAN_POINT('Ctrl Pts',(-41.428739251663,38.4493295055196,39.9099574401697));
#31977=CARTESIAN_POINT('Ctrl Pts',(-41.4594190838782,38.5164341505905,39.9396513442881));
#31978=CARTESIAN_POINT('Ctrl Pts',(-41.4889894666493,38.5845176033686,39.968159167787));
#31979=CARTESIAN_POINT('Ctrl Pts',(-41.5185598494203,38.6526010561467,39.9966669912859));
#31980=CARTESIAN_POINT('Ctrl Pts',(-41.5470207776582,38.7216633049293,40.0239887292596));
#31981=CARTESIAN_POINT('Ctrl Pts',(-41.5743398987155,38.7916258966968,40.0500933242638));
#31982=CARTESIAN_POINT('Ctrl Pts',(-41.6016590197727,38.8615884884645,40.076197919268));
#31983=CARTESIAN_POINT('Ctrl Pts',(-41.6278363289469,38.9324514111914,40.1010853668093));
#31984=CARTESIAN_POINT('Ctrl Pts',(-41.6528420656479,39.0041341665286,40.1247273725364));
#31985=CARTESIAN_POINT('Ctrl Pts',(-41.677847802349,39.0758169218658,40.1483693782635));
#31986=CARTESIAN_POINT('Ctrl Pts',(-41.7016819622716,39.1483194974918,40.1707659381056));
#31987=CARTESIAN_POINT('Ctrl Pts',(-41.7243174444527,39.2215595323573,40.1918915850447));
#31988=CARTESIAN_POINT('Ctrl Pts',(-41.7469529266338,39.294799567223,40.2130172319838));
#31989=CARTESIAN_POINT('Ctrl Pts',(-41.7683897271757,39.3687770487358,40.2328719623783));
#31990=CARTESIAN_POINT('Ctrl Pts',(-41.7886034662798,39.4434079400089,40.2514331943797));
#31991=CARTESIAN_POINT('Ctrl Pts',(-41.8088172053839,39.5180388312821,40.2699944263809));
#31992=CARTESIAN_POINT('Ctrl Pts',(-41.8278078795668,39.5933231194876,40.2872621567905));
#31993=CARTESIAN_POINT('Ctrl Pts',(-41.845553885571,39.6691752825398,40.3032167402025));
#31994=CARTESIAN_POINT('Ctrl Pts',(-41.8632998915752,39.745027445592,40.3191713236146));
#31995=CARTESIAN_POINT('Ctrl Pts',(-41.8798012263413,39.8214474704518,40.3338127572778));
#31996=CARTESIAN_POINT('Ctrl Pts',(-41.8950391122194,39.8983485438927,40.3471243768842));
#31997=CARTESIAN_POINT('Ctrl Pts',(-41.9102769980975,39.9752496173336,40.3604359964905));
#31998=CARTESIAN_POINT('Ctrl Pts',(-41.9242514324582,40.052631726137,40.3724177997423));
#31999=CARTESIAN_POINT('Ctrl Pts',(-41.9369465059397,40.1304069628652,40.3830561412809));
#32000=CARTESIAN_POINT('Ctrl Pts',(-41.9496415794212,40.2081821995935,40.3936944828194));
#32001=CARTESIAN_POINT('Ctrl Pts',(-41.9610572898313,40.2863505508764,40.4029893608057));
#32002=CARTESIAN_POINT('Ctrl Pts',(-41.971180632251,40.3648232145459,40.410930179883));
#32003=CARTESIAN_POINT('Ctrl Pts',(-41.981312971717,40.4433656202187,40.4188780563049));
#32004=CARTESIAN_POINT('Ctrl Pts',(-41.9901506432521,40.5222128659156,40.4254694645501));
#32005=CARTESIAN_POINT('Ctrl Pts',(-41.9976835491019,40.601275217353,40.4306968632843));
#32006=CARTESIAN_POINT('Ctrl Pts',(-40.6785539801473,37.3249227696823,39.2456884342118));
#32007=CARTESIAN_POINT('Ctrl Pts',(-40.7225836966845,37.3768280462168,39.2898096944072));
#32008=CARTESIAN_POINT('Ctrl Pts',(-40.7657628716283,37.4302491946363,39.3329964106504));
#32009=CARTESIAN_POINT('Ctrl Pts',(-40.8080404421579,37.4851230437161,39.3751975128904));
#32010=CARTESIAN_POINT('Ctrl Pts',(-40.8503180126875,37.5399968927959,39.4173986151304));
#32011=CARTESIAN_POINT('Ctrl Pts',(-40.8916939709274,37.5963234323158,39.4586140955063));
#32012=CARTESIAN_POINT('Ctrl Pts',(-40.9321193846504,37.654036057902,39.4987952130883));
#32013=CARTESIAN_POINT('Ctrl Pts',(-40.9725447983734,37.7117486834884,39.5389763306701));
#32014=CARTESIAN_POINT('Ctrl Pts',(-41.0120196600483,37.7708473843928,39.5781230779729));
#32015=CARTESIAN_POINT('Ctrl Pts',(-41.0504972836104,37.8312622803774,39.6161891583012));
#32016=CARTESIAN_POINT('Ctrl Pts',(-41.0889749071725,37.891677176362,39.6542552386296));
#32017=CARTESIAN_POINT('Ctrl Pts',(-41.1264552854528,37.9534082561759,39.6912406448916));
#32018=CARTESIAN_POINT('Ctrl Pts',(-41.1628940888185,38.0163825287324,39.7271016339729));
#32019=CARTESIAN_POINT('Ctrl Pts',(-41.1993328921841,38.0793568012888,39.7629626230543));
#32020=CARTESIAN_POINT('Ctrl Pts',(-41.234730113845,38.1435742548608,39.7976991882729));
#32021=CARTESIAN_POINT('Ctrl Pts',(-41.2690438853101,38.2089589598693,39.8312702434172));
#32022=CARTESIAN_POINT('Ctrl Pts',(-41.3033576567751,38.2743436648777,39.8648412985615));
#32023=CARTESIAN_POINT('Ctrl Pts',(-41.3365879716492,38.3408956091474,39.897246837375));
#32024=CARTESIAN_POINT('Ctrl Pts',(-41.3686955214862,38.4085361038988,39.9284485276018));
#32025=CARTESIAN_POINT('Ctrl Pts',(-41.4008030713232,38.4761765986501,39.9596502178287));
#32026=CARTESIAN_POINT('Ctrl Pts',(-41.4317878501381,38.5449056312883,39.9896480536529));
#32027=CARTESIAN_POINT('Ctrl Pts',(-41.4616132023931,38.614641939638,40.0184065473303));
#32028=CARTESIAN_POINT('Ctrl Pts',(-41.4914385546482,38.6843782479877,40.0471650410077));
#32029=CARTESIAN_POINT('Ctrl Pts',(-41.5201044747827,38.755121819064,40.0746841871765));
#32030=CARTESIAN_POINT('Ctrl Pts',(-41.5475770467723,38.8267890091748,40.1009314264494));
#32031=CARTESIAN_POINT('Ctrl Pts',(-41.5750496187618,38.8984561992857,40.1271786657222));
#32032=CARTESIAN_POINT('Ctrl Pts',(-41.6013288374831,38.9710469950868,40.1521539932042));
#32033=CARTESIAN_POINT('Ctrl Pts',(-41.6263836065667,39.044475568871,40.1758278548012));
#32034=CARTESIAN_POINT('Ctrl Pts',(-41.6514383756503,39.1179041426551,40.1995017163983));
#32035=CARTESIAN_POINT('Ctrl Pts',(-41.6752686904225,39.1921704807498,40.2218741076939));
#32036=CARTESIAN_POINT('Ctrl Pts',(-41.6978463476587,39.2671867740911,40.2429185497343));
#32037=CARTESIAN_POINT('Ctrl Pts',(-41.7204240048949,39.3422030674324,40.2639629917746));
#32038=CARTESIAN_POINT('Ctrl Pts',(-41.7417490003819,39.417969302052,40.2836794806318));
#32039=CARTESIAN_POINT('Ctrl Pts',(-41.7617960907045,39.4943958948663,40.3020446750837));
#32040=CARTESIAN_POINT('Ctrl Pts',(-41.781843181027,39.5708224876806,40.3204098695356));
#32041=CARTESIAN_POINT('Ctrl Pts',(-41.8006123624423,39.6479094244583,40.3374237661525));
#32042=CARTESIAN_POINT('Ctrl Pts',(-41.818081411026,39.7255655596244,40.353066216633));
#32043=CARTESIAN_POINT('Ctrl Pts',(-41.8355504596097,39.8032216947905,40.3687086671135));
#32044=CARTESIAN_POINT('Ctrl Pts',(-41.8517193720981,39.8814470138844,40.3829796685342));
#32045=CARTESIAN_POINT('Ctrl Pts',(-41.8665689966161,39.9601490240587,40.3958623131708));
#32046=CARTESIAN_POINT('Ctrl Pts',(-41.8814186211341,40.0388510342329,40.4087449578074));
#32047=CARTESIAN_POINT('Ctrl Pts',(-41.8949489549049,40.1180297208319,40.4202392432495));
#32048=CARTESIAN_POINT('Ctrl Pts',(-41.9071439634125,40.1975914621405,40.4303315423613));
#32049=CARTESIAN_POINT('Ctrl Pts',(-41.9193389719201,40.277153203449,40.440423841473));
#32050=CARTESIAN_POINT('Ctrl Pts',(-41.9301986528813,40.3570979846507,40.4491141523626));
#32051=CARTESIAN_POINT('Ctrl Pts',(-41.9397101270951,40.4373312762363,40.4563921607536));
#32052=CARTESIAN_POINT('Ctrl Pts',(-41.9492300545616,40.5176358745705,40.4636766374209));
#32053=CARTESIAN_POINT('Ctrl Pts',(-41.9573993760106,40.5982294813707,40.4695462987562));
#32054=CARTESIAN_POINT('Ctrl Pts',(-41.9642083721993,40.6790166284688,40.4739941491783));
#32055=CARTESIAN_POINT('Ctrl Pts',(-40.6391656485255,37.3261470729264,39.2835221829441));
#32056=CARTESIAN_POINT('Ctrl Pts',(-40.6840266281348,37.3790556848234,39.3285143662084));
#32057=CARTESIAN_POINT('Ctrl Pts',(-40.7280035489272,37.4335399036566,39.3725351780446));
#32058=CARTESIAN_POINT('Ctrl Pts',(-40.7710423171585,37.4895327111958,39.4155304707204));
#32059=CARTESIAN_POINT('Ctrl Pts',(-40.8140810853897,37.5455255187351,39.4585257633961));
#32060=CARTESIAN_POINT('Ctrl Pts',(-40.8561816923719,37.6030269036775,39.5004955282322));
#32061=CARTESIAN_POINT('Ctrl Pts',(-40.8972923523177,37.6619661365324,39.5413881403836));
#32062=CARTESIAN_POINT('Ctrl Pts',(-40.9384030122634,37.7209053693873,39.5822807525349));
#32063=CARTESIAN_POINT('Ctrl Pts',(-40.9785237168741,37.7812824382571,39.6220962037469));
#32064=CARTESIAN_POINT('Ctrl Pts',(-41.0176051157382,37.8430230764203,39.6607855190843));
#32065=CARTESIAN_POINT('Ctrl Pts',(-41.0566865146023,37.9047637145835,39.6994748344218));
#32066=CARTESIAN_POINT('Ctrl Pts',(-41.0947285998308,37.9678679095771,39.7370380060749));
#32067=CARTESIAN_POINT('Ctrl Pts',(-41.1316845778148,38.0322580401824,39.7734288295218));
#32068=CARTESIAN_POINT('Ctrl Pts',(-41.1686405557988,38.0966481707877,39.8098196529687));
#32069=CARTESIAN_POINT('Ctrl Pts',(-41.2045104190784,38.1623242240067,39.8450381208633));
#32070=CARTESIAN_POINT('Ctrl Pts',(-41.2392500459829,38.2292054151105,39.8790409127831));
#32071=CARTESIAN_POINT('Ctrl Pts',(-41.2739896728873,38.2960866062143,39.9130437047028));
#32072=CARTESIAN_POINT('Ctrl Pts',(-41.3075990564042,38.364172921702,39.9458308137839));
#32073=CARTESIAN_POINT('Ctrl Pts',(-41.3400368553625,38.4333806121052,39.9773619102927));
#32074=CARTESIAN_POINT('Ctrl Pts',(-41.3724746543208,38.5025883025084,40.0088930068016));
#32075=CARTESIAN_POINT('Ctrl Pts',(-41.4037408621726,38.5729173538569,40.0391680843732));
#32076=CARTESIAN_POINT('Ctrl Pts',(-41.4337970199666,38.6442812580081,40.0681499031948));
#32077=CARTESIAN_POINT('Ctrl Pts',(-41.4638531777607,38.7156451621594,40.0971317220163));
#32078=CARTESIAN_POINT('Ctrl Pts',(-41.4926992794298,38.7880439047079,40.1248202762375));
#32079=CARTESIAN_POINT('Ctrl Pts',(-41.5202998428706,38.861388431691,40.1511815075944));
#32080=CARTESIAN_POINT('Ctrl Pts',(-41.5479004063115,38.9347329586739,40.1775427389512));
#32081=CARTESIAN_POINT('Ctrl Pts',(-41.5742554259526,39.009023255286,40.2025766421226));
#32082=CARTESIAN_POINT('Ctrl Pts',(-41.5993324838422,39.084167940861,40.2262524241938));
#32083=CARTESIAN_POINT('Ctrl Pts',(-41.6244095417318,39.1593126264361,40.2499282062651));
#32084=CARTESIAN_POINT('Ctrl Pts',(-41.648208632808,39.2353116858053,40.2722458624571));
#32085=CARTESIAN_POINT('Ctrl Pts',(-41.6707004830348,39.3120716364419,40.2931779409709));
#32086=CARTESIAN_POINT('Ctrl Pts',(-41.6931923332617,39.3888315870784,40.3141100194848));
#32087=CARTESIAN_POINT('Ctrl Pts',(-41.7143769380992,39.4663524134872,40.3336565160952));
#32088=CARTESIAN_POINT('Ctrl Pts',(-41.7342282394564,39.5445387612942,40.3517933876636));
#32089=CARTESIAN_POINT('Ctrl Pts',(-41.7540795408135,39.6227251091012,40.3699302592321));
#32090=CARTESIAN_POINT('Ctrl Pts',(-41.7725975346832,39.7015769625234,40.3866575020975));
#32091=CARTESIAN_POINT('Ctrl Pts',(-41.7897594430353,39.7809973299591,40.4019545409404));
#32092=CARTESIAN_POINT('Ctrl Pts',(-41.8069213513874,39.8604176973947,40.4172515797833));
#32093=CARTESIAN_POINT('Ctrl Pts',(-41.8227271707575,39.9404065628119,40.4311184115157));
#32094=CARTESIAN_POINT('Ctrl Pts',(-41.8371574592217,40.0208655360286,40.4435379792625));
#32095=CARTESIAN_POINT('Ctrl Pts',(-41.8515877476859,40.1013245092453,40.4559575470093));
#32096=CARTESIAN_POINT('Ctrl Pts',(-41.8646425023312,40.18225357402,40.4669298482633));
#32097=CARTESIAN_POINT('Ctrl Pts',(-41.8763056651767,40.2635531836801,40.4764413865623));
#32098=CARTESIAN_POINT('Ctrl Pts',(-41.8879688280222,40.3448527933402,40.4859529248613));
#32099=CARTESIAN_POINT('Ctrl Pts',(-41.8982403967134,40.4265229314745,40.4940036982851));
#32100=CARTESIAN_POINT('Ctrl Pts',(-41.9071077367231,40.5084631398541,40.5005838039923));
#32101=CARTESIAN_POINT('Ctrl Pts',(-41.915982957516,40.5904761719918,40.5071697577201));
#32102=CARTESIAN_POINT('Ctrl Pts',(-41.9234514507292,40.6727597380641,40.5122824271486));
#32103=CARTESIAN_POINT('Ctrl Pts',(-41.9295040118784,40.755212445608,40.5159155106514));
#32104=CARTESIAN_POINT('Ctrl Pts',(-40.5997773169037,37.3273713761706,39.3213559316764));
#32105=CARTESIAN_POINT('Ctrl Pts',(-40.6454695595851,37.38128332343,39.3672190380096));
#32106=CARTESIAN_POINT('Ctrl Pts',(-40.6902442262262,37.4368306126769,39.4120739454389));
#32107=CARTESIAN_POINT('Ctrl Pts',(-40.734044192159,37.4939423786756,39.4558634285503));
#32108=CARTESIAN_POINT('Ctrl Pts',(-40.7778441580919,37.5510541446742,39.4996529116618));
#32109=CARTESIAN_POINT('Ctrl Pts',(-40.8206694138164,37.6097303750392,39.5423769609582));
#32110=CARTESIAN_POINT('Ctrl Pts',(-40.862465319985,37.6698962151627,39.583981067679));
#32111=CARTESIAN_POINT('Ctrl Pts',(-40.9042612261534,37.7300620552863,39.6255851743997));
#32112=CARTESIAN_POINT('Ctrl Pts',(-40.9450277736999,37.7917174921214,39.6660693295208));
#32113=CARTESIAN_POINT('Ctrl Pts',(-40.984712947866,37.8547838724632,39.7053818798674));
#32114=CARTESIAN_POINT('Ctrl Pts',(-41.024398122032,37.9178502528052,39.7446944302139));
#32115=CARTESIAN_POINT('Ctrl Pts',(-41.0630019142087,37.9823275629784,39.7828353672583));
#32116=CARTESIAN_POINT('Ctrl Pts',(-41.1004750668111,38.0481335516325,39.8197560250706));
#32117=CARTESIAN_POINT('Ctrl Pts',(-41.1379482194135,38.1139395402866,39.856676682883));
#32118=CARTESIAN_POINT('Ctrl Pts',(-41.1742907243117,38.1810741931526,39.8923770534537));
#32119=CARTESIAN_POINT('Ctrl Pts',(-41.2094562066557,38.2494518703517,39.926811582149));
#32120=CARTESIAN_POINT('Ctrl Pts',(-41.2446216889996,38.3178295475508,39.9612461108442));
#32121=CARTESIAN_POINT('Ctrl Pts',(-41.2786101411592,38.3874502342565,39.9944147901928));
#32122=CARTESIAN_POINT('Ctrl Pts',(-41.3113781892388,38.4582251203117,40.0262752929836));
#32123=CARTESIAN_POINT('Ctrl Pts',(-41.3441462373184,38.5290000063668,40.0581357957744));
#32124=CARTESIAN_POINT('Ctrl Pts',(-41.3756938742071,38.6009290764255,40.0886881150935));
#32125=CARTESIAN_POINT('Ctrl Pts',(-41.4059808375401,38.6739205763783,40.1178932590592));
#32126=CARTESIAN_POINT('Ctrl Pts',(-41.4362678008732,38.7469120763311,40.147098403025));
#32127=CARTESIAN_POINT('Ctrl Pts',(-41.4652940840769,38.820965990352,40.1749563652985));
#32128=CARTESIAN_POINT('Ctrl Pts',(-41.493022638969,38.8959878542071,40.2014315887393));
#32129=CARTESIAN_POINT('Ctrl Pts',(-41.5207511938611,38.9710097180622,40.2279068121803));
#32130=CARTESIAN_POINT('Ctrl Pts',(-41.547182014422,39.0469995154852,40.252999291041));
#32131=CARTESIAN_POINT('Ctrl Pts',(-41.5722813611177,39.1238603128512,40.2766769935864));
#32132=CARTESIAN_POINT('Ctrl Pts',(-41.5973807078133,39.2007211102171,40.3003546961319));
#32133=CARTESIAN_POINT('Ctrl Pts',(-41.6211485751934,39.2784528908609,40.3226176172202));
#32134=CARTESIAN_POINT('Ctrl Pts',(-41.643554618411,39.3569564987926,40.3434373322076));
#32135=CARTESIAN_POINT('Ctrl Pts',(-41.6659606616286,39.4354601067243,40.3642570471951));
#32136=CARTESIAN_POINT('Ctrl Pts',(-41.6870048758165,39.5147355249225,40.3836335515585));
#32137=CARTESIAN_POINT('Ctrl Pts',(-41.7066603882083,39.5946816277222,40.4015421002435));
#32138=CARTESIAN_POINT('Ctrl Pts',(-41.7263159006,39.6746277305219,40.4194506489285));
#32139=CARTESIAN_POINT('Ctrl Pts',(-41.7445827069242,39.7552445005886,40.4358912380425));
#32140=CARTESIAN_POINT('Ctrl Pts',(-41.7614374750446,39.8364291002939,40.4508428652477));
#32141=CARTESIAN_POINT('Ctrl Pts',(-41.778292243165,39.9176136999991,40.4657944924529));
#32142=CARTESIAN_POINT('Ctrl Pts',(-41.7937349694168,39.9993661117394,40.4792571544972));
#32143=CARTESIAN_POINT('Ctrl Pts',(-41.8077459218272,40.0815820479985,40.4912136453542));
#32144=CARTESIAN_POINT('Ctrl Pts',(-41.8217568742376,40.1637979842576,40.5031701362111));
#32145=CARTESIAN_POINT('Ctrl Pts',(-41.8343360497575,40.246477427208,40.5136204532771));
#32146=CARTESIAN_POINT('Ctrl Pts',(-41.8454673669409,40.3295149052198,40.5225512307633));
#32147=CARTESIAN_POINT('Ctrl Pts',(-41.8565986841243,40.4125523832314,40.5314820082495));
#32148=CARTESIAN_POINT('Ctrl Pts',(-41.8662821405455,40.4959478782984,40.5388932442076));
#32149=CARTESIAN_POINT('Ctrl Pts',(-41.8745053463511,40.5795950034718,40.544775447231));
#32150=CARTESIAN_POINT('Ctrl Pts',(-41.8827358604704,40.6633164694133,40.5506628780192));
#32151=CARTESIAN_POINT('Ctrl Pts',(-41.8895035254478,40.7472899947576,40.5550185555409));
#32152=CARTESIAN_POINT('Ctrl Pts',(-41.8947996515575,40.8314082627473,40.5578368721246));
#32153=CARTESIAN_POINT('Ctrl Pts',(-40.5603747681421,37.3285790821591,39.3591756979305));
#32154=CARTESIAN_POINT('Ctrl Pts',(-40.6068808335252,37.3834720268057,39.4058893665872));
#32155=CARTESIAN_POINT('Ctrl Pts',(-40.6524355994228,37.440060415916,39.4515577822779));
#32156=CARTESIAN_POINT('Ctrl Pts',(-40.6969788080551,37.4982694003275,39.4961205382474));
#32157=CARTESIAN_POINT('Ctrl Pts',(-40.7415220166874,37.556478384739,39.5406832942169));
#32158=CARTESIAN_POINT('Ctrl Pts',(-40.7850536576694,37.6163079508829,39.5841403800759));
#32159=CARTESIAN_POINT('Ctrl Pts',(-40.8275161474155,37.6776789650634,39.626434312041));
#32160=CARTESIAN_POINT('Ctrl Pts',(-40.8699786371616,37.7390499792439,39.668728244006));
#32161=CARTESIAN_POINT('Ctrl Pts',(-40.9113719657712,37.8019624271558,39.7098590122159));
#32162=CARTESIAN_POINT('Ctrl Pts',(-40.9516413760227,37.8663330996633,39.7497722077611));
#32163=CARTESIAN_POINT('Ctrl Pts',(-40.9919107862741,37.9307037721708,39.7896854033063));
#32164=CARTESIAN_POINT('Ctrl Pts',(-41.0310562687772,37.9965326542701,39.82838101688));
#32165=CARTESIAN_POINT('Ctrl Pts',(-41.0690260373813,38.0637326812403,39.8658078582303));
#32166=CARTESIAN_POINT('Ctrl Pts',(-41.1069958059855,38.1309327082104,39.9032346995806));
#32167=CARTESIAN_POINT('Ctrl Pts',(-41.1437898518358,38.1995038643887,39.9393927599795));
#32168=CARTESIAN_POINT('Ctrl Pts',(-41.1793594967149,38.2693554595067,39.9742342031185));
#32169=CARTESIAN_POINT('Ctrl Pts',(-41.2149291415941,38.3392070546247,40.0090756462575));
#32170=CARTESIAN_POINT('Ctrl Pts',(-41.2492743772058,38.4103390724019,40.0426004640103));
#32171=CARTESIAN_POINT('Ctrl Pts',(-41.282349761923,38.4826574366354,40.0747643004416));
#32172=CARTESIAN_POINT('Ctrl Pts',(-41.3154251466403,38.5549758008688,40.106928136873));
#32173=CARTESIAN_POINT('Ctrl Pts',(-41.3472306727472,38.6284804947033,40.1377309844799));
#32174=CARTESIAN_POINT('Ctrl Pts',(-41.3777242553182,38.7030743045571,40.1671320849417));
#32175=CARTESIAN_POINT('Ctrl Pts',(-41.4082178378893,38.7776681144109,40.1965331854034));
#32176=CARTESIAN_POINT('Ctrl Pts',(-41.4373994698095,38.8533510228988,40.2245325318599));
#32177=CARTESIAN_POINT('Ctrl Pts',(-41.4652305341039,38.9300229359037,40.2510930713476));
#32178=CARTESIAN_POINT('Ctrl Pts',(-41.4930615983982,39.0066948489086,40.2776536108352));
#32179=CARTESIAN_POINT('Ctrl Pts',(-41.5195420885715,39.0843557485611,40.3027753371549));
#32180=CARTESIAN_POINT('Ctrl Pts',(-41.5446369576921,39.1629029246618,40.3264250006599));
#32181=CARTESIAN_POINT('Ctrl Pts',(-41.5697318268126,39.2414501007626,40.3500746641649));
#32182=CARTESIAN_POINT('Ctrl Pts',(-41.593441069022,39.3208835350051,40.3722522593337));
#32183=CARTESIAN_POINT('Ctrl Pts',(-41.6157333000996,39.4010981724733,40.3929284277542));
#32184=CARTESIAN_POINT('Ctrl Pts',(-41.6380255311772,39.4813128099415,40.4136045961748));
#32185=CARTESIAN_POINT('Ctrl Pts',(-41.6589007459169,39.5623086319402,40.4327793330178));
#32186=CARTESIAN_POINT('Ctrl Pts',(-41.6783313058059,39.6439785163979,40.4504272487505));
#32187=CARTESIAN_POINT('Ctrl Pts',(-41.697761865695,39.7256484008556,40.4680751644832));
#32188=CARTESIAN_POINT('Ctrl Pts',(-41.7157477661934,39.8079923287374,40.4841962549813));
#32189=CARTESIAN_POINT('Ctrl Pts',(-41.7322651876043,39.8909013938422,40.4987691667571));
#32190=CARTESIAN_POINT('Ctrl Pts',(-41.7487826090152,39.973810458947,40.513342078533));
#32191=CARTESIAN_POINT('Ctrl Pts',(-41.7638315474766,40.0572846419505,40.5263668081778));
#32192=CARTESIAN_POINT('Ctrl Pts',(-41.7773920651324,40.1412135402639,40.537826094759));
#32193=CARTESIAN_POINT('Ctrl Pts',(-41.7909525827882,40.2251424385774,40.5492853813402));
#32194=CARTESIAN_POINT('Ctrl Pts',(-41.8030246764649,40.3095260326383,40.5591792221737));
#32195=CARTESIAN_POINT('Ctrl Pts',(-41.8135923429232,40.3942527151709,40.5674944945855));
#32196=CARTESIAN_POINT('Ctrl Pts',(-41.8241600093816,40.4789793977035,40.5758097669973));
#32197=CARTESIAN_POINT('Ctrl Pts',(-41.8332232461447,40.5640491489585,40.5825464690351));
#32198=CARTESIAN_POINT('Ctrl Pts',(-41.8407700269778,40.6493494518621,40.5876956510615));
#32199=CARTESIAN_POINT('Ctrl Pts',(-41.848323514957,40.7347255647833,40.5928494093856));
#32200=CARTESIAN_POINT('Ctrl Pts',(-41.8543578485532,40.8203326194182,40.5964128234335));
#32201=CARTESIAN_POINT('Ctrl Pts',(-41.858864989028,40.9060571842964,40.5983811276797));
#32202=CARTESIAN_POINT('Ctrl Pts',(-40.5209614242509,37.3297741857869,39.3969848472346));
#32203=CARTESIAN_POINT('Ctrl Pts',(-40.5682667277247,37.3856292560404,39.4445317407691));
#32204=CARTESIAN_POINT('Ctrl Pts',(-40.614586797881,37.4432402480706,39.4909960961139));
#32205=CARTESIAN_POINT('Ctrl Pts',(-40.6598581425081,37.502528192884,39.5363142232817));
#32206=CARTESIAN_POINT('Ctrl Pts',(-40.7051294871352,37.5618161376976,39.5816323504493));
#32207=CARTESIAN_POINT('Ctrl Pts',(-40.7493520948838,37.6227810204313,39.625804238079));
#32208=CARTESIAN_POINT('Ctrl Pts',(-40.7924653485924,37.6853392748206,39.6687693385324));
#32209=CARTESIAN_POINT('Ctrl Pts',(-40.835578602301,37.7478975292098,39.7117344389858));
#32210=CARTESIAN_POINT('Ctrl Pts',(-40.8775824911613,37.8120491395717,39.7534927414919));
#32211=CARTESIAN_POINT('Ctrl Pts',(-40.9184194392716,37.8777061715048,39.7939870067811));
#32212=CARTESIAN_POINT('Ctrl Pts',(-40.9592563873819,37.9433632034379,39.8344812720702));
#32213=CARTESIAN_POINT('Ctrl Pts',(-40.9989263845046,38.0105256404827,39.8737114899907));
#32214=CARTESIAN_POINT('Ctrl Pts',(-41.0373750538685,38.0791014212136,39.911623886589));
#32215=CARTESIAN_POINT('Ctrl Pts',(-41.0758237232324,38.1476772019446,39.9495362831873));
#32216=CARTESIAN_POINT('Ctrl Pts',(-41.1130510551986,38.2176663091703,39.986130848959));
#32217=CARTESIAN_POINT('Ctrl Pts',(-41.1490060212252,38.2889728068698,40.0213574227123));
#32218=CARTESIAN_POINT('Ctrl Pts',(-41.1849609872517,38.3602793045694,40.0565839964655));
#32219=CARTESIAN_POINT('Ctrl Pts',(-41.219643578325,38.4329031748667,40.0904425693693));
#32220=CARTESIAN_POINT('Ctrl Pts',(-41.2530062540501,38.5067448701977,40.1228867305336));
#32221=CARTESIAN_POINT('Ctrl Pts',(-41.2863689297752,38.5805865655286,40.1553308916979));
#32222=CARTESIAN_POINT('Ctrl Pts',(-41.3184116817886,38.6556460673815,40.1863606329891));
#32223=CARTESIAN_POINT('Ctrl Pts',(-41.3490905881962,38.7318204896042,40.2159334210757));
#32224=CARTESIAN_POINT('Ctrl Pts',(-41.379769494604,38.8079949118268,40.2455062091623));
#32225=CARTESIAN_POINT('Ctrl Pts',(-41.4090845477151,38.8852842353228,40.2736220366305));
#32226=CARTESIAN_POINT('Ctrl Pts',(-41.4369955645689,38.9635825174611,40.3002423643315));
#32227=CARTESIAN_POINT('Ctrl Pts',(-41.4649065814228,39.0418807995995,40.3268626920326));
#32228=CARTESIAN_POINT('Ctrl Pts',(-41.4914135550221,39.1211880207514,40.3519875132929));
#32229=CARTESIAN_POINT('Ctrl Pts',(-41.5164801515192,39.2013954722972,40.3755823888195));
#32230=CARTESIAN_POINT('Ctrl Pts',(-41.5415467480163,39.281602923843,40.3991772643461));
#32231=CARTESIAN_POINT('Ctrl Pts',(-41.565172961127,39.3627105856755,40.4212421882239));
#32232=CARTESIAN_POINT('Ctrl Pts',(-41.5873264057423,39.4446072812604,40.4417469154463));
#32233=CARTESIAN_POINT('Ctrl Pts',(-41.6094798503576,39.5265039768455,40.4622516426688));
#32234=CARTESIAN_POINT('Ctrl Pts',(-41.6301605209237,39.6091896856524,40.4811961680955));
#32235=CARTESIAN_POINT('Ctrl Pts',(-41.6493400698688,39.6925510680742,40.4985545239373));
#32236=CARTESIAN_POINT('Ctrl Pts',(-41.6685196188139,39.7759124504959,40.5159128797791));
#32237=CARTESIAN_POINT('Ctrl Pts',(-41.6861980413298,39.8599494856346,40.5316850616842));
#32238=CARTESIAN_POINT('Ctrl Pts',(-41.7023511051097,39.9445469815827,40.5458494502833));
#32239=CARTESIAN_POINT('Ctrl Pts',(-41.7185041688897,40.0291444775307,40.5600138388823));
#32240=CARTESIAN_POINT('Ctrl Pts',(-41.7331318698843,40.1143024130801,40.5725704306242));
#32241=CARTESIAN_POINT('Ctrl Pts',(-41.7462141574959,40.1999040598739,40.5835020138387));
#32242=CARTESIAN_POINT('Ctrl Pts',(-41.7592964451075,40.2855057066677,40.5944335970531));
#32243=CARTESIAN_POINT('Ctrl Pts',(-41.7708333160563,40.3715510432463,40.6037401689996));
#32244=CARTESIAN_POINT('Ctrl Pts',(-41.7808089564319,40.4579221248672,40.6114089729004));
#32245=CARTESIAN_POINT('Ctrl Pts',(-41.7907845968073,40.5442932064881,40.6190777768011));
#32246=CARTESIAN_POINT('Ctrl Pts',(-41.7991990041087,40.6309900114988,40.6251088107337));
#32247=CARTESIAN_POINT('Ctrl Pts',(-41.806040644473,40.7178937021711,40.6294938077917));
#32248=CARTESIAN_POINT('Ctrl Pts',(-41.812888365295,40.8048746278599,40.6338827019837));
#32249=CARTESIAN_POINT('Ctrl Pts',(-41.8181605206493,40.8920627852852,40.6366226310933));
#32250=CARTESIAN_POINT('Ctrl Pts',(-41.8218498690737,40.9793384509368,40.6377098307341));
#32251=CARTESIAN_POINT('Ctrl Pts',(-40.4815480803598,37.3309692894148,39.4347939965387));
#32252=CARTESIAN_POINT('Ctrl Pts',(-40.5296526219241,37.3877864852751,39.4831741149509));
#32253=CARTESIAN_POINT('Ctrl Pts',(-40.5767379963392,37.4464200802252,39.53043440995));
#32254=CARTESIAN_POINT('Ctrl Pts',(-40.6227374769611,37.5067869854406,39.5765079083159));
#32255=CARTESIAN_POINT('Ctrl Pts',(-40.668736957583,37.567153890656,39.6225814066818));
#32256=CARTESIAN_POINT('Ctrl Pts',(-40.7136505320982,37.6292540899798,39.667468096082));
#32257=CARTESIAN_POINT('Ctrl Pts',(-40.7574145497693,37.6929995845778,39.7111043650238));
#32258=CARTESIAN_POINT('Ctrl Pts',(-40.8011785674403,37.7567450791758,39.7547406339656));
#32259=CARTESIAN_POINT('Ctrl Pts',(-40.8437930165514,37.8221358519875,39.7971264707679));
#32260=CARTESIAN_POINT('Ctrl Pts',(-40.8851975025205,37.8890792433462,39.838201805801));
#32261=CARTESIAN_POINT('Ctrl Pts',(-40.9266019884896,37.956022634705,39.8792771408341));
#32262=CARTESIAN_POINT('Ctrl Pts',(-40.966796500232,38.0245186266951,39.9190419631016));
#32263=CARTESIAN_POINT('Ctrl Pts',(-41.0057240703556,38.0944701611869,39.9574399149478));
#32264=CARTESIAN_POINT('Ctrl Pts',(-41.0446516404792,38.1644216956787,39.9958378667941));
#32265=CARTESIAN_POINT('Ctrl Pts',(-41.0823122585615,38.2358287539518,40.0328689379385));
#32266=CARTESIAN_POINT('Ctrl Pts',(-41.1186525457355,38.308590154233,40.068480642306));
#32267=CARTESIAN_POINT('Ctrl Pts',(-41.1549928329094,38.3813515545141,40.1040923466735));
#32268=CARTESIAN_POINT('Ctrl Pts',(-41.1900127794441,38.4554672773316,40.1382846747284));
#32269=CARTESIAN_POINT('Ctrl Pts',(-41.2236627461772,38.53083230376,40.1710091606256));
#32270=CARTESIAN_POINT('Ctrl Pts',(-41.2573127129103,38.6061973301884,40.2037336465228));
#32271=CARTESIAN_POINT('Ctrl Pts',(-41.2895926908299,38.6828116400597,40.2349902814984));
#32272=CARTESIAN_POINT('Ctrl Pts',(-41.3204569210743,38.7605666746512,40.2647347572098));
#32273=CARTESIAN_POINT('Ctrl Pts',(-41.3513211513187,38.8383217092427,40.2944792329211));
#32274=CARTESIAN_POINT('Ctrl Pts',(-41.3807696256207,38.9172174477468,40.322711541401));
#32275=CARTESIAN_POINT('Ctrl Pts',(-41.408760595034,38.9971420990185,40.3493916573154));
#32276=CARTESIAN_POINT('Ctrl Pts',(-41.4367515644473,39.0770667502903,40.3760717732299));
#32277=CARTESIAN_POINT('Ctrl Pts',(-41.4632850214728,39.1580202929416,40.4011996894309));
#32278=CARTESIAN_POINT('Ctrl Pts',(-41.4883233453464,39.2398880199326,40.4247397769792));
#32279=CARTESIAN_POINT('Ctrl Pts',(-41.51336166922,39.3217557469235,40.4482798645274));
#32280=CARTESIAN_POINT('Ctrl Pts',(-41.5369048532321,39.4045376363458,40.4702321171141));
#32281=CARTESIAN_POINT('Ctrl Pts',(-41.558919511385,39.4881163900476,40.4905654031384));
#32282=CARTESIAN_POINT('Ctrl Pts',(-41.580934169538,39.5716951437495,40.5108986891627));
#32283=CARTESIAN_POINT('Ctrl Pts',(-41.6014202959306,39.6560707393645,40.5296130031733));
#32284=CARTESIAN_POINT('Ctrl Pts',(-41.6203488339317,39.7411236197504,40.5466817991241));
#32285=CARTESIAN_POINT('Ctrl Pts',(-41.6392773719328,39.8261765001363,40.5637505950749));
#32286=CARTESIAN_POINT('Ctrl Pts',(-41.6566483164661,39.9119066425318,40.5791738683872));
#32287=CARTESIAN_POINT('Ctrl Pts',(-41.6724370226152,39.9981925693231,40.5929297338094));
#32288=CARTESIAN_POINT('Ctrl Pts',(-41.6882257287643,40.0844784961144,40.6066855992316));
#32289=CARTESIAN_POINT('Ctrl Pts',(-41.7024321922921,40.1713201842097,40.6187740530706));
#32290=CARTESIAN_POINT('Ctrl Pts',(-41.7150362498594,40.2585945794838,40.6291779329183));
#32291=CARTESIAN_POINT('Ctrl Pts',(-41.7276403074267,40.345868974758,40.639581812766));
#32292=CARTESIAN_POINT('Ctrl Pts',(-41.7386419556478,40.4335760538542,40.6483011158255));
#32293=CARTESIAN_POINT('Ctrl Pts',(-41.7480255699405,40.5215915345635,40.6553234512153));
#32294=CARTESIAN_POINT('Ctrl Pts',(-41.7574091842331,40.6096070152727,40.6623457866051));
#32295=CARTESIAN_POINT('Ctrl Pts',(-41.7651747620727,40.697930874039,40.6676711524323));
#32296=CARTESIAN_POINT('Ctrl Pts',(-41.7713112619682,40.78643795248,40.6712919645219));
#32297=CARTESIAN_POINT('Ctrl Pts',(-41.777453215633,40.8750236909366,40.6749159945816));
#32298=CARTESIAN_POINT('Ctrl Pts',(-41.7819631927455,40.9637929511522,40.6768324387531));
#32299=CARTESIAN_POINT('Ctrl Pts',(-41.7848347491195,41.0526197175773,40.6770385337885));
#32300=CARTESIAN_POINT('Ctrl Pts',(-40.4421239266209,37.3321517734995,39.4725925144174));
#32301=CARTESIAN_POINT('Ctrl Pts',(-40.4910131080268,37.3899122066288,39.521788505816));
#32302=CARTESIAN_POINT('Ctrl Pts',(-40.5388489780531,37.4495498910191,39.5698271574031));
#32303=CARTESIAN_POINT('Ctrl Pts',(-40.5855614742959,37.510977482102,39.6166381108269));
#32304=CARTESIAN_POINT('Ctrl Pts',(-40.6322739705388,37.5724050731848,39.6634490642507));
#32305=CARTESIAN_POINT('Ctrl Pts',(-40.6778630796419,37.6356225533988,39.709032306127));
#32306=CARTESIAN_POINT('Ctrl Pts',(-40.7222620279456,37.70053733785,39.753321072269));
#32307=CARTESIAN_POINT('Ctrl Pts',(-40.7666609762493,37.7654521223013,39.797609838411));
#32308=CARTESIAN_POINT('Ctrl Pts',(-40.809869751058,37.8320641924323,39.8406041161547));
#32309=CARTESIAN_POINT('Ctrl Pts',(-40.8518250628848,37.9002759939679,39.8822409308761));
#32310=CARTESIAN_POINT('Ctrl Pts',(-40.8937803747117,37.9684877955036,39.9238777455974));
#32311=CARTESIAN_POINT('Ctrl Pts',(-40.9344822115587,38.0382993089447,39.9641570853898));
#32312=CARTESIAN_POINT('Ctrl Pts',(-40.9738709533507,38.1096082961141,40.0030199495069));
#32313=CARTESIAN_POINT('Ctrl Pts',(-41.0132596951426,38.1809172832835,40.041882813624));
#32314=CARTESIAN_POINT('Ctrl Pts',(-41.0513353306142,38.2537237237974,40.0793291909511));
#32315=CARTESIAN_POINT('Ctrl Pts',(-41.0880420836084,38.3279209947579,40.1153042273124));
#32316=CARTESIAN_POINT('Ctrl Pts',(-41.1247488366024,38.4021182657185,40.1512792636738));
#32317=CARTESIAN_POINT('Ctrl Pts',(-41.1600866966196,38.4777063459167,40.1857829487792));
#32318=CARTESIAN_POINT('Ctrl Pts',(-41.1940038946856,38.5545745397419,40.2187647355886));
#32319=CARTESIAN_POINT('Ctrl Pts',(-41.2279210927516,38.6314427335672,40.2517465223981));
#32320=CARTESIAN_POINT('Ctrl Pts',(-41.2604176191636,38.7095910190472,40.2832064014761));
#32321=CARTESIAN_POINT('Ctrl Pts',(-41.2914458636761,38.7889049517819,40.3130982808877));
#32322=CARTESIAN_POINT('Ctrl Pts',(-41.3224741081885,38.8682188845166,40.3429901602992));
#32323=CARTESIAN_POINT('Ctrl Pts',(-41.3520340619235,38.9486984418346,40.371314031491));
#32324=CARTESIAN_POINT('Ctrl Pts',(-41.3800824127475,39.0302257654376,40.3980283925727));
#32325=CARTESIAN_POINT('Ctrl Pts',(-41.4081307635715,39.1117530890405,40.4247427536544));
#32326=CARTESIAN_POINT('Ctrl Pts',(-41.4346675034574,39.1943281556243,40.4498475969801));
#32327=CARTESIAN_POINT('Ctrl Pts',(-41.4596537451974,39.2778300378728,40.4733061322202));
#32328=CARTESIAN_POINT('Ctrl Pts',(-41.4846399869374,39.3613319201213,40.4967646674603));
#32329=CARTESIAN_POINT('Ctrl Pts',(-41.5080757233786,39.4457605941657,40.5185768878985));
#32330=CARTESIAN_POINT('Ctrl Pts',(-41.5299266061116,39.5309924175345,40.5387108225031));
#32331=CARTESIAN_POINT('Ctrl Pts',(-41.5517774888446,39.6162242409034,40.5588447571076));
#32332=CARTESIAN_POINT('Ctrl Pts',(-41.5720435116116,39.7022591892331,40.5773004001115));
#32333=CARTESIAN_POINT('Ctrl Pts',(-41.5906949654003,39.7889712667059,40.5940506934234));
#32334=CARTESIAN_POINT('Ctrl Pts',(-41.6093464191891,39.8756833441786,40.6108009867352));
#32335=CARTESIAN_POINT('Ctrl Pts',(-41.6263832986553,39.9630725260074,40.6258459255541));
#32336=CARTESIAN_POINT('Ctrl Pts',(-41.6417806212144,40.051010831727,40.6391634440034));
#32337=CARTESIAN_POINT('Ctrl Pts',(-41.6571779437735,40.1389491374466,40.6524809624527));
#32338=CARTESIAN_POINT('Ctrl Pts',(-41.6709357050106,40.2274365419188,40.6640710567117));
#32339=CARTESIAN_POINT('Ctrl Pts',(-41.6830337219766,40.3163434545426,40.6739167177927));
#32340=CARTESIAN_POINT('Ctrl Pts',(-41.6951317389425,40.4052503671663,40.6837623788737));
#32341=CARTESIAN_POINT('Ctrl Pts',(-41.7055700081645,40.4945767625257,40.6918636039474));
#32342=CARTESIAN_POINT('Ctrl Pts',(-41.7143332054998,40.5841918191118,40.6982084907992));
#32343=CARTESIAN_POINT('Ctrl Pts',(-41.7230964028351,40.6738068756978,40.7045533776511));
#32344=CARTESIAN_POINT('Ctrl Pts',(-41.730184525763,40.7637105678913,40.7091419244515));
#32345=CARTESIAN_POINT('Ctrl Pts',(-41.7355871539075,40.8537712261132,40.711967370708));
#32346=CARTESIAN_POINT('Ctrl Pts',(-41.7409945835981,40.9439119250834,40.7147953280591));
#32347=CARTESIAN_POINT('Ctrl Pts',(-41.7447135196681,41.0342098434169,40.7158570487623));
#32348=CARTESIAN_POINT('Ctrl Pts',(-41.746738461486,41.1245324961841,40.7151509296908));
#32349=CARTESIAN_POINT('Ctrl Pts',(-40.4026917455303,37.3333248863599,39.5103831374403));
#32350=CARTESIAN_POINT('Ctrl Pts',(-40.4523532259874,37.392012397429,39.5603800219979));
#32351=CARTESIAN_POINT('Ctrl Pts',(-40.500927035616,37.4526383953682,39.6091818138752));
#32352=CARTESIAN_POINT('Ctrl Pts',(-40.548339675232,37.5151111442932,39.6567146689183));
#32353=CARTESIAN_POINT('Ctrl Pts',(-40.595752314848,37.5775838932182,39.7042475239613));
#32354=CARTESIAN_POINT('Ctrl Pts',(-40.6420037699661,37.6419033740425,39.750511427648));
#32355=CARTESIAN_POINT('Ctrl Pts',(-40.6870240554598,37.7079722621093,39.7954363760154));
#32356=CARTESIAN_POINT('Ctrl Pts',(-40.7320443409536,37.7740411501762,39.8403613243828));
#32357=CARTESIAN_POINT('Ctrl Pts',(-40.7758334430686,37.8418594253004,39.8839473037057));
#32358=CARTESIAN_POINT('Ctrl Pts',(-40.8183251025737,37.9113244686443,39.9261283621071));
#32359=CARTESIAN_POINT('Ctrl Pts',(-40.8608167620789,37.9807895119883,39.9683094205084));
#32360=CARTESIAN_POINT('Ctrl Pts',(-40.9020109659924,38.0519013023294,40.0090855451013));
#32361=CARTESIAN_POINT('Ctrl Pts',(-40.9418453815386,38.1245522372661,40.0483950357245));
#32362=CARTESIAN_POINT('Ctrl Pts',(-40.9816797970848,38.1972031722028,40.0877045263477));
#32363=CARTESIAN_POINT('Ctrl Pts',(-41.0201544120938,38.2713932295392,40.1255473709915));
#32364=CARTESIAN_POINT('Ctrl Pts',(-41.0572110089203,38.3470101490115,40.1618663079706));
#32365=CARTESIAN_POINT('Ctrl Pts',(-41.0942676057469,38.4226270684837,40.1981852449497));
#32366=CARTESIAN_POINT('Ctrl Pts',(-41.1299061730698,38.4996708269898,40.2329802631682));
#32367=CARTESIAN_POINT('Ctrl Pts',(-41.1640727845932,38.5780248462043,40.2661987127418));
#32368=CARTESIAN_POINT('Ctrl Pts',(-41.1982393961167,38.6563788654189,40.2994171623154));
#32369=CARTESIAN_POINT('Ctrl Pts',(-41.2309340414024,38.7360431214034,40.3310590330955));
#32370=CARTESIAN_POINT('Ctrl Pts',(-41.2621072487336,38.8168970706418,40.361076446365));
#32371=CARTESIAN_POINT('Ctrl Pts',(-41.2932804560647,38.8977510198801,40.3910938596345));
#32372=CARTESIAN_POINT('Ctrl Pts',(-41.3229322159175,38.9797946376701,40.4194868062228));
#32373=CARTESIAN_POINT('Ctrl Pts',(-41.3510176608998,39.0629037801777,40.4462123235039));
#32374=CARTESIAN_POINT('Ctrl Pts',(-41.3791031058822,39.1460129226852,40.472937840785));
#32375=CARTESIAN_POINT('Ctrl Pts',(-41.4056222274137,39.2301875645192,40.497995920594));
#32376=CARTESIAN_POINT('Ctrl Pts',(-41.4305348982363,39.3153003372986,40.5213486464397));
#32377=CARTESIAN_POINT('Ctrl Pts',(-41.4554475690588,39.400413110078,40.5447013722854));
#32378=CARTESIAN_POINT('Ctrl Pts',(-41.4787537815612,39.4864639877996,40.5663487370333));
#32379=CARTESIAN_POINT('Ctrl Pts',(-41.5004182700804,39.5733227630668,40.5862579850963));
#32380=CARTESIAN_POINT('Ctrl Pts',(-41.5220827585996,39.6601815383338,40.6061672331594));
#32381=CARTESIAN_POINT('Ctrl Pts',(-41.5421055165168,39.7478481846099,40.624338358455));
#32382=CARTESIAN_POINT('Ctrl Pts',(-41.5604562465096,39.8361900496069,40.6407438654482));
#32383=CARTESIAN_POINT('Ctrl Pts',(-41.5788069765024,39.924531914604,40.6571493724415));
#32384=CARTESIAN_POINT('Ctrl Pts',(-41.5954856729644,40.0135489713325,40.6717892561202));
#32385=CARTESIAN_POINT('Ctrl Pts',(-41.6104670986208,40.1031065241387,40.6846413642276));
#32386=CARTESIAN_POINT('Ctrl Pts',(-41.6254485242772,40.1926640769449,40.697493472335));
#32387=CARTESIAN_POINT('Ctrl Pts',(-41.638732674551,40.2827620984677,40.7085578009445));
#32388=CARTESIAN_POINT('Ctrl Pts',(-41.6502994486055,40.3732642573977,40.7178176081302));
#32389=CARTESIAN_POINT('Ctrl Pts',(-41.6618662226601,40.4637664163277,40.7270774153159));
#32390=CARTESIAN_POINT('Ctrl Pts',(-41.6717156169618,40.5546726850152,40.7345326982488));
#32391=CARTESIAN_POINT('Ctrl Pts',(-41.6798327279554,40.6458455091562,40.7401721760098));
#32392=CARTESIAN_POINT('Ctrl Pts',(-41.687949838949,40.7370183332971,40.7458116537709));
#32393=CARTESIAN_POINT('Ctrl Pts',(-41.6943346641547,40.8284576850369,40.7496353246372));
#32394=CARTESIAN_POINT('Ctrl Pts',(-41.6989775424105,40.92002520344,40.7516374028428));
#32395=CARTESIAN_POINT('Ctrl Pts',(-41.7036245469903,41.0116741018023,40.7536412603807));
#32396=CARTESIAN_POINT('Ctrl Pts',(-41.7065265055382,41.1034513667184,40.7538202853523));
#32397=CARTESIAN_POINT('Ctrl Pts',(-41.7076790168147,41.1952178791612,40.7521742039289));
#32398=CARTESIAN_POINT('Ctrl Pts',(-40.3238273833491,37.3356711120808,39.5859643834861));
#32399=CARTESIAN_POINT('Ctrl Pts',(-40.3750334619085,37.3962127790296,39.6375630543615));
#32400=CARTESIAN_POINT('Ctrl Pts',(-40.4250831507418,37.4588154040666,39.6878911268195));
#32401=CARTESIAN_POINT('Ctrl Pts',(-40.4738960771041,37.5233784686756,39.736867785101));
#32402=CARTESIAN_POINT('Ctrl Pts',(-40.5227090034662,37.5879415332848,39.7858444433824));
#32403=CARTESIAN_POINT('Ctrl Pts',(-40.5702851506146,37.65446501533,39.83346967069));
#32404=CARTESIAN_POINT('Ctrl Pts',(-40.6165481104883,37.722842110628,39.8796669835082));
#32405=CARTESIAN_POINT('Ctrl Pts',(-40.6628110703621,37.7912192059259,39.9258642963265));
#32406=CARTESIAN_POINT('Ctrl Pts',(-40.7077608270898,37.8614498910366,39.9706336788078));
#32407=CARTESIAN_POINT('Ctrl Pts',(-40.7513251819515,37.9334214179972,40.0139032245691));
#32408=CARTESIAN_POINT('Ctrl Pts',(-40.7948895368132,38.0053929449577,40.0571727703304));
#32409=CARTESIAN_POINT('Ctrl Pts',(-40.8370684748596,38.0791052890989,40.0989424645244));
#32410=CARTESIAN_POINT('Ctrl Pts',(-40.8777942379143,38.1544401195702,40.1391452081597));
#32411=CARTESIAN_POINT('Ctrl Pts',(-40.9185200009691,38.2297749500413,40.1793479517951));
#32412=CARTESIAN_POINT('Ctrl Pts',(-40.9577925750527,38.3067322410228,40.2179837310723));
#32413=CARTESIAN_POINT('Ctrl Pts',(-40.9955488595443,38.3851884575184,40.2549904692869));
#32414=CARTESIAN_POINT('Ctrl Pts',(-41.0333051440358,38.4636446740141,40.2919972075016));
#32415=CARTESIAN_POINT('Ctrl Pts',(-41.06954512597,38.5435997891364,40.3273748919461));
#32416=CARTESIAN_POINT('Ctrl Pts',(-41.1042105644085,38.6249254591294,40.361066667048));
#32417=CARTESIAN_POINT('Ctrl Pts',(-41.1388760028468,38.7062511291223,40.39475844215));
#32418=CARTESIAN_POINT('Ctrl Pts',(-41.1719668858801,38.7889473261161,40.4267642963341));
#32419=CARTESIAN_POINT('Ctrl Pts',(-41.2034300188486,38.8728813083616,40.4570327773197));
#32420=CARTESIAN_POINT('Ctrl Pts',(-41.2348931518171,38.9568152906071,40.4873012583052));
#32421=CARTESIAN_POINT('Ctrl Pts',(-41.2647285239056,39.041987029341,40.5158323556863));
#32422=CARTESIAN_POINT('Ctrl Pts',(-41.2928881572047,39.1282598096577,40.5425801853663));
#32423=CARTESIAN_POINT('Ctrl Pts',(-41.3210477905038,39.2145325899743,40.5693280150463));
#32424=CARTESIAN_POINT('Ctrl Pts',(-41.3475316753265,39.3019063823089,40.5942925678218));
#32425=CARTESIAN_POINT('Ctrl Pts',(-41.3722972043141,39.3902409361501,40.6174336748788));
#32426=CARTESIAN_POINT('Ctrl Pts',(-41.3970627333016,39.4785754899914,40.6405747819357));
#32427=CARTESIAN_POINT('Ctrl Pts',(-41.4201098979263,39.5678707750675,40.6618924353029));
#32428=CARTESIAN_POINT('Ctrl Pts',(-41.4414015980179,39.6579834541311,40.6813523102829));
#32429=CARTESIAN_POINT('Ctrl Pts',(-41.4626932981095,39.7480961331947,40.7008121852628));
#32430=CARTESIAN_POINT('Ctrl Pts',(-41.482229526327,39.8390261753633,40.7184142751419));
#32431=CARTESIAN_POINT('Ctrl Pts',(-41.499978808728,39.930627615409,40.734130209498));
#32432=CARTESIAN_POINT('Ctrl Pts',(-41.517728091129,40.0222290554547,40.7498461438541));
#32433=CARTESIAN_POINT('Ctrl Pts',(-41.5336904215826,40.1145018619828,40.7636759172525));
#32434=CARTESIAN_POINT('Ctrl Pts',(-41.5478400534335,40.2072979089622,40.775597204676));
#32435=CARTESIAN_POINT('Ctrl Pts',(-41.5619896852844,40.3000939559416,40.7875184920995));
#32436=CARTESIAN_POINT('Ctrl Pts',(-41.5743266136316,40.3934132115655,40.7975312894101));
#32437=CARTESIAN_POINT('Ctrl Pts',(-41.5848309018635,40.4871058631079,40.8056193888052));
#32438=CARTESIAN_POINT('Ctrl Pts',(-41.5953351900953,40.5807985146504,40.8137074882003));
#32439=CARTESIAN_POINT('Ctrl Pts',(-41.6040068345563,40.6748645299942,40.8198708868516));
#32440=CARTESIAN_POINT('Ctrl Pts',(-41.6108317728666,40.769152889245,40.824099546431));
#32441=CARTESIAN_POINT('Ctrl Pts',(-41.6176567111769,40.8634412484956,40.8283282060105));
#32442=CARTESIAN_POINT('Ctrl Pts',(-41.6226349409381,40.9579519193281,40.8306221250085));
#32443=CARTESIAN_POINT('Ctrl Pts',(-41.6257583194165,41.0525331580936,40.8309774671124));
#32444=CARTESIAN_POINT('Ctrl Pts',(-41.6288844737746,41.1471984552401,40.831333125024));
#32445=CARTESIAN_POINT('Ctrl Pts',(-41.6301524772784,41.2419344133214,40.8297467585323));
#32446=CARTESIAN_POINT('Ctrl Pts',(-41.6295601274722,41.3365886451155,40.8262207524052));
#32447=CARTESIAN_POINT('Ctrl Pts',(-40.2449312129505,37.3379802045158,39.6615143463265));
#32448=CARTESIAN_POINT('Ctrl Pts',(-40.2976328145503,37.4003117501095,39.7146552060781));
#32449=CARTESIAN_POINT('Ctrl Pts',(-40.3491084470698,37.4648282580176,39.7664490162522));
#32450=CARTESIAN_POINT('Ctrl Pts',(-40.3992704605161,37.5314198852677,39.8168075871395));
#32451=CARTESIAN_POINT('Ctrl Pts',(-40.4494324739624,37.5980115125179,39.8671661580268));
#32452=CARTESIAN_POINT('Ctrl Pts',(-40.4982808489931,37.6666782334438,39.9160894702099));
#32453=CARTESIAN_POINT('Ctrl Pts',(-40.5457324008023,37.7373031500135,39.9634942126056));
#32454=CARTESIAN_POINT('Ctrl Pts',(-40.5931839526115,37.8079280665833,40.0108989550013));
#32455=CARTESIAN_POINT('Ctrl Pts',(-40.6392386628975,37.8805111515807,40.0567851093263));
#32456=CARTESIAN_POINT('Ctrl Pts',(-40.6838180944329,37.9549288486176,40.1010745259389));
#32457=CARTESIAN_POINT('Ctrl Pts',(-40.7283975259683,38.0293465456543,40.1453639425515));
#32458=CARTESIAN_POINT('Ctrl Pts',(-40.7715016615542,38.1055988260566,40.1880566043646));
#32459=CARTESIAN_POINT('Ctrl Pts',(-40.8130570778548,38.1835558943449,40.2290797885122));
#32460=CARTESIAN_POINT('Ctrl Pts',(-40.8546124941553,38.2615129626333,40.2701029726598));
#32461=CARTESIAN_POINT('Ctrl Pts',(-40.8946191751323,38.341174788773,40.3094566633089));
#32462=CARTESIAN_POINT('Ctrl Pts',(-40.9330089606741,38.4224057786039,40.3470738113249));
#32463=CARTESIAN_POINT('Ctrl Pts',(-40.9713987462159,38.5036367684348,40.3846909593409));
#32464=CARTESIAN_POINT('Ctrl Pts',(-41.0081716214994,38.5864368906626,40.4205715501982));
#32465=CARTESIAN_POINT('Ctrl Pts',(-41.0432649211462,38.6706652125133,40.4546544362353));
#32466=CARTESIAN_POINT('Ctrl Pts',(-41.078358220793,38.7548935343639,40.4887373222725));
#32467=CARTESIAN_POINT('Ctrl Pts',(-41.1117719312452,38.8405500233895,40.5210224903204));
#32468=CARTESIAN_POINT('Ctrl Pts',(-41.1434490947603,38.9274888863699,40.5514549019477));
#32469=CARTESIAN_POINT('Ctrl Pts',(-41.1751262582754,39.0144277493503,40.581887313575));
#32470=CARTESIAN_POINT('Ctrl Pts',(-41.2050668626066,39.1026489527938,40.6104669570138));
#32471=CARTESIAN_POINT('Ctrl Pts',(-41.2332198512222,39.1920023376887,40.6371450901319));
#32472=CARTESIAN_POINT('Ctrl Pts',(-41.2613728398378,39.2813557225836,40.6638232232499));
#32473=CARTESIAN_POINT('Ctrl Pts',(-41.2877382018437,39.3718412545073,40.6885998357202));
#32474=CARTESIAN_POINT('Ctrl Pts',(-41.3122709555114,39.4633049181251,40.7114326474576));
#32475=CARTESIAN_POINT('Ctrl Pts',(-41.3368037091791,39.5547685817429,40.7342654591949));
#32476=CARTESIAN_POINT('Ctrl Pts',(-41.359503845004,39.6472103418177,40.7551544613484));
#32477=CARTESIAN_POINT('Ctrl Pts',(-41.3803326090827,39.7404728492527,40.7740639797447));
#32478=CARTESIAN_POINT('Ctrl Pts',(-41.4011613731614,39.8337353566877,40.792973498141));
#32479=CARTESIAN_POINT('Ctrl Pts',(-41.4201187574111,39.9278185755504,40.8099035254352));
#32480=CARTESIAN_POINT('Ctrl Pts',(-41.4371723676855,40.0225623568698,40.8248251148608));
#32481=CARTESIAN_POINT('Ctrl Pts',(-41.4542259779599,40.1173061381893,40.8397467042862));
#32482=CARTESIAN_POINT('Ctrl Pts',(-41.4693758076255,40.212710445459,40.8526598500291));
#32483=CARTESIAN_POINT('Ctrl Pts',(-41.4825959326887,40.3086128732442,40.8635424314407));
#32484=CARTESIAN_POINT('Ctrl Pts',(-41.4958160577518,40.4045153010295,40.8744250128523));
#32485=CARTESIAN_POINT('Ctrl Pts',(-41.5071064730508,40.5009158123731,40.8832770256696));
#32486=CARTESIAN_POINT('Ctrl Pts',(-41.5164478132281,40.5976502964727,40.8900832509554));
#32487=CARTESIAN_POINT('Ctrl Pts',(-41.5257891534055,40.6943847805722,40.8968894762412));
#32488=CARTESIAN_POINT('Ctrl Pts',(-41.5331814147889,40.7914532001451,40.9016499112979));
#32489=CARTESIAN_POINT('Ctrl Pts',(-41.5386118569276,40.8886902959407,40.9043562911171));
#32490=CARTESIAN_POINT('Ctrl Pts',(-41.5440422990664,40.9859273917364,40.9070626709362));
#32491=CARTESIAN_POINT('Ctrl Pts',(-41.54751091979,41.0833331262726,40.9077149943948));
#32492=CARTESIAN_POINT('Ctrl Pts',(-41.5490116473865,41.1807416527115,40.9063119790764));
#32493=CARTESIAN_POINT('Ctrl Pts',(-41.5505137087437,41.2782367502626,40.9049077168384));
#32494=CARTESIAN_POINT('Ctrl Pts',(-41.550044376856,41.375734607059,40.9014444613216));
#32495=CARTESIAN_POINT('Ctrl Pts',(-41.5476042716421,41.4730689089368,40.8959279329355));
#32496=CARTESIAN_POINT('Ctrl Pts',(-40.166020457705,37.3402722704297,39.7370499650508));
#32497=CARTESIAN_POINT('Ctrl Pts',(-40.2201818127886,37.4043453509955,39.7916871518576));
#32498=CARTESIAN_POINT('Ctrl Pts',(-40.2730467145036,37.4707290102875,39.8448998436378));
#32499=CARTESIAN_POINT('Ctrl Pts',(-40.3245198289288,37.539303535333,39.8965920792831));
#32500=CARTESIAN_POINT('Ctrl Pts',(-40.375992943354,37.6078780603784,39.9482843149283));
#32501=CARTESIAN_POINT('Ctrl Pts',(-40.4260742481497,37.6786434214157,39.998456072004));
#32502=CARTESIAN_POINT('Ctrl Pts',(-40.4746734291945,37.7514720037299,40.0470168732713));
#32503=CARTESIAN_POINT('Ctrl Pts',(-40.5232726102392,37.8243005860441,40.0955776745386));
#32504=CARTESIAN_POINT('Ctrl Pts',(-40.5703896464407,37.8991923580274,40.1425274989219));
#32505=CARTESIAN_POINT('Ctrl Pts',(-40.615939569291,37.9760122636019,40.1877816794548));
#32506=CARTESIAN_POINT('Ctrl Pts',(-40.6614894921413,38.0528321691764,40.2330358599877));
#32507=CARTESIAN_POINT('Ctrl Pts',(-40.7054722818716,38.1315801750017,40.2765943770297));
#32508=CARTESIAN_POINT('Ctrl Pts',(-40.7478086221175,38.2121142708607,40.3183786793286));
#32509=CARTESIAN_POINT('Ctrl Pts',(-40.7901449623634,38.2926483667197,40.3601629816274));
#32510=CARTESIAN_POINT('Ctrl Pts',(-40.8308348347507,38.3749685176602,40.4001730510485));
#32511=CARTESIAN_POINT('Ctrl Pts',(-40.8698048611974,38.4589262716369,40.4383367354326));
#32512=CARTESIAN_POINT('Ctrl Pts',(-40.9087748876443,38.5428840256135,40.4765004198168));
#32513=CARTESIAN_POINT('Ctrl Pts',(-40.9460250512374,38.6284793461884,40.5128177026007));
#32514=CARTESIAN_POINT('Ctrl Pts',(-40.9814881768939,38.7155578750389,40.5472230910122));
#32515=CARTESIAN_POINT('Ctrl Pts',(-41.0169513025503,38.8026364038895,40.5816284794236));
#32516=CARTESIAN_POINT('Ctrl Pts',(-41.050627374879,38.8911981032232,40.6141219585304));
#32517=CARTESIAN_POINT('Ctrl Pts',(-41.0824556641344,38.9810832652986,40.6446449312166));
#32518=CARTESIAN_POINT('Ctrl Pts',(-41.1142839533898,39.070968427374,40.6751679039028));
#32519=CARTESIAN_POINT('Ctrl Pts',(-41.1442644457583,39.1621770131804,40.7037203569213));
#32520=CARTESIAN_POINT('Ctrl Pts',(-41.1723430759186,39.2545445417134,40.7302508002056));
#32521=CARTESIAN_POINT('Ctrl Pts',(-41.2004217060789,39.3469120702464,40.7567812434898));
#32522=CARTESIAN_POINT('Ctrl Pts',(-41.2265984618448,39.4404385014183,40.7812896655255));
#32523=CARTESIAN_POINT('Ctrl Pts',(-41.2508261373634,39.5349551743379,40.8037318690495));
#32524=CARTESIAN_POINT('Ctrl Pts',(-41.275053812882,39.6294718472575,40.8261740725734));
#32525=CARTESIAN_POINT('Ctrl Pts',(-41.2973323976383,39.7249787209044,40.8465500478457));
#32526=CARTESIAN_POINT('Ctrl Pts',(-41.3176217155464,39.8213035629566,40.8648230498508));
#32527=CARTESIAN_POINT('Ctrl Pts',(-41.3379110334544,39.9176284050089,40.883096051856));
#32528=CARTESIAN_POINT('Ctrl Pts',(-41.3562110757085,40.014771173661,40.8992660726636));
#32529=CARTESIAN_POINT('Ctrl Pts',(-41.3724888409272,40.1125566865002,40.9133039520663));
#32530=CARTESIAN_POINT('Ctrl Pts',(-41.3887666061459,40.2103421993392,40.927341831469));
#32531=CARTESIAN_POINT('Ctrl Pts',(-41.4030220872645,40.3087704139258,40.9392475633744));
#32532=CARTESIAN_POINT('Ctrl Pts',(-41.415229576661,40.407663829738,40.9489996775807));
#32533=CARTESIAN_POINT('Ctrl Pts',(-41.4274370660576,40.50655724555,40.958751791787));
#32534=CARTESIAN_POINT('Ctrl Pts',(-41.437596558434,40.6059158196674,40.9663502840617));
#32535=CARTESIAN_POINT('Ctrl Pts',(-41.4456897326694,40.7055603738042,40.9717814516636));
#32536=CARTESIAN_POINT('Ctrl Pts',(-41.4537829069049,40.8052049279409,40.9772126192656));
#32537=CARTESIAN_POINT('Ctrl Pts',(-41.459809759487,40.9051354188509,40.9804764598378));
#32538=CARTESIAN_POINT('Ctrl Pts',(-41.4637594218909,41.0051716368821,40.981567087533));
#32539=CARTESIAN_POINT('Ctrl Pts',(-41.467709084295,41.1052078549132,40.9826577152283));
#32540=CARTESIAN_POINT('Ctrl Pts',(-41.4695815548068,41.2053497566493,40.9815751295735));
#32541=CARTESIAN_POINT('Ctrl Pts',(-41.4693734567066,41.3054167511905,40.9783212828493));
#32542=CARTESIAN_POINT('Ctrl Pts',(-41.4691651736608,41.4055726795378,40.9750645442929));
#32543=CARTESIAN_POINT('Ctrl Pts',(-41.46687262227,41.5056535239781,40.9696326849821));
#32544=CARTESIAN_POINT('Ctrl Pts',(-41.4624999408153,41.6054784826541,40.9620355143906));
#32545=CARTESIAN_POINT('Ctrl Pts',(-40.0871097024595,37.3425643363436,39.8125855837751));
#32546=CARTESIAN_POINT('Ctrl Pts',(-40.1427308110269,37.4083789518815,39.868719097637));
#32547=CARTESIAN_POINT('Ctrl Pts',(-40.1969849819375,37.4766297625575,39.9233506710234));
#32548=CARTESIAN_POINT('Ctrl Pts',(-40.2497691973415,37.5471871853983,39.9763765714266));
#32549=CARTESIAN_POINT('Ctrl Pts',(-40.3025534127456,37.617744608239,40.0294024718299));
#32550=CARTESIAN_POINT('Ctrl Pts',(-40.3538676473064,37.6906086093875,40.0808226737981));
#32551=CARTESIAN_POINT('Ctrl Pts',(-40.4036144575867,37.7656408574462,40.130539533937));
#32552=CARTESIAN_POINT('Ctrl Pts',(-40.453361267867,37.8406731055049,40.1802563940759));
#32553=CARTESIAN_POINT('Ctrl Pts',(-40.501540629984,37.9178735644741,40.2282698885175));
#32554=CARTESIAN_POINT('Ctrl Pts',(-40.5480610441492,37.9970956785862,40.2744888329708));
#32555=CARTESIAN_POINT('Ctrl Pts',(-40.5945814583144,38.0763177926983,40.320707777424));
#32556=CARTESIAN_POINT('Ctrl Pts',(-40.6394429021891,38.1575615239468,40.365132149695));
#32557=CARTESIAN_POINT('Ctrl Pts',(-40.6825601663803,38.2406726473765,40.407677570145));
#32558=CARTESIAN_POINT('Ctrl Pts',(-40.7256774305715,38.3237837708061,40.450222990595));
#32559=CARTESIAN_POINT('Ctrl Pts',(-40.767050494369,38.4087622465473,40.4908894387881));
#32560=CARTESIAN_POINT('Ctrl Pts',(-40.8066007617208,38.4954467646698,40.5295996595404));
#32561=CARTESIAN_POINT('Ctrl Pts',(-40.8461510290726,38.5821312827923,40.5683098802926));
#32562=CARTESIAN_POINT('Ctrl Pts',(-40.8838784809754,38.6705218017141,40.6050638550033));
#32563=CARTESIAN_POINT('Ctrl Pts',(-40.9197114326415,38.7604505375645,40.639791745789));
#32564=CARTESIAN_POINT('Ctrl Pts',(-40.9555443843077,38.850379273415,40.6745196365747));
#32565=CARTESIAN_POINT('Ctrl Pts',(-40.9894828185128,38.941846183057,40.7072214267404));
#32566=CARTESIAN_POINT('Ctrl Pts',(-41.0214622335085,39.0346776442273,40.7378349604855));
#32567=CARTESIAN_POINT('Ctrl Pts',(-41.0534416485042,39.1275091053977,40.7684484942305));
#32568=CARTESIAN_POINT('Ctrl Pts',(-41.08346202891,39.2217050735669,40.7969737568287));
#32569=CARTESIAN_POINT('Ctrl Pts',(-41.111466300615,39.3170867457382,40.8233565102792));
#32570=CARTESIAN_POINT('Ctrl Pts',(-41.1394705723201,39.4124684179094,40.8497392637297));
#32571=CARTESIAN_POINT('Ctrl Pts',(-41.1654587218459,39.5090357483292,40.8739794953308));
#32572=CARTESIAN_POINT('Ctrl Pts',(-41.1893813192154,39.6066054305506,40.8960310906414));
#32573=CARTESIAN_POINT('Ctrl Pts',(-41.2133039165849,39.7041751127721,40.918082685952));
#32574=CARTESIAN_POINT('Ctrl Pts',(-41.2351609502726,39.8027470999911,40.9379456343429));
#32575=CARTESIAN_POINT('Ctrl Pts',(-41.2549108220101,39.9021342766605,40.955582119957));
#32576=CARTESIAN_POINT('Ctrl Pts',(-41.2746606937475,40.00152145333,40.973218605571));
#32577=CARTESIAN_POINT('Ctrl Pts',(-41.292303394006,40.1017237717717,40.9886286198919));
#32578=CARTESIAN_POINT('Ctrl Pts',(-41.3078053141689,40.2025510161305,41.0017827892718));
#32579=CARTESIAN_POINT('Ctrl Pts',(-41.3233072343318,40.3033782604891,41.0149369586518));
#32580=CARTESIAN_POINT('Ctrl Pts',(-41.3366683669035,40.4048303823926,41.0258352767197));
#32581=CARTESIAN_POINT('Ctrl Pts',(-41.3478632206334,40.5067147862316,41.0344569237207));
#32582=CARTESIAN_POINT('Ctrl Pts',(-41.3590580743634,40.6085991900705,41.0430785707216));
#32583=CARTESIAN_POINT('Ctrl Pts',(-41.3680866438171,40.7109158269618,41.0494235424537));
#32584=CARTESIAN_POINT('Ctrl Pts',(-41.3749316521107,40.8134704511357,41.0534796523719));
#32585=CARTESIAN_POINT('Ctrl Pts',(-41.3817766604043,40.9160250753096,41.05753576229));
#32586=CARTESIAN_POINT('Ctrl Pts',(-41.386438104185,41.0188176375568,41.0593030083776));
#32587=CARTESIAN_POINT('Ctrl Pts',(-41.3889069868543,41.1216529778233,41.058777883949));
#32588=CARTESIAN_POINT('Ctrl Pts',(-41.3913758695236,41.2244883180898,41.0582527595205));
#32589=CARTESIAN_POINT('Ctrl Pts',(-41.3916521898236,41.3273663870258,41.0554352647522));
#32590=CARTESIAN_POINT('Ctrl Pts',(-41.3897352660267,41.4300918496695,41.0503305866223));
#32591=CARTESIAN_POINT('Ctrl Pts',(-41.3878166385779,41.5329086088132,41.0452213717473));
#32592=CARTESIAN_POINT('Ctrl Pts',(-41.383700867684,41.6355724408973,41.0378209086425));
#32593=CARTESIAN_POINT('Ctrl Pts',(-41.3773956099884,41.7378880563715,41.0281430958457));
#32594=CARTESIAN_POINT('Ctrl Pts',(-40.0081842027545,37.3448391894026,39.8881067014052));
#32595=CARTESIAN_POINT('Ctrl Pts',(-40.065229152976,37.41234682335,39.9456905295488));
#32596=CARTESIAN_POINT('Ctrl Pts',(-40.1208357762505,37.4824178811549,40.0016939774043));
#32597=CARTESIAN_POINT('Ctrl Pts',(-40.1748929640454,37.5549123641953,40.0560051435073));
#32598=CARTESIAN_POINT('Ctrl Pts',(-40.2289501518402,37.6274068472357,40.1103163096102));
#32599=CARTESIAN_POINT('Ctrl Pts',(-40.2814578754243,37.7023247169942,40.1629351650944));
#32600=CARTESIAN_POINT('Ctrl Pts',(-40.3323112093966,37.7795163024568,40.2137565617103));
#32601=CARTESIAN_POINT('Ctrl Pts',(-40.3831645433688,37.8567078879194,40.2645779583263));
#32602=CARTESIAN_POINT('Ctrl Pts',(-40.4323634606956,37.9361731480789,40.3136018690566));
#32603=CARTESIAN_POINT('Ctrl Pts',(-40.4798096374514,38.0177533361164,40.3607303181027));
#32604=CARTESIAN_POINT('Ctrl Pts',(-40.5272558142073,38.0993335241538,40.4078587671488));
#32605=CARTESIAN_POINT('Ctrl Pts',(-40.5729492251636,38.1830285967346,40.4530917294489));
#32606=CARTESIAN_POINT('Ctrl Pts',(-40.6167985399401,38.2686713639595,40.4963387923452));
#32607=CARTESIAN_POINT('Ctrl Pts',(-40.6606478547166,38.3543141311843,40.5395858552415));
#32608=CARTESIAN_POINT('Ctrl Pts',(-40.7026530499896,38.4419045475642,40.580846995729));
#32609=CARTESIAN_POINT('Ctrl Pts',(-40.7427301531617,38.5312676464628,40.620039724875));
#32610=CARTESIAN_POINT('Ctrl Pts',(-40.7828072563337,38.6206307453612,40.659232454021));
#32611=CARTESIAN_POINT('Ctrl Pts',(-40.8209562460789,38.7117664793156,40.6963567509687));
#32612=CARTESIAN_POINT('Ctrl Pts',(-40.8571008425368,38.8044928022744,40.7313383795681));
#32613=CARTESIAN_POINT('Ctrl Pts',(-40.8932454389946,38.8972191252332,40.7663200081675));
#32614=CARTESIAN_POINT('Ctrl Pts',(-40.9273856229222,38.991535987948,40.7991589497917));
#32615=CARTESIAN_POINT('Ctrl Pts',(-40.9594531115379,39.0872549904745,40.8297895172827));
#32616=CARTESIAN_POINT('Ctrl Pts',(-40.9915206001535,39.182973993001,40.8604200847737));
#32617=CARTESIAN_POINT('Ctrl Pts',(-41.0215153763742,39.2800950845001,40.8888422618082));
#32618=CARTESIAN_POINT('Ctrl Pts',(-41.0493774270134,39.3784242619804,40.9149991724108));
#32619=CARTESIAN_POINT('Ctrl Pts',(-41.0772394776526,39.4767534394608,40.9411560830135));
#32620=CARTESIAN_POINT('Ctrl Pts',(-41.102968787854,39.5762906506965,40.9650477132315));
#32621=CARTESIAN_POINT('Ctrl Pts',(-41.126513853637,39.676837062824,40.9866262253897));
#32622=CARTESIAN_POINT('Ctrl Pts',(-41.15005891942,39.7773834749515,41.0082047375478));
#32623=CARTESIAN_POINT('Ctrl Pts',(-41.1714197282146,39.8789390345654,41.0274701201193));
#32624=CARTESIAN_POINT('Ctrl Pts',(-41.1905534909882,39.9813008713815,41.0443837648881));
#32625=CARTESIAN_POINT('Ctrl Pts',(-41.2096872537618,40.0836627081975,41.061297409657));
#32626=CARTESIAN_POINT('Ctrl Pts',(-41.2265939602815,40.1868307678413,41.0758593075667));
#32627=CARTESIAN_POINT('Ctrl Pts',(-41.2412397075264,40.290598951167,41.0880402342802));
#32628=CARTESIAN_POINT('Ctrl Pts',(-41.2558854547714,40.3943671344927,41.1002211609936));
#32629=CARTESIAN_POINT('Ctrl Pts',(-41.268270234886,40.4987353863741,41.1100211099617));
#32630=CARTESIAN_POINT('Ctrl Pts',(-41.2783691665588,40.6034952002683,41.1174203578003));
#32631=CARTESIAN_POINT('Ctrl Pts',(-41.2884680982315,40.7082550141624,41.124819605639));
#32632=CARTESIAN_POINT('Ctrl Pts',(-41.2962811760157,40.8134063344103,41.1298181483325));
#32633=CARTESIAN_POINT('Ctrl Pts',(-41.3017926401003,40.9187390781749,41.1324058427085));
#32634=CARTESIAN_POINT('Ctrl Pts',(-41.3073041041849,41.0240718219395,41.1349935370845));
#32635=CARTESIAN_POINT('Ctrl Pts',(-41.3105139515539,41.12958593325,41.1351703816769));
#32636=CARTESIAN_POINT('Ctrl Pts',(-41.3114156073819,41.235070590414,41.1329358546501));
#32637=CARTESIAN_POINT('Ctrl Pts',(-41.31231726321,41.3405552475781,41.1307013276233));
#32638=CARTESIAN_POINT('Ctrl Pts',(-41.3109107269242,41.4460103945356,41.1260554300668));
#32639=CARTESIAN_POINT('Ctrl Pts',(-41.3071986356094,41.5512253111845,41.119007264307));
#32640=CARTESIAN_POINT('Ctrl Pts',(-41.3034832452007,41.6565337368175,41.1119528345416));
#32641=CARTESIAN_POINT('Ctrl Pts',(-41.2974582017289,41.7616014489183,41.1024918683256));
#32642=CARTESIAN_POINT('Ctrl Pts',(-41.2891353760335,41.8662181092778,41.090643106539));
#32643=CARTESIAN_POINT('Ctrl Pts',(-39.929257160475,37.3471122416422,39.9636263019219));
#32644=CARTESIAN_POINT('Ctrl Pts',(-39.9876994389499,37.4162754036955,40.0226237631534));
#32645=CARTESIAN_POINT('Ctrl Pts',(-40.0446310452863,37.4881309212478,40.0799613539993));
#32646=CARTESIAN_POINT('Ctrl Pts',(-40.0999323645469,37.5625278237963,40.135518606537));
#32647=CARTESIAN_POINT('Ctrl Pts',(-40.1552336838076,37.6369247263448,40.1910758590747));
#32648=CARTESIAN_POINT('Ctrl Pts',(-40.2089046834089,37.7138629700548,40.24485274057));
#32649=CARTESIAN_POINT('Ctrl Pts',(-40.260832599042,37.7931809054704,40.2967362642528));
#32650=CARTESIAN_POINT('Ctrl Pts',(-40.3127605146749,37.8724988408859,40.3486197879357));
#32651=CARTESIAN_POINT('Ctrl Pts',(-40.3629453157436,37.9541964212729,40.3986099232363));
#32652=CARTESIAN_POINT('Ctrl Pts',(-40.4112815625419,38.0381019976722,40.4466016394471));
#32653=CARTESIAN_POINT('Ctrl Pts',(-40.4596178093403,38.1220075740716,40.4945933556579));
#32654=CARTESIAN_POINT('Ctrl Pts',(-40.5061054733888,38.2081210970459,40.5405866245016));
#32655=CARTESIAN_POINT('Ctrl Pts',(-40.550646882772,38.2962616396148,40.5844848128026));
#32656=CARTESIAN_POINT('Ctrl Pts',(-40.5951882921553,38.3844021821838,40.6283830011036));
#32657=CARTESIAN_POINT('Ctrl Pts',(-40.6377834206293,38.4745696924153,40.6701860829973));
#32658=CARTESIAN_POINT('Ctrl Pts',(-40.6783427746084,38.5665747257838,40.7098062290088));
#32659=CARTESIAN_POINT('Ctrl Pts',(-40.7189021285875,38.6585797591524,40.7494263750202));
#32660=CARTESIAN_POINT('Ctrl Pts',(-40.7574256841738,38.7524222614492,40.7868635618058));
#32661=CARTESIAN_POINT('Ctrl Pts',(-40.7938325022725,38.8479050668861,40.8220391327627));
#32662=CARTESIAN_POINT('Ctrl Pts',(-40.8302393203712,38.9433878723231,40.8572147037195));
#32663=CARTESIAN_POINT('Ctrl Pts',(-40.8645293795313,39.0405109246417,40.8901286381222));
#32664=CARTESIAN_POINT('Ctrl Pts',(-40.8966306353554,39.1390701655243,40.9207117828508));
#32665=CARTESIAN_POINT('Ctrl Pts',(-40.9287318911796,39.2376294064068,40.9512949275794));
#32666=CARTESIAN_POINT('Ctrl Pts',(-40.958644324754,39.3376247777812,40.9795472646133));
#32667=CARTESIAN_POINT('Ctrl Pts',(-40.9863050891974,39.4388461865069,41.0054094349843));
#32668=CARTESIAN_POINT('Ctrl Pts',(-41.0139658536407,39.5400675952327,41.0312716053553));
#32669=CARTESIAN_POINT('Ctrl Pts',(-41.0393749326551,39.6425149816702,41.0547435938255));
#32670=CARTESIAN_POINT('Ctrl Pts',(-41.062478941038,39.7459731009211,41.075776085072));
#32671=CARTESIAN_POINT('Ctrl Pts',(-41.0855829494209,39.849431220172,41.0968085763185));
#32672=CARTESIAN_POINT('Ctrl Pts',(-41.1063818735589,39.9539000112797,41.11540155795));
#32673=CARTESIAN_POINT('Ctrl Pts',(-41.124832014316,40.0591599823187,41.131515965579));
#32674=CARTESIAN_POINT('Ctrl Pts',(-41.1432821550731,40.1644199533577,41.147630373208));
#32675=CARTESIAN_POINT('Ctrl Pts',(-41.1593835015786,40.2704710423087,41.1612661973399));
#32676=CARTESIAN_POINT('Ctrl Pts',(-41.1731022244417,40.3770904327933,41.1723947887171));
#32677=CARTESIAN_POINT('Ctrl Pts',(-41.1868209473048,40.4837098232777,41.1835233800944));
#32678=CARTESIAN_POINT('Ctrl Pts',(-41.1981570384424,40.5908974524755,41.19214473216));
#32679=CARTESIAN_POINT('Ctrl Pts',(-41.207086680402,40.6984281161042,41.1982407312062));
#32680=CARTESIAN_POINT('Ctrl Pts',(-41.2160163223617,40.8059587797328,41.2043367302524));
#32681=CARTESIAN_POINT('Ctrl Pts',(-41.2225395098821,40.9138324144353,41.2079073726873));
#32682=CARTESIAN_POINT('Ctrl Pts',(-41.2266425375591,41.0218223746121,41.2089451564889));
#32683=CARTESIAN_POINT('Ctrl Pts',(-41.2307455652362,41.1298123347889,41.2099829402905));
#32684=CARTESIAN_POINT('Ctrl Pts',(-41.2324284306523,41.2379185568123,41.2084878648472));
#32685=CARTESIAN_POINT('Ctrl Pts',(-41.2316875980592,41.34591390641,41.2044630713555));
#32686=CARTESIAN_POINT('Ctrl Pts',(-41.2309467654661,41.4539092560078,41.2004382778638));
#32687=CARTESIAN_POINT('Ctrl Pts',(-41.2277822353002,41.561793669549,41.193883768695));
#32688=CARTESIAN_POINT('Ctrl Pts',(-41.22220065633,41.6693404787875,41.1848133150609));
#32689=CARTESIAN_POINT('Ctrl Pts',(-41.2166141167725,41.7769828694626,41.1757348001277));
#32690=CARTESIAN_POINT('Ctrl Pts',(-41.208606233529,41.8842869920002,41.1641358720405));
#32691=CARTESIAN_POINT('Ctrl Pts',(-41.1981938567826,41.9910269958237,41.1500409391072));
#32692=CARTESIAN_POINT('Ctrl Pts',(-39.8503301181955,37.3493852938817,40.0391459024386));
#32693=CARTESIAN_POINT('Ctrl Pts',(-39.9101697249238,37.4202039840409,40.0995569967581));
#32694=CARTESIAN_POINT('Ctrl Pts',(-39.9684263143221,37.4938439613405,40.1582287305944));
#32695=CARTESIAN_POINT('Ctrl Pts',(-40.0249717650485,37.5701432833972,40.2150320695668));
#32696=CARTESIAN_POINT('Ctrl Pts',(-40.081517215775,37.6464426054539,40.2718354085393));
#32697=CARTESIAN_POINT('Ctrl Pts',(-40.1363514913936,37.7254012231154,40.3267703160456));
#32698=CARTESIAN_POINT('Ctrl Pts',(-40.1893539886873,37.806845508484,40.3797159667953));
#32699=CARTESIAN_POINT('Ctrl Pts',(-40.242356485981,37.8882897938525,40.432661617545));
#32700=CARTESIAN_POINT('Ctrl Pts',(-40.2935271707916,37.9722196944668,40.483617977416));
#32701=CARTESIAN_POINT('Ctrl Pts',(-40.3427534876325,38.0584506592281,40.5324729607915));
#32702=CARTESIAN_POINT('Ctrl Pts',(-40.3919798044733,38.1446816239894,40.581327944167));
#32703=CARTESIAN_POINT('Ctrl Pts',(-40.439261721614,38.2332135973571,40.6280815195542));
#32704=CARTESIAN_POINT('Ctrl Pts',(-40.4844952256039,38.3238519152703,40.67263083326));
#32705=CARTESIAN_POINT('Ctrl Pts',(-40.5297287295939,38.4144902331834,40.7171801469658));
#32706=CARTESIAN_POINT('Ctrl Pts',(-40.572913791269,38.5072348372663,40.7595251702657));
#32707=CARTESIAN_POINT('Ctrl Pts',(-40.6139553960551,38.601881805105,40.7995727331425));
#32708=CARTESIAN_POINT('Ctrl Pts',(-40.6549970008413,38.6965287729436,40.8396202960194));
#32709=CARTESIAN_POINT('Ctrl Pts',(-40.6938951222687,38.7930780435828,40.8773703726429));
#32710=CARTESIAN_POINT('Ctrl Pts',(-40.7305641620082,38.8913173314979,40.9127398859572));
#32711=CARTESIAN_POINT('Ctrl Pts',(-40.7672332017477,38.989556619413,40.9481093992715));
#32712=CARTESIAN_POINT('Ctrl Pts',(-40.8016731361404,39.0894858613354,40.9810983264527));
#32713=CARTESIAN_POINT('Ctrl Pts',(-40.833808159173,39.190885340574,41.0116340484189));
#32714=CARTESIAN_POINT('Ctrl Pts',(-40.8659431822056,39.2922848198126,41.042169770385));
#32715=CARTESIAN_POINT('Ctrl Pts',(-40.8957732731339,39.3951544710623,41.0702522674185));
#32716=CARTESIAN_POINT('Ctrl Pts',(-40.9232327513814,39.4992681110334,41.0958196975579));
#32717=CARTESIAN_POINT('Ctrl Pts',(-40.9506922296289,39.6033817510046,41.1213871276972));
#32718=CARTESIAN_POINT('Ctrl Pts',(-40.9757810774562,39.7087393126439,41.1444394744195));
#32719=CARTESIAN_POINT('Ctrl Pts',(-40.998444028439,39.8151091390182,41.1649259447544));
#32720=CARTESIAN_POINT('Ctrl Pts',(-41.0211069794218,39.9214789653925,41.1854124150893));
#32721=CARTESIAN_POINT('Ctrl Pts',(-41.0413440189032,40.0288609879939,41.2033329957808));
#32722=CARTESIAN_POINT('Ctrl Pts',(-41.0591105376438,40.1370190932559,41.2186481662699));
#32723=CARTESIAN_POINT('Ctrl Pts',(-41.0768770563845,40.2451771985179,41.233963336759));
#32724=CARTESIAN_POINT('Ctrl Pts',(-41.0921730428756,40.3541113167763,41.246673087113));
#32725=CARTESIAN_POINT('Ctrl Pts',(-41.1049647413569,40.4635819144196,41.256749343154));
#32726=CARTESIAN_POINT('Ctrl Pts',(-41.1177564398381,40.5730525120629,41.266825599195));
#32727=CARTESIAN_POINT('Ctrl Pts',(-41.1280438419988,40.6830595185769,41.2742683543583));
#32728=CARTESIAN_POINT('Ctrl Pts',(-41.1358041942453,40.7933610319401,41.279061104612));
#32729=CARTESIAN_POINT('Ctrl Pts',(-41.1435645464919,40.9036625453032,41.2838538548657));
#32730=CARTESIAN_POINT('Ctrl Pts',(-41.1487978437484,41.0142584944603,41.2859965970421));
#32731=CARTESIAN_POINT('Ctrl Pts',(-41.1514924350179,41.1249056710494,41.2854844702693));
#32732=CARTESIAN_POINT('Ctrl Pts',(-41.1541870262875,41.2355528476383,41.2849723434964));
#32733=CARTESIAN_POINT('Ctrl Pts',(-41.1543429097509,41.3462511803745,41.2818053480175));
#32734=CARTESIAN_POINT('Ctrl Pts',(-41.1519595887366,41.4567572224059,41.2759902880609));
#32735=CARTESIAN_POINT('Ctrl Pts',(-41.1495762677222,41.5672632644374,41.2701752281043));
#32736=CARTESIAN_POINT('Ctrl Pts',(-41.1446537436761,41.6775769445624,41.2617121073232));
#32737=CARTESIAN_POINT('Ctrl Pts',(-41.1372026770507,41.7874556463905,41.2506193658148));
#32738=CARTESIAN_POINT('Ctrl Pts',(-41.1297449883444,41.8974320021077,41.2395167657139));
#32739=CARTESIAN_POINT('Ctrl Pts',(-41.1197542653291,42.0069725350821,41.2257798757554));
#32740=CARTESIAN_POINT('Ctrl Pts',(-41.1072523375316,42.1158358823698,41.2094387716753));
#32741=CARTESIAN_POINT('Ctrl Pts',(-39.7714014444761,37.3516564415591,40.1146638984432));
#32742=CARTESIAN_POINT('Ctrl Pts',(-39.8326117898446,37.4240930776539,40.1764518650056));
#32743=CARTESIAN_POINT('Ctrl Pts',(-39.8921658167799,37.4994816354714,40.2364199306906));
#32744=CARTESIAN_POINT('Ctrl Pts',(-39.9499264817845,37.5776486444628,40.2944300970907));
#32745=CARTESIAN_POINT('Ctrl Pts',(-40.0076871467891,37.6558156534542,40.3524402634908));
#32746=CARTESIAN_POINT('Ctrl Pts',(-40.0636544091168,37.7367610584931,40.408492489682));
#32747=CARTESIAN_POINT('Ctrl Pts',(-40.1176994696642,37.8202986143656,40.4624577781161));
#32748=CARTESIAN_POINT('Ctrl Pts',(-40.1717445302117,37.9038361702381,40.5164230665502));
#32749=CARTESIAN_POINT('Ctrl Pts',(-40.223867350847,37.989965818037,40.5683013791495));
#32750=CARTESIAN_POINT('Ctrl Pts',(-40.2739479686196,38.0784893933889,40.6179733119099));
#32751=CARTESIAN_POINT('Ctrl Pts',(-40.3240285863921,38.1670129687408,40.6676452446704));
#32752=CARTESIAN_POINT('Ctrl Pts',(-40.3720669659594,38.2579304092274,40.7151107625352));
#32753=CARTESIAN_POINT('Ctrl Pts',(-40.417952531741,38.3510325415251,40.7602606037133));
#32754=CARTESIAN_POINT('Ctrl Pts',(-40.4638380975226,38.4441346738228,40.8054104448913));
#32755=CARTESIAN_POINT('Ctrl Pts',(-40.5075708171276,38.5394214322887,40.8482445775075));
#32756=CARTESIAN_POINT('Ctrl Pts',(-40.5490500104958,38.6366735953907,40.8886643841204));
#32757=CARTESIAN_POINT('Ctrl Pts',(-40.590529203864,38.7339257584929,40.9290841907332));
#32758=CARTESIAN_POINT('Ctrl Pts',(-40.6297548417044,38.8331432576641,40.9670896427955));
#32759=CARTESIAN_POINT('Ctrl Pts',(-40.6666366022296,38.934097830037,41.002593220518));
#32760=CARTESIAN_POINT('Ctrl Pts',(-40.7035183627549,39.0350524024099,41.0380967982405));
#32761=CARTESIAN_POINT('Ctrl Pts',(-40.7380562199081,39.1377439768077,41.0710984765346));
#32762=CARTESIAN_POINT('Ctrl Pts',(-40.7701706254072,39.2419362974163,41.1015222356531));
#32763=CARTESIAN_POINT('Ctrl Pts',(-40.8022850309064,39.3461286180248,41.1319459947717));
#32764=CARTESIAN_POINT('Ctrl Pts',(-40.8319759620484,39.4518216113835,41.1597918131997));
#32765=CARTESIAN_POINT('Ctrl Pts',(-40.8591750098643,39.558772113834,41.1849955208619));
#32766=CARTESIAN_POINT('Ctrl Pts',(-40.8863740576804,39.6657226162845,41.2101992285241));
#32767=CARTESIAN_POINT('Ctrl Pts',(-40.9110812029252,39.773930552419,41.2327608075782));
#32768=CARTESIAN_POINT('Ctrl Pts',(-40.9332394906484,39.8831469675769,41.2526282328875));
#32769=CARTESIAN_POINT('Ctrl Pts',(-40.9553977783715,39.9923633827349,41.2724956581968));
#32770=CARTESIAN_POINT('Ctrl Pts',(-40.9750071928742,40.1025881999071,41.2896689156735));
#32771=CARTESIAN_POINT('Ctrl Pts',(-40.9920224953816,40.2135678168966,41.3041083646667));
#32772=CARTESIAN_POINT('Ctrl Pts',(-41.009037797889,40.3245474338861,41.31854781366));
#32773=CARTESIAN_POINT('Ctrl Pts',(-41.0234589763207,40.4362817724348,41.3302534439013));
#32774=CARTESIAN_POINT('Ctrl Pts',(-41.0352527164837,40.5485137476579,41.3391981819529));
#32775=CARTESIAN_POINT('Ctrl Pts',(-41.0470464566467,40.6607457228809,41.3481429200046));
#32776=CARTESIAN_POINT('Ctrl Pts',(-41.0562127501345,40.7734752556303,41.3543267594645));
#32777=CARTESIAN_POINT('Ctrl Pts',(-41.0627303610314,40.886442959227,41.3577353191749));
#32778=CARTESIAN_POINT('Ctrl Pts',(-41.0692479719283,40.9994106628236,41.3611438788854));
#32779=CARTESIAN_POINT('Ctrl Pts',(-41.0731168955402,41.1126164575932,41.361777156341));
#32780=CARTESIAN_POINT('Ctrl Pts',(-41.0743280725085,41.225799846588,41.3596335294917));
#32781=CARTESIAN_POINT('Ctrl Pts',(-41.0755392494769,41.3389832355827,41.3574899026424));
#32782=CARTESIAN_POINT('Ctrl Pts',(-41.0740926788428,41.452144138965,41.3525693728901));
#32783=CARTESIAN_POINT('Ctrl Pts',(-41.0699915202077,41.5650221462243,41.3448830855782));
#32784=CARTESIAN_POINT('Ctrl Pts',(-41.0658903615727,41.6779001534836,41.3371967982663));
#32785=CARTESIAN_POINT('Ctrl Pts',(-41.0591346177177,41.7904951849852,41.3267447586977));
#32786=CARTESIAN_POINT('Ctrl Pts',(-41.049739653545,41.9025481130374,41.3135508292975));
#32787=CARTESIAN_POINT('Ctrl Pts',(-41.040336339667,42.0147006273062,41.3003451738894));
#32788=CARTESIAN_POINT('Ctrl Pts',(-41.02828911873,42.126309994911,41.2843927620129));
#32789=CARTESIAN_POINT('Ctrl Pts',(-41.0136255646488,42.2371188766663,41.2657301618302));
#32790=CARTESIAN_POINT('Ctrl Pts',(-39.6924821306133,37.3539385160429,40.1901910998149));
#32791=CARTESIAN_POINT('Ctrl Pts',(-39.7550437057594,37.4279635608479,40.2533257828455));
#32792=CARTESIAN_POINT('Ctrl Pts',(-39.8158746486762,37.5050729659852,40.3145589119263));
#32793=CARTESIAN_POINT('Ctrl Pts',(-39.8748285637661,37.5850811601499,40.3737431235591));
#32794=CARTESIAN_POINT('Ctrl Pts',(-39.9337824788559,37.6650893543145,40.4329273351919));
#32795=CARTESIAN_POINT('Ctrl Pts',(-39.9908593205375,37.7479962756468,40.4900625836176));
#32796=CARTESIAN_POINT('Ctrl Pts',(-40.0459217278239,37.8336024005534,40.5450113672875));
#32797=CARTESIAN_POINT('Ctrl Pts',(-40.1009841351103,37.9192085254601,40.5999601509574));
#32798=CARTESIAN_POINT('Ctrl Pts',(-40.154032065429,38.0075137877534,40.652722427387));
#32799=CARTESIAN_POINT('Ctrl Pts',(-40.2049378537611,38.0983056722058,40.7031712190114));
#32800=CARTESIAN_POINT('Ctrl Pts',(-40.2558436420933,38.1890975566583,40.7536200106359));
#32801=CARTESIAN_POINT('Ctrl Pts',(-40.3046072490803,38.2823759930726,40.8017552784498));
#32802=CARTESIAN_POINT('Ctrl Pts',(-40.3511113203454,38.3779164977929,40.8474611802359));
#32803=CARTESIAN_POINT('Ctrl Pts',(-40.3976153916104,38.4734570025133,40.8931670820219));
#32804=CARTESIAN_POINT('Ctrl Pts',(-40.441859891198,38.5712595016707,40.9364435824419));
#32805=CARTESIAN_POINT('Ctrl Pts',(-40.4837383404043,38.671088624011,40.9771865323761));
#32806=CARTESIAN_POINT('Ctrl Pts',(-40.5256167896104,38.7709177463515,41.0179294823103));
#32807=CARTESIAN_POINT('Ctrl Pts',(-40.5651291560561,38.8727734146902,41.0561388502577));
#32808=CARTESIAN_POINT('Ctrl Pts',(-40.6021803493774,38.9764105034259,41.0917226816472));
#32809=CARTESIAN_POINT('Ctrl Pts',(-40.6392315426986,39.0800475921617,41.1273065130367));
#32810=CARTESIAN_POINT('Ctrl Pts',(-40.6738215342485,39.1854660211658,41.1602647803561));
#32811=CARTESIAN_POINT('Ctrl Pts',(-40.7058670798385,39.2924120907059,41.1905181663201));
#32812=CARTESIAN_POINT('Ctrl Pts',(-40.7379126254285,39.3993581602459,41.2207715522841));
#32813=CARTESIAN_POINT('Ctrl Pts',(-40.7674137002819,39.5078317876348,41.2483200335019));
#32814=CARTESIAN_POINT('Ctrl Pts',(-40.7942993071845,39.6175719205072,41.2730973118662));
#32815=CARTESIAN_POINT('Ctrl Pts',(-40.8211849140871,39.7273120533795,41.2978745902305));
#32816=CARTESIAN_POINT('Ctrl Pts',(-40.8454550322518,39.838318606888,41.3198806465843));
#32817=CARTESIAN_POINT('Ctrl Pts',(-40.8670512532719,39.9503244329335,41.3390625212065));
#32818=CARTESIAN_POINT('Ctrl Pts',(-40.8886474742919,40.0623302589791,41.3582443958287));
#32819=CARTESIAN_POINT('Ctrl Pts',(-40.9075697814698,40.1753352709624,41.3746020738885));
#32820=CARTESIAN_POINT('Ctrl Pts',(-40.9237726364277,40.2890675112993,41.3880961890381));
#32821=CARTESIAN_POINT('Ctrl Pts',(-40.9399754913854,40.4027997516363,41.4015903041876));
#32822=CARTESIAN_POINT('Ctrl Pts',(-40.9534588815956,40.5172591323928,41.4122208459937));
#32823=CARTESIAN_POINT('Ctrl Pts',(-40.9641903579644,40.6321701959042,41.4199622310205));
#32824=CARTESIAN_POINT('Ctrl Pts',(-40.9749218343331,40.7470812594156,41.4277036160472));
#32825=CARTESIAN_POINT('Ctrl Pts',(-40.9829013885633,40.8624439168365,41.4325558383094));
#32826=CARTESIAN_POINT('Ctrl Pts',(-40.9881098170792,40.9779805366789,41.4345072204607));
#32827=CARTESIAN_POINT('Ctrl Pts',(-40.9933182455951,41.0935171565213,41.436458602612));
#32828=CARTESIAN_POINT('Ctrl Pts',(-40.9957555443691,41.209227649457,41.4355091431444));
#32829=CARTESIAN_POINT('Ctrl Pts',(-40.9954158478053,41.3248335468961,41.4316611270233));
#32830=CARTESIAN_POINT('Ctrl Pts',(-40.9950761512415,41.4404394443352,41.4278131109023));
#32831=CARTESIAN_POINT('Ctrl Pts',(-40.9919594596027,41.5559406568948,41.4210665411031));
#32832=CARTESIAN_POINT('Ctrl Pts',(-40.9860732735097,41.6710592196427,41.4114376539052));
#32833=CARTESIAN_POINT('Ctrl Pts',(-40.9801870874168,41.7861777823904,41.4018087667073));
#32834=CARTESIAN_POINT('Ctrl Pts',(-40.9715314114214,41.9009136063195,41.3892975695548));
#32835=CARTESIAN_POINT('Ctrl Pts',(-40.9601270762523,42.0149905684778,41.3739341718642));
#32836=CARTESIAN_POINT('Ctrl Pts',(-40.9487126055641,42.129168915698,41.3585571200667));
#32837=CARTESIAN_POINT('Ctrl Pts',(-40.9345445966629,42.2426871411525,41.3403228076332));
#32838=CARTESIAN_POINT('Ctrl Pts',(-40.9176572009828,42.3552715649338,41.319275189134));
#32839=CARTESIAN_POINT('Ctrl Pts',(-39.6135628167506,37.3562205905267,40.2657183011866));
#32840=CARTESIAN_POINT('Ctrl Pts',(-39.6774756216741,37.4318340440419,40.3301997006854));
#32841=CARTESIAN_POINT('Ctrl Pts',(-39.7395834805726,37.510664296499,40.3926978931619));
#32842=CARTESIAN_POINT('Ctrl Pts',(-39.7997306457477,37.5925136758369,40.4530561500275));
#32843=CARTESIAN_POINT('Ctrl Pts',(-39.8598778109228,37.6743630551748,40.5134144068931));
#32844=CARTESIAN_POINT('Ctrl Pts',(-39.9180642319583,37.7592314928005,40.5716326775531));
#32845=CARTESIAN_POINT('Ctrl Pts',(-39.9741439859836,37.8469061867413,40.6275649564589));
#32846=CARTESIAN_POINT('Ctrl Pts',(-40.030223740009,37.9345808806821,40.6834972353646));
#32847=CARTESIAN_POINT('Ctrl Pts',(-40.0841967800109,38.0250617574698,40.7371434756245));
#32848=CARTESIAN_POINT('Ctrl Pts',(-40.1359277389027,38.1181219510228,40.7883691261129));
#32849=CARTESIAN_POINT('Ctrl Pts',(-40.1876586977945,38.2111821445759,40.8395947766013));
#32850=CARTESIAN_POINT('Ctrl Pts',(-40.2371475322013,38.3068215769179,40.8883997943643));
#32851=CARTESIAN_POINT('Ctrl Pts',(-40.2842701089497,38.4048004540608,40.9346617567584));
#32852=CARTESIAN_POINT('Ctrl Pts',(-40.3313926856981,38.5027793312036,40.9809237191525));
#32853=CARTESIAN_POINT('Ctrl Pts',(-40.3761489652685,38.6030975710527,41.0246425873763));
#32854=CARTESIAN_POINT('Ctrl Pts',(-40.4184266703127,38.7055036526314,41.0657086806318));
#32855=CARTESIAN_POINT('Ctrl Pts',(-40.4607043753569,38.8079097342101,41.1067747738874));
#32856=CARTESIAN_POINT('Ctrl Pts',(-40.500503470408,38.9124035717163,41.14518805772));
#32857=CARTESIAN_POINT('Ctrl Pts',(-40.5377240965251,39.0187231768149,41.1808521427764));
#32858=CARTESIAN_POINT('Ctrl Pts',(-40.5749447226423,39.1250427819136,41.2165162278329));
#32859=CARTESIAN_POINT('Ctrl Pts',(-40.609586848589,39.2331880655239,41.2494310841775));
#32860=CARTESIAN_POINT('Ctrl Pts',(-40.6415635342698,39.3428878839955,41.279514096987));
#32861=CARTESIAN_POINT('Ctrl Pts',(-40.6735402199505,39.4525877024671,41.3095971097965));
#32862=CARTESIAN_POINT('Ctrl Pts',(-40.7028514385154,39.563841963886,41.3368482538041));
#32863=CARTESIAN_POINT('Ctrl Pts',(-40.7294236045046,39.6763717271803,41.3611991028705));
#32864=CARTESIAN_POINT('Ctrl Pts',(-40.7559957704939,39.7889014904745,41.3855499519369));
#32865=CARTESIAN_POINT('Ctrl Pts',(-40.7798288615784,39.9027066613571,41.4070004855904));
#32866=CARTESIAN_POINT('Ctrl Pts',(-40.8008630158954,40.0175018982901,41.4254968095255));
#32867=CARTESIAN_POINT('Ctrl Pts',(-40.8218971702123,40.1322971352231,41.4439931334607));
#32868=CARTESIAN_POINT('Ctrl Pts',(-40.8401323700655,40.2480823420177,41.4595352321036));
#32869=CARTESIAN_POINT('Ctrl Pts',(-40.8555227774737,40.3645672057021,41.4720840134094));
#32870=CARTESIAN_POINT('Ctrl Pts',(-40.8709131848819,40.4810520693865,41.4846327947152));
#32871=CARTESIAN_POINT('Ctrl Pts',(-40.8834587868704,40.5982364923508,41.494188248086));
#32872=CARTESIAN_POINT('Ctrl Pts',(-40.893127999445,40.7158266441505,41.500726280088));
#32873=CARTESIAN_POINT('Ctrl Pts',(-40.9027972120195,40.8334167959504,41.5072643120899));
#32874=CARTESIAN_POINT('Ctrl Pts',(-40.9095900269921,40.9514125780428,41.5107849171542));
#32875=CARTESIAN_POINT('Ctrl Pts',(-40.913489273127,41.0695181141309,41.5112791217464));
#32876=CARTESIAN_POINT('Ctrl Pts',(-40.9173885192619,41.187623650219,41.5117733263386));
#32877=CARTESIAN_POINT('Ctrl Pts',(-40.918394193198,41.3058388413209,41.5092411299477));
#32878=CARTESIAN_POINT('Ctrl Pts',(-40.9165036231021,41.4238672472043,41.503688724555));
#32879=CARTESIAN_POINT('Ctrl Pts',(-40.9146130530062,41.5418956530876,41.4981363191623));
#32880=CARTESIAN_POINT('Ctrl Pts',(-40.9098262403625,41.6597371748247,41.489563709316));
#32881=CARTESIAN_POINT('Ctrl Pts',(-40.9021550268117,41.777096293061,41.4779922222321));
#32882=CARTESIAN_POINT('Ctrl Pts',(-40.8944838132608,41.8944554112973,41.4664207351483));
#32883=CARTESIAN_POINT('Ctrl Pts',(-40.8839282051252,42.0113320276539,41.4518503804119));
#32884=CARTESIAN_POINT('Ctrl Pts',(-40.8705144989597,42.1274330239181,41.4343175144308));
#32885=CARTESIAN_POINT('Ctrl Pts',(-40.8570888714613,42.2436372040898,41.4167690662439));
#32886=CARTESIAN_POINT('Ctrl Pts',(-40.8408000745959,42.3590642873939,41.3962528532535));
#32887=CARTESIAN_POINT('Ctrl Pts',(-40.8216888373169,42.4734242532013,41.3728202164377));
#32888=CARTESIAN_POINT('Ctrl Pts',(-39.5346528073732,37.3585135271757,40.341254653468));
#32889=CARTESIAN_POINT('Ctrl Pts',(-39.5998972885217,37.4356857994494,40.4070525688079));
#32890=CARTESIAN_POINT('Ctrl Pts',(-39.6632614971712,37.5162091132762,40.4707845113903));
#32891=CARTESIAN_POINT('Ctrl Pts',(-39.7245799035767,37.5998731232236,40.5322839864252));
#32892=CARTESIAN_POINT('Ctrl Pts',(-39.7858983099821,37.6835371331711,40.59378346146));
#32893=CARTESIAN_POINT('Ctrl Pts',(-39.8451708583676,37.7703417631542,40.6530504130031));
#32894=CARTESIAN_POINT('Ctrl Pts',(-39.9022426979749,37.8600602717383,40.7099299997107));
#32895=CARTESIAN_POINT('Ctrl Pts',(-39.9593145375822,37.9497787803222,40.7668095864183));
#32896=CARTESIAN_POINT('Ctrl Pts',(-40.0141856164902,38.042411085924,40.82130175654));
#32897=CARTESIAN_POINT('Ctrl Pts',(-40.0667125709269,38.1377152340127,40.8732641301578));
#32898=CARTESIAN_POINT('Ctrl Pts',(-40.1192395253635,38.2330193821015,40.9252265037756));
#32899=CARTESIAN_POINT('Ctrl Pts',(-40.1694223075328,38.3309952860207,40.9746590336024));
#32900=CARTESIAN_POINT('Ctrl Pts',(-40.2171297887776,38.4313870403645,41.0214325441754));
#32901=CARTESIAN_POINT('Ctrl Pts',(-40.2648372700223,38.5317787947084,41.0682060547483));
#32902=CARTESIAN_POINT('Ctrl Pts',(-40.3100694069207,38.634586308198,41.1123205034901));
#32903=CARTESIAN_POINT('Ctrl Pts',(-40.3527079902916,38.7395410595142,41.1536605936016));
#32904=CARTESIAN_POINT('Ctrl Pts',(-40.3953465736626,38.8444958108302,41.1950006837132));
#32905=CARTESIAN_POINT('Ctrl Pts',(-40.4353915646849,38.9515977045472,41.2335663775487));
#32906=CARTESIAN_POINT('Ctrl Pts',(-40.4727382906827,39.0605670041845,41.2692568588486));
#32907=CARTESIAN_POINT('Ctrl Pts',(-40.5100850166805,39.1695363038219,41.3049473401485));
#32908=CARTESIAN_POINT('Ctrl Pts',(-40.5447334436354,39.2803729103039,41.3377625763946));
#32909=CARTESIAN_POINT('Ctrl Pts',(-40.5765929818585,39.3927873312385,41.3676167582733));
#32910=CARTESIAN_POINT('Ctrl Pts',(-40.6084525200816,39.5052017521732,41.3974709401519));
#32911=CARTESIAN_POINT('Ctrl Pts',(-40.6375231405345,39.6191938853506,41.424364040442));
#32912=CARTESIAN_POINT('Ctrl Pts',(-40.6637288096024,39.7344659926158,41.448225704969));
#32913=CARTESIAN_POINT('Ctrl Pts',(-40.6899344786702,39.8497380998812,41.472087369496));
#32914=CARTESIAN_POINT('Ctrl Pts',(-40.7132751724454,39.9662900764232,41.4929175764786));
#32915=CARTESIAN_POINT('Ctrl Pts',(-40.7336898106128,40.0838174915083,41.5106617945233));
#32916=CARTESIAN_POINT('Ctrl Pts',(-40.7541044487802,40.2013449065934,41.5284060125681));
#32917=CARTESIAN_POINT('Ctrl Pts',(-40.7715930126886,40.3198476533541,41.5430642254468));
#32918=CARTESIAN_POINT('Ctrl Pts',(-40.786109694613,40.4390161966153,41.5545980097256));
#32919=CARTESIAN_POINT('Ctrl Pts',(-40.8006263765375,40.5581847398765,41.5661317940043));
#32920=CARTESIAN_POINT('Ctrl Pts',(-40.8121711631813,40.6780189712691,41.5745411390913));
#32921=CARTESIAN_POINT('Ctrl Pts',(-40.8207137591026,40.7982058659919,41.5798039307316));
#32922=CARTESIAN_POINT('Ctrl Pts',(-40.8292563550239,40.9183927607145,41.585066722372));
#32923=CARTESIAN_POINT('Ctrl Pts',(-40.834796752349,41.0389322094628,41.587182955667));
#32924=CARTESIAN_POINT('Ctrl Pts',(-40.8373203267629,41.1595093308912,41.5861469417492));
#32925=CARTESIAN_POINT('Ctrl Pts',(-40.8398439011769,41.2800864523198,41.5851109278313));
#32926=CARTESIAN_POINT('Ctrl Pts',(-40.8393506502698,41.4007011367585,41.5809226675212));
#32927=CARTESIAN_POINT('Ctrl Pts',(-40.835841698011,41.5210382891738,41.5735929279324));
#32928=CARTESIAN_POINT('Ctrl Pts',(-40.8323327457522,41.6413754415893,41.5662631883435));
#32929=CARTESIAN_POINT('Ctrl Pts',(-40.825808095209,41.761434952516,41.5557919760115));
#32930=CARTESIAN_POINT('Ctrl Pts',(-40.8162846137041,41.8809031572982,41.5422064588396));
#32931=CARTESIAN_POINT('Ctrl Pts',(-40.8067611321992,42.0003713620803,41.5286209416676));
#32932=CARTESIAN_POINT('Ctrl Pts',(-40.7942388282604,42.1192481520286,41.5119211318735));
#32933=CARTESIAN_POINT('Ctrl Pts',(-40.778750225565,42.2372229295778,41.492150457457));
#32934=CARTESIAN_POINT('Ctrl Pts',(-40.7632478574878,42.3553025563437,41.472362211999));
#32935=CARTESIAN_POINT('Ctrl Pts',(-40.7447739297299,42.4724784591441,41.4494976589433));
#32936=CARTESIAN_POINT('Ctrl Pts',(-40.723376581818,42.5884439120029,41.4236164196056));
#32937=CARTESIAN_POINT('Ctrl Pts',(-39.4557619421374,37.3608288129201,40.4168098339066));
#32938=CARTESIAN_POINT('Ctrl Pts',(-39.5223241949095,37.4395364367563,40.4838988547304));
#32939=CARTESIAN_POINT('Ctrl Pts',(-39.5869297733209,37.5217312603981,40.5488379555043));
#32940=CARTESIAN_POINT('Ctrl Pts',(-39.6494029164308,37.6071896709646,40.6114504679323));
#32941=CARTESIAN_POINT('Ctrl Pts',(-39.7118760595407,37.6926480815311,40.6740629803604));
#32942=CARTESIAN_POINT('Ctrl Pts',(-39.772216705614,37.7813699945731,40.7343488425698));
#32943=CARTESIAN_POINT('Ctrl Pts',(-39.830260696555,37.873114040115,40.7921440455055));
#32944=CARTESIAN_POINT('Ctrl Pts',(-39.888304687496,37.9648580856568,40.8499392484413));
#32945=CARTESIAN_POINT('Ctrl Pts',(-39.9440519659463,38.0596241730381,40.905243734991));
#32946=CARTESIAN_POINT('Ctrl Pts',(-39.9973508701712,38.1571544889698,40.9579070480451));
#32947=CARTESIAN_POINT('Ctrl Pts',(-40.0506497743961,38.2546848049014,41.0105703610992));
#32948=CARTESIAN_POINT('Ctrl Pts',(-40.1015002517261,38.3549792530051,41.0605924486165));
#32949=CARTESIAN_POINT('Ctrl Pts',(-40.149763962285,38.457764979961,41.1078372243739));
#32950=CARTESIAN_POINT('Ctrl Pts',(-40.1980276728438,38.5605507069169,41.1550820001313));
#32951=CARTESIAN_POINT('Ctrl Pts',(-40.2437045689378,38.6658276111535,41.199549417442));
#32952=CARTESIAN_POINT('Ctrl Pts',(-40.2866703855357,38.773309284466,41.2411185016893));
#32953=CARTESIAN_POINT('Ctrl Pts',(-40.3296362021336,38.8807909577785,41.2826875859365));
#32954=CARTESIAN_POINT('Ctrl Pts',(-40.369890896777,38.9904772939548,41.3213582960421));
#32955=CARTESIAN_POINT('Ctrl Pts',(-40.4073249556566,39.1020698888309,41.3570254274626));
#32956=CARTESIAN_POINT('Ctrl Pts',(-40.4447590145362,39.2136624837069,41.3926925588832));
#32957=CARTESIAN_POINT('Ctrl Pts',(-40.4793724006601,39.327161227008,41.4253560763727));
#32958=CARTESIAN_POINT('Ctrl Pts',(-40.5110709475265,39.4422573428303,41.4549271180914));
#32959=CARTESIAN_POINT('Ctrl Pts',(-40.542769494393,39.5573534586525,41.4844981598102));
#32960=CARTESIAN_POINT('Ctrl Pts',(-40.571553170678,39.674046833259,41.5109766965364));
#32961=CARTESIAN_POINT('Ctrl Pts',(-40.5973436697376,39.7920199996788,41.5342906928107));
#32962=CARTESIAN_POINT('Ctrl Pts',(-40.6231341687972,39.9099931660986,41.5576046890849));
#32963=CARTESIAN_POINT('Ctrl Pts',(-40.6459314651451,40.0292460077526,41.5777541218692));
#32964=CARTESIAN_POINT('Ctrl Pts',(-40.6656735382207,40.1494540945804,41.5946841741736));
#32965=CARTESIAN_POINT('Ctrl Pts',(-40.6854156112962,40.2696621814082,41.611614226478));
#32966=CARTESIAN_POINT('Ctrl Pts',(-40.7021024415902,40.390825394622,41.625324881573));
#32967=CARTESIAN_POINT('Ctrl Pts',(-40.7156886322023,40.5126141069537,41.6357788393107));
#32968=CARTESIAN_POINT('Ctrl Pts',(-40.7292748228144,40.6344028192854,41.6462327970483));
#32969=CARTESIAN_POINT('Ctrl Pts',(-40.7397603603196,40.7568169103839,41.6534300470975));
#32970=CARTESIAN_POINT('Ctrl Pts',(-40.7471167185743,40.8795233499408,41.6573510091775));
#32971=CARTESIAN_POINT('Ctrl Pts',(-40.754473076829,41.0022297894977,41.6612719712575));
#32972=CARTESIAN_POINT('Ctrl Pts',(-40.7587002485643,41.1252284562551,41.6619166414932));
#32973=CARTESIAN_POINT('Ctrl Pts',(-40.7597867336636,41.2481847295518,41.6592832660444));
#32974=CARTESIAN_POINT('Ctrl Pts',(-40.7608732187629,41.3711410028484,41.6566498905956));
#32975=CARTESIAN_POINT('Ctrl Pts',(-40.7588190161525,41.4940547611804,41.6507384720647));
#32976=CARTESIAN_POINT('Ctrl Pts',(-40.7536297143373,41.6165916148816,41.6415650925998));
#32977=CARTESIAN_POINT('Ctrl Pts',(-40.7484404125221,41.7391284685829,41.6323917131349));
#32978=CARTESIAN_POINT('Ctrl Pts',(-40.74011601663,41.8612882965639,41.619956381801));
#32979=CARTESIAN_POINT('Ctrl Pts',(-40.7286791733688,41.9827387602433,41.6042929291989));
#32980=CARTESIAN_POINT('Ctrl Pts',(-40.7172423301077,42.1041892239226,41.5886294765968));
#32981=CARTESIAN_POINT('Ctrl Pts',(-40.7026930507781,42.2249302032856,41.5697379182055));
#32982=CARTESIAN_POINT('Ctrl Pts',(-40.6850709170265,42.3446332197583,41.5476696489369));
#32983=CARTESIAN_POINT('Ctrl Pts',(-40.6674331217329,42.4644426214073,41.525581766656));
#32984=CARTESIAN_POINT('Ctrl Pts',(-40.6467170250815,42.583212095883,41.5003115462781));
#32985=CARTESIAN_POINT('Ctrl Pts',(-40.6229790784524,42.7006179510356,41.4719278505636));
#32986=CARTESIAN_POINT('Ctrl Pts',(-39.3768710769017,37.3631440986644,40.4923650143452));
#32987=CARTESIAN_POINT('Ctrl Pts',(-39.4447511012974,37.4433870740631,40.5607451406529));
#32988=CARTESIAN_POINT('Ctrl Pts',(-39.5105980494706,37.52725340752,40.6268913996182));
#32989=CARTESIAN_POINT('Ctrl Pts',(-39.574225929285,37.6145062187056,40.6906169494395));
#32990=CARTESIAN_POINT('Ctrl Pts',(-39.6378538090993,37.7017590298911,40.7543424992609));
#32991=CARTESIAN_POINT('Ctrl Pts',(-39.6992625528604,37.7923982259919,40.8156472721364));
#32992=CARTESIAN_POINT('Ctrl Pts',(-39.7582786951351,37.8861678084917,40.8743580913004));
#32993=CARTESIAN_POINT('Ctrl Pts',(-39.8172948374097,37.9799373909914,40.9330689104643));
#32994=CARTESIAN_POINT('Ctrl Pts',(-39.8739183154024,38.0768372601523,40.9891857134419));
#32995=CARTESIAN_POINT('Ctrl Pts',(-39.9279891694155,38.1765937439268,41.0425499659323));
#32996=CARTESIAN_POINT('Ctrl Pts',(-39.9820600234286,38.2763502277013,41.0959142184228));
#32997=CARTESIAN_POINT('Ctrl Pts',(-40.0335781959193,38.3789632199894,41.1465258636306));
#32998=CARTESIAN_POINT('Ctrl Pts',(-40.0823981357924,38.4841429195575,41.1942419045724));
#32999=CARTESIAN_POINT('Ctrl Pts',(-40.1312180756654,38.5893226191255,41.2419579455143));
#33000=CARTESIAN_POINT('Ctrl Pts',(-40.177339730955,38.6970689141089,41.286778331394));
#33001=CARTESIAN_POINT('Ctrl Pts',(-40.2206327807798,38.8070775094178,41.328576409777));
#33002=CARTESIAN_POINT('Ctrl Pts',(-40.2639258306046,38.9170861047267,41.3703744881599));
#33003=CARTESIAN_POINT('Ctrl Pts',(-40.3043902288691,39.0293568833625,41.4091502145356));
#33004=CARTESIAN_POINT('Ctrl Pts',(-40.3419116206305,39.1435727734772,41.4447939960767));
#33005=CARTESIAN_POINT('Ctrl Pts',(-40.3794330123919,39.2577886635919,41.4804377776179));
#33006=CARTESIAN_POINT('Ctrl Pts',(-40.4140113576848,39.3739495437122,41.5129495763508));
#33007=CARTESIAN_POINT('Ctrl Pts',(-40.4455489131946,39.491727354422,41.5422374779096));
#33008=CARTESIAN_POINT('Ctrl Pts',(-40.4770864687044,39.6095051651317,41.5715253794685));
#33009=CARTESIAN_POINT('Ctrl Pts',(-40.5055832008214,39.7288997811675,41.5975893526308));
#33010=CARTESIAN_POINT('Ctrl Pts',(-40.5309585298728,39.8495740067417,41.6203556806524));
#33011=CARTESIAN_POINT('Ctrl Pts',(-40.5563338589242,39.9702482323161,41.6431220086739));
#33012=CARTESIAN_POINT('Ctrl Pts',(-40.5785877578449,40.0922019390821,41.6625906672598));
#33013=CARTESIAN_POINT('Ctrl Pts',(-40.5976572658285,40.2150906976525,41.6787065538238));
#33014=CARTESIAN_POINT('Ctrl Pts',(-40.6167267738122,40.3379794562229,41.6948224403878));
#33015=CARTESIAN_POINT('Ctrl Pts',(-40.6326118704917,40.46180313589,41.7075855376992));
#33016=CARTESIAN_POINT('Ctrl Pts',(-40.6452675697915,40.5862120172922,41.7169596688957));
#33017=CARTESIAN_POINT('Ctrl Pts',(-40.6579232690913,40.7106208986944,41.7263338000923));
#33018=CARTESIAN_POINT('Ctrl Pts',(-40.667349557458,40.8356148494986,41.7323189551036));
#33019=CARTESIAN_POINT('Ctrl Pts',(-40.6735196780461,40.9608408338897,41.7348980876234));
#33020=CARTESIAN_POINT('Ctrl Pts',(-40.6796897986341,41.0860668182808,41.737477220143));
#33021=CARTESIAN_POINT('Ctrl Pts',(-40.6826037447796,41.2115247030474,41.7366503273193));
#33022=CARTESIAN_POINT('Ctrl Pts',(-40.6822531405642,41.3368601282123,41.7324195903396));
#33023=CARTESIAN_POINT('Ctrl Pts',(-40.6819025363488,41.4621955533772,41.72818885336));
#33024=CARTESIAN_POINT('Ctrl Pts',(-40.6782873820352,41.5874083856024,41.7205542766081));
#33025=CARTESIAN_POINT('Ctrl Pts',(-40.6714177306635,41.7121449405895,41.7095372572672));
#33026=CARTESIAN_POINT('Ctrl Pts',(-40.6645480792919,41.8368814955765,41.6985202379262));
#33027=CARTESIAN_POINT('Ctrl Pts',(-40.6544239380509,41.9611416406117,41.6841207875904));
#33028=CARTESIAN_POINT('Ctrl Pts',(-40.6410737330335,42.0845743631883,41.6663793995582));
#33029=CARTESIAN_POINT('Ctrl Pts',(-40.6277235280161,42.208007085765,41.6486380115259));
#33030=CARTESIAN_POINT('Ctrl Pts',(-40.6111472732959,42.3306122545426,41.6275547045377));
#33031=CARTESIAN_POINT('Ctrl Pts',(-40.5913916084879,42.4520435099388,41.6031888404167));
#33032=CARTESIAN_POINT('Ctrl Pts',(-40.5716183859781,42.573582686471,41.5788013213131));
#33033=CARTESIAN_POINT('Ctrl Pts',(-40.5486601204331,42.6939457326218,41.5511254336129));
#33034=CARTESIAN_POINT('Ctrl Pts',(-40.5225815750869,42.8127919900683,41.5202392815215));
#33035=CARTESIAN_POINT('Ctrl Pts',(-39.2979993170057,37.3654816882064,40.5679389847796));
#33036=CARTESIAN_POINT('Ctrl Pts',(-39.367183179944,37.4472365158672,40.6375847800584));
#33037=CARTESIAN_POINT('Ctrl Pts',(-39.4342564894374,37.5327527754326,40.7049115791748));
#33038=CARTESIAN_POINT('Ctrl Pts',(-39.4990225730245,37.6217797250398,40.7697219594771));
#33039=CARTESIAN_POINT('Ctrl Pts',(-39.5637886566116,37.7108066746471,40.8345323397794));
#33040=CARTESIAN_POINT('Ctrl Pts',(-39.6262474400391,37.8033442122469,40.8968262269577));
#33041=CARTESIAN_POINT('Ctrl Pts',(-39.6862157711,37.8991210217028,40.9564209445738));
#33042=CARTESIAN_POINT('Ctrl Pts',(-39.746184102161,37.9948978311585,41.0160156621899));
#33043=CARTESIAN_POINT('Ctrl Pts',(-39.8036619120932,38.0939138026928,41.0729111419033));
#33044=CARTESIAN_POINT('Ctrl Pts',(-39.8584806419644,38.1958786351937,41.1269405237714));
#33045=CARTESIAN_POINT('Ctrl Pts',(-39.9132993718355,38.2978434676945,41.1809699056395));
#33046=CARTESIAN_POINT('Ctrl Pts',(-39.9654589587768,38.4027570442984,41.2321331276911));
#33047=CARTESIAN_POINT('Ctrl Pts',(-40.0148064247347,38.5103117793659,41.2802801241842));
#33048=CARTESIAN_POINT('Ctrl Pts',(-40.0641538906926,38.6178665144333,41.3284271206772));
#33049=CARTESIAN_POINT('Ctrl Pts',(-40.1106891790595,38.7280622846981,41.3735578363725));
#33050=CARTESIAN_POINT('Ctrl Pts',(-40.1542757890722,38.840576021645,41.4155398791369));
#33051=CARTESIAN_POINT('Ctrl Pts',(-40.1978623990849,38.9530897585918,41.4575219219013));
#33052=CARTESIAN_POINT('Ctrl Pts',(-40.2385002807281,39.0679213332727,41.4963552435508));
#33053=CARTESIAN_POINT('Ctrl Pts',(-40.2760702105016,39.1847340866154,41.5319259015271));
#33054=CARTESIAN_POINT('Ctrl Pts',(-40.3136401402752,39.3015468399581,41.5674965595035));
#33055=CARTESIAN_POINT('Ctrl Pts',(-40.3481420750489,39.420340638087,41.5998045129599));
#33056=CARTESIAN_POINT('Ctrl Pts',(-40.3794747674399,39.5407672032934,41.6287549368956));
#33057=CARTESIAN_POINT('Ctrl Pts',(-40.410807459831,39.6611937684996,41.6577053608314));
#33058=CARTESIAN_POINT('Ctrl Pts',(-40.4389708738467,39.7832529627628,41.683298221976));
#33059=CARTESIAN_POINT('Ctrl Pts',(-40.4638823318658,39.9065869297263,41.7054583689751));
#33060=CARTESIAN_POINT('Ctrl Pts',(-40.4887937898849,40.0299208966897,41.7276185159742));
#33061=CARTESIAN_POINT('Ctrl Pts',(-40.5104532632632,40.1545294949953,41.7463459233285));
#33062=CARTESIAN_POINT('Ctrl Pts',(-40.5287971291004,40.280047385766,41.7615855542687));
#33063=CARTESIAN_POINT('Ctrl Pts',(-40.5471409949375,40.4055652765367,41.7768251852089));
#33064=CARTESIAN_POINT('Ctrl Pts',(-40.5621692321055,40.5319923159037,41.7885770221565));
#33065=CARTESIAN_POINT('Ctrl Pts',(-40.5738376458591,40.6589578224765,41.7968064661327));
#33066=CARTESIAN_POINT('Ctrl Pts',(-40.5855060596127,40.7859233290494,41.8050359101089));
#33067=CARTESIAN_POINT('Ctrl Pts',(-40.5938146364638,40.91342715729,41.8097429515589));
#33068=CARTESIAN_POINT('Ctrl Pts',(-40.5987388695419,41.0410954546661,41.8109136328711));
#33069=CARTESIAN_POINT('Ctrl Pts',(-40.60366310262,41.1687637520422,41.8120843141834));
#33070=CARTESIAN_POINT('Ctrl Pts',(-40.6052029861564,41.2965963721973,41.8097186338833));
#33071=CARTESIAN_POINT('Ctrl Pts',(-40.603353845636,41.4242184814935,41.8038233584774));
#33072=CARTESIAN_POINT('Ctrl Pts',(-40.6015047051155,41.5518405907898,41.7979280830714));
#33073=CARTESIAN_POINT('Ctrl Pts',(-40.5962665425231,41.6792520429083,41.7885032191744));
#33074=CARTESIAN_POINT('Ctrl Pts',(-40.5876545440908,41.8060792189963,41.7755762188468));
#33075=CARTESIAN_POINT('Ctrl Pts',(-40.5790425456584,41.9329063950843,41.7626492185191));
#33076=CARTESIAN_POINT('Ctrl Pts',(-40.567056721113,42.0591491497169,41.7462200964266));
#33077=CARTESIAN_POINT('Ctrl Pts',(-40.5517320295636,42.1844372677281,41.7263368305228));
#33078=CARTESIAN_POINT('Ctrl Pts',(-40.5364073380141,42.3097253857393,41.7064535646191));
#33079=CARTESIAN_POINT('Ctrl Pts',(-40.5177437968734,42.4340587234487,41.6831161775353));
#33080=CARTESIAN_POINT('Ctrl Pts',(-40.4957959345014,42.5570726384864,41.6563928932872));
#33081=CARTESIAN_POINT('Ctrl Pts',(-40.473828566128,42.6801958812373,41.6296458589165));
#33082=CARTESIAN_POINT('Ctrl Pts',(-40.4485710611385,42.8019972136734,41.5995069368439));
#33083=CARTESIAN_POINT('Ctrl Pts',(-40.420097395835,42.9221187503367,41.5660644338022));
#33084=CARTESIAN_POINT('Ctrl Pts',(-39.2191560456546,37.3678525356093,40.6435409735397));
#33085=CARTESIAN_POINT('Ctrl Pts',(-39.289634570114,37.4511005411706,40.7144304990469));
#33086=CARTESIAN_POINT('Ctrl Pts',(-39.3579239195882,37.5382500908353,40.7829146422872));
#33087=CARTESIAN_POINT('Ctrl Pts',(-39.423816267808,37.6290359607303,40.848784984172));
#33088=CARTESIAN_POINT('Ctrl Pts',(-39.4897086160278,37.7198218306253,40.9146553260567));
#33089=CARTESIAN_POINT('Ctrl Pts',(-39.5532038814973,37.8142439084663,40.9779117851173));
#33090=CARTESIAN_POINT('Ctrl Pts',(-39.614108827874,37.9120148377575,41.0383618517751));
#33091=CARTESIAN_POINT('Ctrl Pts',(-39.6750137742507,38.0097857670486,41.0988119184329));
#33092=CARTESIAN_POINT('Ctrl Pts',(-39.7333283262069,38.1109054268666,41.156455517923));
#33093=CARTESIAN_POINT('Ctrl Pts',(-39.7888750139637,38.2150660778376,41.2111172223887));
#33094=CARTESIAN_POINT('Ctrl Pts',(-39.8444217017204,38.3192267288085,41.2657789268544));
#33095=CARTESIAN_POINT('Ctrl Pts',(-39.8972004565773,38.4264282421062,41.3174586686899));
#33096=CARTESIAN_POINT('Ctrl Pts',(-39.9470506559512,38.5363443693372,41.365999169959));
#33097=CARTESIAN_POINT('Ctrl Pts',(-39.9969008553251,38.6462604965682,41.4145396712281));
#33098=CARTESIAN_POINT('Ctrl Pts',(-40.043822437561,38.7588911017878,41.4599408718959));
#33099=CARTESIAN_POINT('Ctrl Pts',(-40.0876726053202,38.8738934141444,41.5020646016294));
#33100=CARTESIAN_POINT('Ctrl Pts',(-40.1315227730794,38.988895726501,41.544188331363));
#33101=CARTESIAN_POINT('Ctrl Pts',(-40.1723014721277,39.1062696037593,41.5830345380635));
#33102=CARTESIAN_POINT('Ctrl Pts',(-40.2098845998788,39.2256578397782,41.6184850003352));
#33103=CARTESIAN_POINT('Ctrl Pts',(-40.2474677276301,39.345046075797,41.6539354626069));
#33104=CARTESIAN_POINT('Ctrl Pts',(-40.2818552376011,39.4664485229166,41.6859901366046));
#33105=CARTESIAN_POINT('Ctrl Pts',(-40.3129424776325,39.589495714773,41.7145514697324));
#33106=CARTESIAN_POINT('Ctrl Pts',(-40.3440297176639,39.7125429066293,41.7431128028603));
#33107=CARTESIAN_POINT('Ctrl Pts',(-40.3718166493068,39.837234691037,41.7681807597935));
#33108=CARTESIAN_POINT('Ctrl Pts',(-40.3962187080664,39.96319159113,41.7896790507446));
#33109=CARTESIAN_POINT('Ctrl Pts',(-40.420620766826,40.0891484912228,41.8111773416957));
#33110=CARTESIAN_POINT('Ctrl Pts',(-40.4416379225217,40.2163703512169,41.8291059400754));
#33111=CARTESIAN_POINT('Ctrl Pts',(-40.4592062132462,40.3444699944187,41.8434102834412));
#33112=CARTESIAN_POINT('Ctrl Pts',(-40.4767745039706,40.4725696376205,41.8577146268069));
#33113=CARTESIAN_POINT('Ctrl Pts',(-40.4908939079951,40.601546905596,41.8683946974671));
#33114=CARTESIAN_POINT('Ctrl Pts',(-40.5015214554703,40.7310092793855,41.8754179925605));
#33115=CARTESIAN_POINT('Ctrl Pts',(-40.5121490029456,40.8604716531751,41.882441287654));
#33116=CARTESIAN_POINT('Ctrl Pts',(-40.5192846807273,40.9904189726592,41.8858077984942));
#33117=CARTESIAN_POINT('Ctrl Pts',(-40.5229067726725,41.120455766702,41.8855072797153));
#33118=CARTESIAN_POINT('Ctrl Pts',(-40.5265288646176,41.2504925607449,41.8852067609363));
#33119=CARTESIAN_POINT('Ctrl Pts',(-40.5266373662463,41.3806186685165,41.8812392129097));
#33120=CARTESIAN_POINT('Ctrl Pts',(-40.5232319473535,41.5104380747713,41.8736167101495));
#33121=CARTESIAN_POINT('Ctrl Pts',(-40.5198265284606,41.6402574810262,41.8659942073892));
#33122=CARTESIAN_POINT('Ctrl Pts',(-40.5129071932581,41.7697700252033,41.8547167593229));
#33123=CARTESIAN_POINT('Ctrl Pts',(-40.5024949994896,41.8985815593266,41.8398186868216));
#33124=CARTESIAN_POINT('Ctrl Pts',(-40.4920828057211,42.02739309345,41.8249206143203));
#33125=CARTESIAN_POINT('Ctrl Pts',(-40.4781777662645,42.155503458205,41.8064019358099));
#33126=CARTESIAN_POINT('Ctrl Pts',(-40.4608221985893,42.2825227728951,41.7843190095351));
#33127=CARTESIAN_POINT('Ctrl Pts',(-40.4434666309142,42.4095420875853,41.7622360832603));
#33128=CARTESIAN_POINT('Ctrl Pts',(-40.422660556486,42.5354701951125,41.7365889365334));
#33129=CARTESIAN_POINT('Ctrl Pts',(-40.3984672948247,42.6599238560849,41.7074556218011));
#33130=CARTESIAN_POINT('Ctrl Pts',(-40.3742525315798,42.7844881243341,41.6782964150494));
#33131=CARTESIAN_POINT('Ctrl Pts',(-40.3466445877264,42.9075751698582,41.6456448770227));
#33132=CARTESIAN_POINT('Ctrl Pts',(-40.3157276232668,43.0288097293944,41.6096005440156));
#33133=CARTESIAN_POINT('Ctrl Pts',(-39.1403127743034,37.3702233830122,40.7191429622998));
#33134=CARTESIAN_POINT('Ctrl Pts',(-39.2120859602839,37.4549645664739,40.7912762180353));
#33135=CARTESIAN_POINT('Ctrl Pts',(-39.2815913497389,37.5437474062381,40.8609177053995));
#33136=CARTESIAN_POINT('Ctrl Pts',(-39.3486099625915,37.6362921964208,40.9278480088668));
#33137=CARTESIAN_POINT('Ctrl Pts',(-39.4156285754441,37.7288369866036,40.9947783123341));
#33138=CARTESIAN_POINT('Ctrl Pts',(-39.4801603229556,37.8251436046857,41.0589973432769));
#33139=CARTESIAN_POINT('Ctrl Pts',(-39.542001884648,37.9249086538123,41.1203027589764));
#33140=CARTESIAN_POINT('Ctrl Pts',(-39.6038434463403,38.0246737029389,41.1816081746759));
#33141=CARTESIAN_POINT('Ctrl Pts',(-39.6629947403206,38.1278970510403,41.2399998939428));
#33142=CARTESIAN_POINT('Ctrl Pts',(-39.719269385963,38.2342535204814,41.2952939210061));
#33143=CARTESIAN_POINT('Ctrl Pts',(-39.7755440316054,38.3406099899225,41.3505879480694));
#33144=CARTESIAN_POINT('Ctrl Pts',(-39.8289419543779,38.450099439914,41.4027842096886));
#33145=CARTESIAN_POINT('Ctrl Pts',(-39.8792948871678,38.5623769593085,41.4517182157338));
#33146=CARTESIAN_POINT('Ctrl Pts',(-39.9296478199576,38.6746544787031,41.500652221779));
#33147=CARTESIAN_POINT('Ctrl Pts',(-39.9769556960625,38.7897199188775,41.5463239074193));
#33148=CARTESIAN_POINT('Ctrl Pts',(-40.0210694215682,38.9072108066439,41.5885893241219));
#33149=CARTESIAN_POINT('Ctrl Pts',(-40.0651831470738,39.0247016944102,41.6308547408246));
#33150=CARTESIAN_POINT('Ctrl Pts',(-40.1061026635273,39.1446178742459,41.6697138325762));
#33151=CARTESIAN_POINT('Ctrl Pts',(-40.1436989892561,39.2665815929409,41.7050440991433));
#33152=CARTESIAN_POINT('Ctrl Pts',(-40.1812953149849,39.3885453116359,41.7403743657104));
#33153=CARTESIAN_POINT('Ctrl Pts',(-40.2155684001534,39.5125564077462,41.7721757602493));
#33154=CARTESIAN_POINT('Ctrl Pts',(-40.2464101878252,39.6382242262525,41.8003480025693));
#33155=CARTESIAN_POINT('Ctrl Pts',(-40.2772519754969,39.7638920447589,41.8285202448892));
#33156=CARTESIAN_POINT('Ctrl Pts',(-40.3046624247669,39.8912164193113,41.853063297611));
#33157=CARTESIAN_POINT('Ctrl Pts',(-40.328555084267,40.0197962525337,41.8738997325141));
#33158=CARTESIAN_POINT('Ctrl Pts',(-40.3524477437671,40.1483760857561,41.8947361674171));
#33159=CARTESIAN_POINT('Ctrl Pts',(-40.3728225817804,40.2782112074384,41.9118659568223));
#33160=CARTESIAN_POINT('Ctrl Pts',(-40.389615297392,40.4088926030714,41.9252350126137));
#33161=CARTESIAN_POINT('Ctrl Pts',(-40.4064080130036,40.5395739987043,41.938604068405));
#33162=CARTESIAN_POINT('Ctrl Pts',(-40.4196185838847,40.6711014952883,41.9482123727777));
#33163=CARTESIAN_POINT('Ctrl Pts',(-40.4292052650816,40.8030607362945,41.9540295189884));
#33164=CARTESIAN_POINT('Ctrl Pts',(-40.4387919462785,40.9350199773008,41.9598466651991));
#33165=CARTESIAN_POINT('Ctrl Pts',(-40.4447547249909,41.0674107880283,41.9618726454296));
#33166=CARTESIAN_POINT('Ctrl Pts',(-40.4470746758031,41.199816078738,41.9601009265594));
#33167=CARTESIAN_POINT('Ctrl Pts',(-40.4493946266152,41.3322213694475,41.9583292076891));
#33168=CARTESIAN_POINT('Ctrl Pts',(-40.4480717463362,41.4646409648356,41.9527597919361));
#33169=CARTESIAN_POINT('Ctrl Pts',(-40.4431100490709,41.5966576680492,41.9434100618216));
#33170=CARTESIAN_POINT('Ctrl Pts',(-40.4381483518057,41.7286743712627,41.9340603317071));
#33171=CARTESIAN_POINT('Ctrl Pts',(-40.429547843993,41.8602880074982,41.9209302994716));
#33172=CARTESIAN_POINT('Ctrl Pts',(-40.4173354548884,41.9910838996568,41.9040611547965));
#33173=CARTESIAN_POINT('Ctrl Pts',(-40.4051230657838,42.1218797918155,41.8871920101214));
#33174=CARTESIAN_POINT('Ctrl Pts',(-40.3892988114159,42.2518577666931,41.8665837751932));
#33175=CARTESIAN_POINT('Ctrl Pts',(-40.3699123676151,42.3806082780621,41.8423011885474));
#33176=CARTESIAN_POINT('Ctrl Pts',(-40.3505259238143,42.5093587894312,41.8180186019016));
#33177=CARTESIAN_POINT('Ctrl Pts',(-40.3275773160987,42.6368816667763,41.7900616955314));
#33178=CARTESIAN_POINT('Ctrl Pts',(-40.301138655148,42.7627750736833,41.7585183503151));
#33179=CARTESIAN_POINT('Ctrl Pts',(-40.2746764970317,42.8887803674308,41.7269469711824));
#33180=CARTESIAN_POINT('Ctrl Pts',(-40.2447181143144,43.0131531260429,41.6917828172015));
#33181=CARTESIAN_POINT('Ctrl Pts',(-40.2113578506985,43.1355007084522,41.6531366542289));
#33182=CARTESIAN_POINT('Ctrl Pts',(-39.0614979606134,37.3726274522223,40.794772939012));
#33183=CARTESIAN_POINT('Ctrl Pts',(-39.1345566113031,37.4588431187849,40.8681279710931));
#33184=CARTESIAN_POINT('Ctrl Pts',(-39.2052676996424,37.5492425921423,40.9389035914507));
#33185=CARTESIAN_POINT('Ctrl Pts',(-39.2734006183025,37.6435310639275,41.0068689724951));
#33186=CARTESIAN_POINT('Ctrl Pts',(-39.3415335369625,37.7378195357127,41.0748343535394));
#33187=CARTESIAN_POINT('Ctrl Pts',(-39.4070881892784,37.8359968721725,41.1399893988339));
#33188=CARTESIAN_POINT('Ctrl Pts',(-39.4698507733057,37.9377429133658,41.2021215990047));
#33189=CARTESIAN_POINT('Ctrl Pts',(-39.532613357333,38.039488954559,41.2642537991755));
#33190=CARTESIAN_POINT('Ctrl Pts',(-39.5925837840149,38.1448035561639,41.3233630660502));
#33191=CARTESIAN_POINT('Ctrl Pts',(-39.6495664502885,38.2533432931017,41.3792565936186));
#33192=CARTESIAN_POINT('Ctrl Pts',(-39.706549116562,38.3618830300396,41.435150121187));
#33193=CARTESIAN_POINT('Ctrl Pts',(-39.7605439415582,38.4736477483594,41.4878278301146));
#33194=CARTESIAN_POINT('Ctrl Pts',(-39.8113747960734,38.5882729958286,41.537117874583));
#33195=CARTESIAN_POINT('Ctrl Pts',(-39.8622056505885,38.7028982432979,41.5864079190514));
#33196=CARTESIAN_POINT('Ctrl Pts',(-39.909872462468,38.8203838573381,41.6323102290807));
#33197=CARTESIAN_POINT('Ctrl Pts',(-39.9542197245262,38.9403467335296,41.6746750393716));
#33198=CARTESIAN_POINT('Ctrl Pts',(-39.9985669865844,39.060309609721,41.7170398496625));
#33199=CARTESIAN_POINT('Ctrl Pts',(-40.0395946358509,39.1827495779158,41.7558671000453));
#33200=CARTESIAN_POINT('Ctrl Pts',(-40.0771688010238,39.3072673780001,41.7910300822715));
#33201=CARTESIAN_POINT('Ctrl Pts',(-40.1147429661966,39.4317851780843,41.8261930644977));
#33202=CARTESIAN_POINT('Ctrl Pts',(-40.1488635938993,39.5583806334479,41.8576917285996));
#33203=CARTESIAN_POINT('Ctrl Pts',(-40.1794193216837,39.6866409300556,41.8854232497566));
#33204=CARTESIAN_POINT('Ctrl Pts',(-40.209975049468,39.8149012266631,41.9131547709135));
#33205=CARTESIAN_POINT('Ctrl Pts',(-40.2369658338992,39.9448261825921,41.9371191096854));
#33206=CARTESIAN_POINT('Ctrl Pts',(-40.2603035477718,40.0759921200064,41.9572379955189));
#33207=CARTESIAN_POINT('Ctrl Pts',(-40.2836412616445,40.2071580574208,41.9773568813524));
#33208=CARTESIAN_POINT('Ctrl Pts',(-40.3033258717486,40.339564790269,41.9936302855921));
#33209=CARTESIAN_POINT('Ctrl Pts',(-40.3192930611983,40.4727805378766,42.006005002883));
#33210=CARTESIAN_POINT('Ctrl Pts',(-40.3352602506479,40.6059962854843,42.0183797201739));
#33211=CARTESIAN_POINT('Ctrl Pts',(-40.3475099966744,40.740020858882,42.0268557328322));
#33212=CARTESIAN_POINT('Ctrl Pts',(-40.3560022127269,40.8744171883912,42.0314052483924));
#33213=CARTESIAN_POINT('Ctrl Pts',(-40.3644944287794,41.0088135179004,42.0359547639526));
#33214=CARTESIAN_POINT('Ctrl Pts',(-40.3692291026792,41.1435814128636,42.036577775818));
#33215=CARTESIAN_POINT('Ctrl Pts',(-40.3701906404258,41.2782813629928,42.0332720865946));
#33216=CARTESIAN_POINT('Ctrl Pts',(-40.3711521781724,41.412981313122,42.0299663973711));
#33217=CARTESIAN_POINT('Ctrl Pts',(-40.3683405782567,41.5476131273126,42.0227320115925));
#33218=CARTESIAN_POINT('Ctrl Pts',(-40.3617648419301,41.6817377190824,42.0115923424155));
#33219=CARTESIAN_POINT('Ctrl Pts',(-40.3551891056035,41.8158623108523,42.0004526732384));
#33220=CARTESIAN_POINT('Ctrl Pts',(-40.3448492420369,41.9494794898936,41.9854077362983));
#33221=CARTESIAN_POINT('Ctrl Pts',(-40.330778790245,42.0821534553238,41.9665064039702));
#33222=CARTESIAN_POINT('Ctrl Pts',(-40.3167083384531,42.2148274207539,41.947605071642));
#33223=CARTESIAN_POINT('Ctrl Pts',(-40.2989073182277,42.3465579843004,41.9248473705619));
#33224=CARTESIAN_POINT('Ctrl Pts',(-40.2774335890346,42.476915471224,41.898307315156));
#33225=CARTESIAN_POINT('Ctrl Pts',(-40.2559598598415,42.6072729581475,41.8717672597502));
#33226=CARTESIAN_POINT('Ctrl Pts',(-40.2308134519652,42.7362571834365,41.8414448874824));
#33227=CARTESIAN_POINT('Ctrl Pts',(-40.2020761695918,42.8634473992982,41.8074388738828));
#33228=CARTESIAN_POINT('Ctrl Pts',(-40.1733133471698,42.9907506545297,41.7734026376885));
#33229=CARTESIAN_POINT('Ctrl Pts',(-40.1409533053408,43.1162565292245,41.7356762577682));
#33230=CARTESIAN_POINT('Ctrl Pts',(-40.1051015420806,43.2395548537019,41.6943827565721));
#33231=CARTESIAN_POINT('Ctrl Pts',(-38.9827210478865,37.375075767461,40.8704401911112));
#33232=CARTESIAN_POINT('Ctrl Pts',(-39.0570601865467,37.4627511375271,40.9449975555894));
#33233=CARTESIAN_POINT('Ctrl Pts',(-39.1289707770862,37.554754637862,41.0168865246252));
#33234=CARTESIAN_POINT('Ctrl Pts',(-39.1982100815384,37.650775705829,41.0858644332364));
#33235=CARTESIAN_POINT('Ctrl Pts',(-39.2674493859905,37.746796773796,41.1548423418474));
#33236=CARTESIAN_POINT('Ctrl Pts',(-39.3340172989842,37.8468352632664,41.2209090850606));
#33237=CARTESIAN_POINT('Ctrl Pts',(-39.3976891170407,37.9505534890766,41.283841651122));
#33238=CARTESIAN_POINT('Ctrl Pts',(-39.4613609350971,38.0542717148869,41.3467742171832));
#33239=CARTESIAN_POINT('Ctrl Pts',(-39.5221365613181,38.1616695191946,41.4065725103194));
#33240=CARTESIAN_POINT('Ctrl Pts',(-39.5798108443924,38.272384375083,41.4630346782584));
#33241=CARTESIAN_POINT('Ctrl Pts',(-39.6374851274667,38.3830992309714,41.5194968461974));
#33242=CARTESIAN_POINT('Ctrl Pts',(-39.6920579796234,38.4971309699505,41.5726228030128));
#33243=CARTESIAN_POINT('Ctrl Pts',(-39.7433451873401,38.6140946719095,41.6222332192534));
#33244=CARTESIAN_POINT('Ctrl Pts',(-39.7946323950568,38.7310583738686,41.6718436354939));
#33245=CARTESIAN_POINT('Ctrl Pts',(-39.8426338802826,38.8509538608077,41.7179384356605));
#33246=CARTESIAN_POINT('Ctrl Pts',(-39.8871876114888,38.9733764192277,41.7603620243398));
#33247=CARTESIAN_POINT('Ctrl Pts',(-39.9317413426949,39.0957989776476,41.802785613019));
#33248=CARTESIAN_POINT('Ctrl Pts',(-39.9728472520778,39.220748421241,41.8415379256489));
#33249=CARTESIAN_POINT('Ctrl Pts',(-40.0103665844861,39.3478029766131,41.8764881517675));
#33250=CARTESIAN_POINT('Ctrl Pts',(-40.0478859168944,39.4748575319852,41.911438377886));
#33251=CARTESIAN_POINT('Ctrl Pts',(-40.0818186152298,39.6040170057794,41.9425864643046));
#33252=CARTESIAN_POINT('Ctrl Pts',(-40.1120501378908,39.7348454134234,41.9698272690252));
#33253=CARTESIAN_POINT('Ctrl Pts',(-40.1422816605518,39.8656738210674,41.9970680737459));
#33254=CARTESIAN_POINT('Ctrl Pts',(-40.168811961531,39.9981709634615,42.0204015553124));
#33255=CARTESIAN_POINT('Ctrl Pts',(-40.191551486407,40.1318895895581,42.039748950335));
#33256=CARTESIAN_POINT('Ctrl Pts',(-40.2142910112829,40.2656082156547,42.0590963453575));
#33257=CARTESIAN_POINT('Ctrl Pts',(-40.2332397254499,40.4005481219555,42.0744576243926));
#33258=CARTESIAN_POINT('Ctrl Pts',(-40.2483336665301,40.5362538117355,42.0857809346378));
#33259=CARTESIAN_POINT('Ctrl Pts',(-40.2634276076103,40.6719595015155,42.0971042448829));
#33260=CARTESIAN_POINT('Ctrl Pts',(-40.2746667526333,40.8084307682524,42.104389569106));
#33261=CARTESIAN_POINT('Ctrl Pts',(-40.2820131632761,40.9452069460336,42.1076123153132));
#33262=CARTESIAN_POINT('Ctrl Pts',(-40.2893595739188,41.0819831238149,42.1108350615203));
#33263=CARTESIAN_POINT('Ctrl Pts',(-40.2928132390013,41.2190640044892,42.1099952248072));
#33264=CARTESIAN_POINT('Ctrl Pts',(-40.2923625004959,41.3559868643603,42.1050956400864));
#33265=CARTESIAN_POINT('Ctrl Pts',(-40.2919117619906,41.4929097242314,42.1001960553657));
#33266=CARTESIAN_POINT('Ctrl Pts',(-40.2875566205834,41.6296743549245,42.0912367300939));
#33267=CARTESIAN_POINT('Ctrl Pts',(-40.2793117772825,41.765819100262,42.0782479069429));
#33268=CARTESIAN_POINT('Ctrl Pts',(-40.2710669339815,41.9019638455995,42.0652590837918));
#33269=CARTESIAN_POINT('Ctrl Pts',(-40.2589324013341,42.0374884983907,42.0482407825286));
#33270=CARTESIAN_POINT('Ctrl Pts',(-40.242949140091,42.1719355880683,42.0272504493207));
#33271=CARTESIAN_POINT('Ctrl Pts',(-40.2269658788481,42.3063826777458,42.0062601161129));
#33272=CARTESIAN_POINT('Ctrl Pts',(-40.2071339133334,42.4397519997028,41.9812977829045));
#33273=CARTESIAN_POINT('Ctrl Pts',(-40.1835201873859,42.5715933588039,41.9524477113593));
#33274=CARTESIAN_POINT('Ctrl Pts',(-40.1599064614385,42.7034347179049,41.9235976398141));
#33275=CARTESIAN_POINT('Ctrl Pts',(-40.1325110109945,42.8337479135088,41.8908598738373));
#33276=CARTESIAN_POINT('Ctrl Pts',(-40.1014263108327,42.9620930665946,41.8543449214736));
#33277=CARTESIAN_POINT('Ctrl Pts',(-40.070313984372,43.0905522854922,41.8177975167142));
#33278=CARTESIAN_POINT('Ctrl Pts',(-40.0355058950823,43.2170397664827,41.77746626436));
#33279=CARTESIAN_POINT('Ctrl Pts',(-39.9971197373371,43.3411277792636,41.7334875353997));
#33280=CARTESIAN_POINT('Ctrl Pts',(-38.9039441351597,37.3775240826997,40.9461074432104));
#33281=CARTESIAN_POINT('Ctrl Pts',(-38.9795637617903,37.4666591562693,41.0218671400858));
#33282=CARTESIAN_POINT('Ctrl Pts',(-39.05267385453,37.5602666835818,41.0948694577997));
#33283=CARTESIAN_POINT('Ctrl Pts',(-39.1230195447743,37.6580203477305,41.1648598939777));
#33284=CARTESIAN_POINT('Ctrl Pts',(-39.1933652350185,37.7557740118792,41.2348503301556));
#33285=CARTESIAN_POINT('Ctrl Pts',(-39.26094640869,37.8576736543604,41.3018287712874));
#33286=CARTESIAN_POINT('Ctrl Pts',(-39.3255274607756,37.9633640647876,41.3655617032392));
#33287=CARTESIAN_POINT('Ctrl Pts',(-39.3901085128612,38.0690544752149,41.429294635191));
#33288=CARTESIAN_POINT('Ctrl Pts',(-39.4516893386213,38.1785354822252,41.4897819545887));
#33289=CARTESIAN_POINT('Ctrl Pts',(-39.5100552384964,38.2914254570642,41.5468127628983));
#33290=CARTESIAN_POINT('Ctrl Pts',(-39.5684211383714,38.4043154319032,41.6038435712078));
#33291=CARTESIAN_POINT('Ctrl Pts',(-39.6235720176885,38.5206141915416,41.657417775911));
#33292=CARTESIAN_POINT('Ctrl Pts',(-39.6753155786067,38.6399163479905,41.7073485639237));
#33293=CARTESIAN_POINT('Ctrl Pts',(-39.727059139525,38.7592185044393,41.7572793519365));
#33294=CARTESIAN_POINT('Ctrl Pts',(-39.7753952980973,38.8815238642774,41.8035666422404));
#33295=CARTESIAN_POINT('Ctrl Pts',(-39.8201554984513,39.0064061049258,41.846049009308));
#33296=CARTESIAN_POINT('Ctrl Pts',(-39.8649156988054,39.1312883455742,41.8885313763755));
#33297=CARTESIAN_POINT('Ctrl Pts',(-39.9060998683047,39.2587472645661,41.9272087512526));
#33298=CARTESIAN_POINT('Ctrl Pts',(-39.9435643679485,39.388338575226,41.9619462212635));
#33299=CARTESIAN_POINT('Ctrl Pts',(-39.9810288675922,39.517929885886,41.9966836912744));
#33300=CARTESIAN_POINT('Ctrl Pts',(-40.0147736365603,39.6496533781108,42.0274812000097));
#33301=CARTESIAN_POINT('Ctrl Pts',(-40.044680954098,39.7830498967912,42.0542312882939));
#33302=CARTESIAN_POINT('Ctrl Pts',(-40.0745882716357,39.9164464154717,42.0809813765782));
#33303=CARTESIAN_POINT('Ctrl Pts',(-40.1006580891627,40.0515157443309,42.1036840009393));
#33304=CARTESIAN_POINT('Ctrl Pts',(-40.122799425042,40.1877870591098,42.1222599051509));
#33305=CARTESIAN_POINT('Ctrl Pts',(-40.1449407609214,40.3240583738885,42.1408358093627));
#33306=CARTESIAN_POINT('Ctrl Pts',(-40.1631535791511,40.461531453642,42.1552849631931));
#33307=CARTESIAN_POINT('Ctrl Pts',(-40.1773742718619,40.5997270855943,42.1655568663926));
#33308=CARTESIAN_POINT('Ctrl Pts',(-40.1915949645728,40.7379227175466,42.175828769592));
#33309=CARTESIAN_POINT('Ctrl Pts',(-40.2018235085922,40.8768406776228,42.1819234053797));
#33310=CARTESIAN_POINT('Ctrl Pts',(-40.2080241138252,41.0159967036761,42.1838193822339));
#33311=CARTESIAN_POINT('Ctrl Pts',(-40.2142247190582,41.1551527297295,42.185715359088));
#33312=CARTESIAN_POINT('Ctrl Pts',(-40.2163973753233,41.2945465961149,42.1834126737962));
#33313=CARTESIAN_POINT('Ctrl Pts',(-40.214534360566,41.4336923657278,42.1769191935783));
#33314=CARTESIAN_POINT('Ctrl Pts',(-40.2126713458088,41.5728381353406,42.1704257133604));
#33315=CARTESIAN_POINT('Ctrl Pts',(-40.2067726629101,41.7117355825366,42.1597414485952));
#33316=CARTESIAN_POINT('Ctrl Pts',(-40.1968587126348,41.8499004814415,42.1449034714703));
#33317=CARTESIAN_POINT('Ctrl Pts',(-40.1869447623595,41.9880653803465,42.1300654943453));
#33318=CARTESIAN_POINT('Ctrl Pts',(-40.1730155606313,42.1254975068878,42.1110738287589));
#33319=CARTESIAN_POINT('Ctrl Pts',(-40.1551194899372,42.2617177208127,42.0879944946714));
#33320=CARTESIAN_POINT('Ctrl Pts',(-40.137223419243,42.3979379347377,42.0649151605838));
#33321=CARTESIAN_POINT('Ctrl Pts',(-40.1153605084391,42.5329460151051,42.0377481952471));
#33322=CARTESIAN_POINT('Ctrl Pts',(-40.0896067857373,42.6662712463838,42.0065881075625));
#33323=CARTESIAN_POINT('Ctrl Pts',(-40.0638530630355,42.7995964776624,41.9754280198779));
#33324=CARTESIAN_POINT('Ctrl Pts',(-40.0342085700239,42.931238643581,41.9402748601922));
#33325=CARTESIAN_POINT('Ctrl Pts',(-40.0007764520737,43.060738733891,41.9012509690643));
#33326=CARTESIAN_POINT('Ctrl Pts',(-39.9673146215742,43.1903539164548,41.8621923957399));
#33327=CARTESIAN_POINT('Ctrl Pts',(-39.9300584848238,43.317823003741,41.8192562709516));
#33328=CARTESIAN_POINT('Ctrl Pts',(-39.8891379325936,43.4427007048253,41.7725923142273));
#33329=CARTESIAN_POINT('Ctrl Pts',(-38.8252050953863,37.3800166112679,41.0218119431493));
#33330=CARTESIAN_POINT('Ctrl Pts',(-38.9021002180776,37.4705965953422,41.0987545205423));
#33331=CARTESIAN_POINT('Ctrl Pts',(-38.9764036011982,37.5657955295521,41.1728493947268));
#33332=CARTESIAN_POINT('Ctrl Pts',(-39.0478477421773,37.6652706909476,41.2438298005602));
#33333=CARTESIAN_POINT('Ctrl Pts',(-39.1192918831564,37.764745852343,41.3148102063937));
#33334=CARTESIAN_POINT('Ctrl Pts',(-39.1878766584313,37.8684970689033,41.3826760211015));
#33335=CARTESIAN_POINT('Ctrl Pts',(-39.2533551414358,37.9761508429034,41.4471828923901));
#33336=CARTESIAN_POINT('Ctrl Pts',(-39.3188336244404,38.0838046169035,41.5116897636787));
#33337=CARTESIAN_POINT('Ctrl Pts',(-39.3812057019163,38.1953607621915,41.5728375799556));
#33338=CARTESIAN_POINT('Ctrl Pts',(-39.440246800283,38.3104176938053,41.6304061603406));
#33339=CARTESIAN_POINT('Ctrl Pts',(-39.4992878986496,38.4254746254192,41.6879747407256));
#33340=CARTESIAN_POINT('Ctrl Pts',(-39.5549979157674,38.5440321444137,41.7419639856107));
#33341=CARTESIAN_POINT('Ctrl Pts',(-39.6071762472742,38.6656634681541,41.7921794702661));
#33342=CARTESIAN_POINT('Ctrl Pts',(-39.6593545787809,38.7872947918946,41.8423949549214));
#33343=CARTESIAN_POINT('Ctrl Pts',(-39.7080011343898,38.9119997100725,41.8888365924393));
#33344=CARTESIAN_POINT('Ctrl Pts',(-39.7529407228233,39.0393293132054,41.9313371137559));
#33345=CARTESIAN_POINT('Ctrl Pts',(-39.7978803112568,39.1666589163385,41.9738376350724));
#33346=CARTESIAN_POINT('Ctrl Pts',(-39.8391128547301,39.2966129842659,42.0123969666053));
#33347=CARTESIAN_POINT('Ctrl Pts',(-39.8764898361686,39.4287237106721,42.046876199188));
#33348=CARTESIAN_POINT('Ctrl Pts',(-39.913866817607,39.5608344370783,42.0813554317706));
#33349=CARTESIAN_POINT('Ctrl Pts',(-39.9473881722875,39.6951015935328,42.1117545056753));
#33350=CARTESIAN_POINT('Ctrl Pts',(-39.976933126641,39.8310418428766,42.1379638719202));
#33351=CARTESIAN_POINT('Ctrl Pts',(-40.0064780809946,39.9669820922203,42.1641732381651));
#33352=CARTESIAN_POINT('Ctrl Pts',(-40.0320465838252,40.1045951993949,42.1861928513067));
#33353=CARTESIAN_POINT('Ctrl Pts',(-40.0535464748672,40.243385774172,42.2039433116964));
#33354=CARTESIAN_POINT('Ctrl Pts',(-40.0750463659091,40.3821763489492,42.2216937720859));
#33355=CARTESIAN_POINT('Ctrl Pts',(-40.0924776078616,40.5221441513319,42.2351750488915));
#33356=CARTESIAN_POINT('Ctrl Pts',(-40.1057773177963,40.6627853025867,42.2443384641273));
#33357=CARTESIAN_POINT('Ctrl Pts',(-40.1190770277309,40.8034264538415,42.2535018793631));
#33358=CARTESIAN_POINT('Ctrl Pts',(-40.1282451825109,40.9447407107577,42.2583474170307));
#33359=CARTESIAN_POINT('Ctrl Pts',(-40.1332486300361,41.0862193318304,42.258857472199));
#33360=CARTESIAN_POINT('Ctrl Pts',(-40.1382520775612,41.2276979529032,42.2593675273673));
#33361=CARTESIAN_POINT('Ctrl Pts',(-40.1390908090258,41.3693406934561,42.2555420989869));
#33362=CARTESIAN_POINT('Ctrl Pts',(-40.1357616428395,41.5106376100576,42.2473947830991));
#33363=CARTESIAN_POINT('Ctrl Pts',(-40.1324324766533,41.651934526659,42.2392474672111));
#33364=CARTESIAN_POINT('Ctrl Pts',(-40.1249354184051,41.7928853749258,42.2267782777238));
#33365=CARTESIAN_POINT('Ctrl Pts',(-40.1132972811551,41.9329826791417,42.2100319151659));
#33366=CARTESIAN_POINT('Ctrl Pts',(-40.101659143905,42.0730799833576,42.1932855526079));
#33367=CARTESIAN_POINT('Ctrl Pts',(-40.0858799475973,42.2123235011892,42.1722620457457));
#33368=CARTESIAN_POINT('Ctrl Pts',(-40.0660163083583,42.3502118766985,42.1470368793923));
#33369=CARTESIAN_POINT('Ctrl Pts',(-40.0461526691193,42.4881002522078,42.121811713039));
#33370=CARTESIAN_POINT('Ctrl Pts',(-40.0222046211057,42.6246332468531,42.0923849306128));
#33371=CARTESIAN_POINT('Ctrl Pts',(-39.9942581775686,42.759319232706,42.0588622595791));
#33372=CARTESIAN_POINT('Ctrl Pts',(-39.9663117340315,42.8940052185588,42.0253395885454));
#33373=CARTESIAN_POINT('Ctrl Pts',(-39.9343669430954,43.0268439625842,41.9877210866631));
#33374=CARTESIAN_POINT('Ctrl Pts',(-39.8985385977431,43.1573571033234,41.9461419648695));
#33375=CARTESIAN_POINT('Ctrl Pts',(-39.8626784102122,43.2879862366576,41.9045258899368));
#33376=CARTESIAN_POINT('Ctrl Pts',(-39.8229278240937,43.4162854048886,41.8589422238337));
#33377=CARTESIAN_POINT('Ctrl Pts',(-39.7794299686218,43.541791724316,41.8095551265968));
#33378=CARTESIAN_POINT('Ctrl Pts',(-38.7465138697966,37.3825649586746,41.0975634680728));
#33379=CARTESIAN_POINT('Ctrl Pts',(-38.8246834400008,37.4745783163285,41.1756711667335));
#33380=CARTESIAN_POINT('Ctrl Pts',(-38.9001777621614,37.5713594409668,41.2508394067609));
#33381=CARTESIAN_POINT('Ctrl Pts',(-38.9727161601587,37.6725485154566,41.3227887243575));
#33382=CARTESIAN_POINT('Ctrl Pts',(-39.045254558156,37.7737375899464,41.3947380419541));
#33383=CARTESIAN_POINT('Ctrl Pts',(-39.1148368980517,37.8793344274476,41.4634683042695));
#33384=CARTESIAN_POINT('Ctrl Pts',(-39.1812044835543,37.9889464353815,41.5287239829036));
#33385=CARTESIAN_POINT('Ctrl Pts',(-39.2475720690568,38.0985584433153,41.5939796615378));
#33386=CARTESIAN_POINT('Ctrl Pts',(-39.3107247776221,38.2121854192892,41.6557606359997));
#33387=CARTESIAN_POINT('Ctrl Pts',(-39.3704278173254,38.3294049159214,41.7138372142582));
#33388=CARTESIAN_POINT('Ctrl Pts',(-39.4301308570288,38.4466244125535,41.7719137925167));
#33389=CARTESIAN_POINT('Ctrl Pts',(-39.4863841176318,38.5674362134046,41.8262858673365));
#33390=CARTESIAN_POINT('Ctrl Pts',(-39.5389784582816,38.6913911590341,41.8767512918204));
#33391=CARTESIAN_POINT('Ctrl Pts',(-39.5915727989315,38.8153461046634,41.9272167163044));
#33392=CARTESIAN_POINT('Ctrl Pts',(-39.6405081225157,38.9424439661952,41.9737753972707));
#33393=CARTESIAN_POINT('Ctrl Pts',(-39.6856024951302,39.0722122135953,42.0162542368022));
#33394=CARTESIAN_POINT('Ctrl Pts',(-39.7306968677448,39.2019804609954,42.0587330763338));
#33395=CARTESIAN_POINT('Ctrl Pts',(-39.7719502061255,39.3344188546537,42.0971319959957));
#33396=CARTESIAN_POINT('Ctrl Pts',(-39.8092091367918,39.4690350092704,42.1313082345913));
#33397=CARTESIAN_POINT('Ctrl Pts',(-39.8464680674581,39.6036511638872,42.1654844731869));
#33398=CARTESIAN_POINT('Ctrl Pts',(-39.8797325216134,39.7404448309009,42.1954379676116));
#33399=CARTESIAN_POINT('Ctrl Pts',(-39.9088788272033,39.8789074327843,42.221057355443));
#33400=CARTESIAN_POINT('Ctrl Pts',(-39.9380251327931,40.0173700346678,42.2466767432743));
#33401=CARTESIAN_POINT('Ctrl Pts',(-39.9630532360005,40.1575013157574,42.2679619772076));
#33402=CARTESIAN_POINT('Ctrl Pts',(-39.9838700862395,40.2987802897971,42.2848339220615));
#33403=CARTESIAN_POINT('Ctrl Pts',(-40.0046869364786,40.4400592638367,42.3017058669153));
#33404=CARTESIAN_POINT('Ctrl Pts',(-40.0212924953122,40.5824856699626,42.3141644915366));
#33405=CARTESIAN_POINT('Ctrl Pts',(-40.0336250258616,40.7255299890016,42.3221634767014));
#33406=CARTESIAN_POINT('Ctrl Pts',(-40.0459575564109,40.8685743080405,42.3301624618662));
#33407=CARTESIAN_POINT('Ctrl Pts',(-40.0540170359046,41.012236275869,42.3337017928048));
#33408=CARTESIAN_POINT('Ctrl Pts',(-40.0577735004543,41.1559817796882,42.3327683108365));
#33409=CARTESIAN_POINT('Ctrl Pts',(-40.0615299650041,41.2997272835074,42.3318348288682));
#33410=CARTESIAN_POINT('Ctrl Pts',(-40.0609834076738,41.4435560578991,42.3264285357167));
#33411=CARTESIAN_POINT('Ctrl Pts',(-40.0561358604786,41.5869333699035,42.3165695311371));
#33412=CARTESIAN_POINT('Ctrl Pts',(-40.0512883132832,41.730310681908,42.3067105265574));
#33413=CARTESIAN_POINT('Ctrl Pts',(-40.0421397851736,41.8732362667868,42.2923988287537));
#33414=CARTESIAN_POINT('Ctrl Pts',(-40.0287242889509,42.0151787494982,42.2736876463871));
#33415=CARTESIAN_POINT('Ctrl Pts',(-40.0153087927281,42.1571212322096,42.2549764640206));
#33416=CARTESIAN_POINT('Ctrl Pts',(-39.9976263531632,42.2980803506645,42.2318658316403));
#33417=CARTESIAN_POINT('Ctrl Pts',(-39.9757427108098,42.4375320408366,42.2044416709745));
#33418=CARTESIAN_POINT('Ctrl Pts',(-39.9538590684562,42.5769837310087,42.1770175103087));
#33419=CARTESIAN_POINT('Ctrl Pts',(-39.9277742637211,42.7149277354081,42.1452798719946));
#33420=CARTESIAN_POINT('Ctrl Pts',(-39.8975852758416,42.8508511997324,42.1093467516234));
#33421=CARTESIAN_POINT('Ctrl Pts',(-39.8673962879621,42.9867746640567,42.0734136312522));
#33422=CARTESIAN_POINT('Ctrl Pts',(-39.8331031726806,43.1206773373308,42.0332850951724));
#33423=CARTESIAN_POINT('Ctrl Pts',(-39.7948334264531,43.2520613902913,41.989110335025));
#33424=CARTESIAN_POINT('Ctrl Pts',(-39.7565296682699,43.3835622098636,41.9448963148841));
#33425=CARTESIAN_POINT('Ctrl Pts',(-39.7142422783854,43.5125396872975,41.8966289570872));
#33426=CARTESIAN_POINT('Ctrl Pts',(-39.6681287411246,43.6385134433798,41.8444880178527));
#33427=CARTESIAN_POINT('Ctrl Pts',(-38.6678226442069,37.3851133060814,41.1733149929962));
#33428=CARTESIAN_POINT('Ctrl Pts',(-38.7472666619239,37.4785600373149,41.2525878129248));
#33429=CARTESIAN_POINT('Ctrl Pts',(-38.8239519231248,37.5769233523815,41.3288294187951));
#33430=CARTESIAN_POINT('Ctrl Pts',(-38.8975845781402,37.6798263399656,41.4017476481549));
#33431=CARTESIAN_POINT('Ctrl Pts',(-38.9712172331556,37.7827293275497,41.4746658775147));
#33432=CARTESIAN_POINT('Ctrl Pts',(-39.0417971376721,37.890171785992,41.5442605874375));
#33433=CARTESIAN_POINT('Ctrl Pts',(-39.1090538256727,38.0017420278596,41.6102650734172));
#33434=CARTESIAN_POINT('Ctrl Pts',(-39.1763105136732,38.1133122697273,41.6762695593968));
#33435=CARTESIAN_POINT('Ctrl Pts',(-39.2402438533279,38.229010076387,41.7386836920437));
#33436=CARTESIAN_POINT('Ctrl Pts',(-39.3006088343679,38.3483921380374,41.7972682681757));
#33437=CARTESIAN_POINT('Ctrl Pts',(-39.3609738154079,38.4677741996879,41.8558528443076));
#33438=CARTESIAN_POINT('Ctrl Pts',(-39.4177703194962,38.5908402823956,41.9106077490624));
#33439=CARTESIAN_POINT('Ctrl Pts',(-39.4707806692892,38.717118849914,41.9613231133749));
#33440=CARTESIAN_POINT('Ctrl Pts',(-39.5237910190821,38.8433974174324,42.0120384776873));
#33441=CARTESIAN_POINT('Ctrl Pts',(-39.5730151106415,38.972888222318,42.058714202102));
#33442=CARTESIAN_POINT('Ctrl Pts',(-39.6182642674372,39.1050951139852,42.1011713598486));
#33443=CARTESIAN_POINT('Ctrl Pts',(-39.6635134242329,39.2373020056522,42.1436285175952));
#33444=CARTESIAN_POINT('Ctrl Pts',(-39.704787557521,39.3722247250415,42.1818670253862));
#33445=CARTESIAN_POINT('Ctrl Pts',(-39.7419284374151,39.5093463078688,42.2157402699947));
#33446=CARTESIAN_POINT('Ctrl Pts',(-39.7790693173092,39.646467890696,42.2496135146032));
#33447=CARTESIAN_POINT('Ctrl Pts',(-39.8120768709394,39.7857880682689,42.2791214295479));
#33448=CARTESIAN_POINT('Ctrl Pts',(-39.8408245277656,39.9267730226921,42.3041508389658));
#33449=CARTESIAN_POINT('Ctrl Pts',(-39.8695721845917,40.0677579771153,42.3291802483837));
#33450=CARTESIAN_POINT('Ctrl Pts',(-39.8940598881757,40.2104074321199,42.3497311031085));
#33451=CARTESIAN_POINT('Ctrl Pts',(-39.9141936976119,40.3541748054221,42.3657245324266));
#33452=CARTESIAN_POINT('Ctrl Pts',(-39.9343275070481,40.4979421787244,42.3817179617447));
#33453=CARTESIAN_POINT('Ctrl Pts',(-39.9501073827628,40.6428271885933,42.3931539341818));
#33454=CARTESIAN_POINT('Ctrl Pts',(-39.9614727339269,40.7882746754164,42.3999884892756));
#33455=CARTESIAN_POINT('Ctrl Pts',(-39.9728380850908,40.9337221622395,42.4068230443694));
#33456=CARTESIAN_POINT('Ctrl Pts',(-39.9797888892982,41.0797318409803,42.4090561685789));
#33457=CARTESIAN_POINT('Ctrl Pts',(-39.9822983708726,41.225744227546,42.406679149474));
#33458=CARTESIAN_POINT('Ctrl Pts',(-39.9848078524469,41.3717566141116,42.4043021303692));
#33459=CARTESIAN_POINT('Ctrl Pts',(-39.9828760063219,41.517771422342,42.3973149724465));
#33460=CARTESIAN_POINT('Ctrl Pts',(-39.9765100781176,41.6632291297494,42.3857442791751));
#33461=CARTESIAN_POINT('Ctrl Pts',(-39.9701441499132,41.8086868371569,42.3741735859036));
#33462=CARTESIAN_POINT('Ctrl Pts',(-39.9593441519422,41.9535871586478,42.3580193797836));
#33463=CARTESIAN_POINT('Ctrl Pts',(-39.9441512967467,42.0973748198546,42.3373433776084));
#33464=CARTESIAN_POINT('Ctrl Pts',(-39.9289584415512,42.2411624810616,42.3166673754332));
#33465=CARTESIAN_POINT('Ctrl Pts',(-39.9093727587292,42.3838372001397,42.291469617535));
#33466=CARTESIAN_POINT('Ctrl Pts',(-39.8854691132612,42.5248522049747,42.2618464625567));
#33467=CARTESIAN_POINT('Ctrl Pts',(-39.8615654677932,42.6658672098096,42.2322233075785));
#33468=CARTESIAN_POINT('Ctrl Pts',(-39.8333439063365,42.805222223963,42.1981748133764));
#33469=CARTESIAN_POINT('Ctrl Pts',(-39.8009123741146,42.9423831667588,42.1598312436677));
#33470=CARTESIAN_POINT('Ctrl Pts',(-39.7684808418927,43.0795441095547,42.121487673959));
#33471=CARTESIAN_POINT('Ctrl Pts',(-39.7318394022657,43.2145107120774,42.0788491036817));
#33472=CARTESIAN_POINT('Ctrl Pts',(-39.6911282551631,43.3467656772593,42.0320787051806));
#33473=CARTESIAN_POINT('Ctrl Pts',(-39.6503809263276,43.4791381830696,41.9852667398315));
#33474=CARTESIAN_POINT('Ctrl Pts',(-39.605556732677,43.6087939697063,41.9343156903406));
#33475=CARTESIAN_POINT('Ctrl Pts',(-39.5568275136275,43.7352351624437,41.8794209091086));
#33476=CARTESIAN_POINT('Ctrl Pts',(-38.5891792041831,37.3877174389177,41.2491135147587));
#33477=CARTESIAN_POINT('Ctrl Pts',(-38.6698966078566,37.4825859979437,41.3295336941693));
#33478=CARTESIAN_POINT('Ctrl Pts',(-38.7477704437814,37.5825222780497,41.4068294727545));
#33479=CARTESIAN_POINT('Ctrl Pts',(-38.8224931492366,37.6871315856152,41.4806955534571));
#33480=CARTESIAN_POINT('Ctrl Pts',(-38.8972158546918,37.7917408931808,41.5545616341598));
#33481=CARTESIAN_POINT('Ctrl Pts',(-38.968787274099,37.9010230104245,41.6249978631657));
#33482=CARTESIAN_POINT('Ctrl Pts',(-39.0369247236146,38.0145463475696,41.6917260218454));
#33483=CARTESIAN_POINT('Ctrl Pts',(-39.1050621731301,38.1280696847148,41.7584541805251));
#33484=CARTESIAN_POINT('Ctrl Pts',(-39.1697655108715,38.2458340054359,41.8214741299099));
#33485=CARTESIAN_POINT('Ctrl Pts',(-39.2307791639605,38.3673742313302,41.8805369267837));
#33486=CARTESIAN_POINT('Ctrl Pts',(-39.2917928170496,38.4889144572246,41.9395997236574));
#33487=CARTESIAN_POINT('Ctrl Pts',(-39.3491166584187,38.6142303352866,41.9947052449932));
#33488=CARTESIAN_POINT('Ctrl Pts',(-39.4025242443065,38.7428269703345,42.0456357889521));
#33489=CARTESIAN_POINT('Ctrl Pts',(-39.4559318301942,38.8714236053824,42.0965663329109));
#33490=CARTESIAN_POINT('Ctrl Pts',(-39.5054230493503,39.003300729726,42.1433217933784));
#33491=CARTESIAN_POINT('Ctrl Pts',(-39.5508023754224,39.137937538607,42.1857174293239));
#33492=CARTESIAN_POINT('Ctrl Pts',(-39.5961817014946,39.272574347488,42.2281130652695));
#33493=CARTESIAN_POINT('Ctrl Pts',(-39.6374490399275,39.4099705606428,42.2661487883285));
#33494=CARTESIAN_POINT('Ctrl Pts',(-39.6744413261037,39.5495835754794,42.2996742776115));
#33495=CARTESIAN_POINT('Ctrl Pts',(-39.71143361228,39.689196590316,42.3331997668946));
#33496=CARTESIAN_POINT('Ctrl Pts',(-39.7441507690855,39.8310261162079,42.3622149524842));
#33497=CARTESIAN_POINT('Ctrl Pts',(-39.7724634818109,39.9745120365822,42.3866051213487));
#33498=CARTESIAN_POINT('Ctrl Pts',(-39.8007761945363,40.1179979569567,42.4109952902132));
#33499=CARTESIAN_POINT('Ctrl Pts',(-39.8246844041175,40.263139973116,42.4307603914344));
#33500=CARTESIAN_POINT('Ctrl Pts',(-39.8440935676073,40.4093648766837,42.4458222265642));
#33501=CARTESIAN_POINT('Ctrl Pts',(-39.8635027310971,40.5555897802513,42.4608840616941));
#33502=CARTESIAN_POINT('Ctrl Pts',(-39.8784128079477,40.7028972668148,42.4712425992159));
#33503=CARTESIAN_POINT('Ctrl Pts',(-39.888764774443,40.8507055618155,42.4768567738399));
#33504=CARTESIAN_POINT('Ctrl Pts',(-39.8991167409382,40.9985138568162,42.4824709484638));
#33505=CARTESIAN_POINT('Ctrl Pts',(-39.904910575367,41.1468226525277,42.4833407483241));
#33506=CARTESIAN_POINT('Ctrl Pts',(-39.9061232404223,41.2950462015824,42.4794625668233));
#33507=CARTESIAN_POINT('Ctrl Pts',(-39.9073359054777,41.443269750637,42.4755843853227));
#33508=CARTESIAN_POINT('Ctrl Pts',(-39.9039673984572,41.5914077444216,42.4669582303403));
#33509=CARTESIAN_POINT('Ctrl Pts',(-39.8960308516571,41.7388750876526,42.4536179838878));
#33510=CARTESIAN_POINT('Ctrl Pts',(-39.888094304857,41.8863424308836,42.4402777374353));
#33511=CARTESIAN_POINT('Ctrl Pts',(-39.8755897346058,42.0331388164954,42.4222234270757));
#33512=CARTESIAN_POINT('Ctrl Pts',(-39.8585663405558,42.1786844212221,42.3995261574783));
#33513=CARTESIAN_POINT('Ctrl Pts',(-39.8415429465059,42.3242300259488,42.3768288878809));
#33514=CARTESIAN_POINT('Ctrl Pts',(-39.8200007638886,42.4685245466947,42.349488706076));
#33515=CARTESIAN_POINT('Ctrl Pts',(-39.79402467282,42.6109980107428,42.3176133796576));
#33516=CARTESIAN_POINT('Ctrl Pts',(-39.7680485817515,42.7534714747909,42.2857380532391));
#33517=CARTESIAN_POINT('Ctrl Pts',(-39.7376386360887,42.8941235854065,42.2493276483347));
#33518=CARTESIAN_POINT('Ctrl Pts',(-39.7029147279111,43.0323987214329,42.2085257463487));
#33519=CARTESIAN_POINT('Ctrl Pts',(-39.6681908197334,43.1706738574592,42.1677238443626));
#33520=CARTESIAN_POINT('Ctrl Pts',(-39.6291530211,43.3065717308636,42.1225305299992));
#33521=CARTESIAN_POINT('Ctrl Pts',(-39.5859552912035,43.4395554600322,42.0731240666598));
#33522=CARTESIAN_POINT('Ctrl Pts',(-39.5427191696421,43.572657377513,42.0236736936891));
#33523=CARTESIAN_POINT('Ctrl Pts',(-39.4953158091684,43.7028396910567,41.9700027824006));
#33524=CARTESIAN_POINT('Ctrl Pts',(-39.4439325208564,43.8295871275298,41.9123234371075));
#33525=CARTESIAN_POINT('Ctrl Pts',(-38.5105944106268,37.3903900363275,41.3249697149968));
#33526=CARTESIAN_POINT('Ctrl Pts',(-38.5925880147889,37.4866716395425,41.4065204448413));
#33527=CARTESIAN_POINT('Ctrl Pts',(-38.6716518465919,37.588174582779,41.4848520562084));
#33528=CARTESIAN_POINT('Ctrl Pts',(-38.747464047146,37.6944856603538,41.559645670985));
#33529=CARTESIAN_POINT('Ctrl Pts',(-38.8232762477,37.8007967379286,41.6344392857616));
#33530=CARTESIAN_POINT('Ctrl Pts',(-38.8958366491455,37.911915714453,41.7056947383436));
#33531=CARTESIAN_POINT('Ctrl Pts',(-38.9648498672373,38.0273902385848,41.7731219567681));
#33532=CARTESIAN_POINT('Ctrl Pts',(-39.0338630853291,38.1428647627166,41.8405491751926));
#33533=CARTESIAN_POINT('Ctrl Pts',(-39.0993289672618,38.2626945787777,41.9041480101658));
#33534=CARTESIAN_POINT('Ctrl Pts',(-39.1609810096845,38.3863918746968,41.9636595588496));
#33535=CARTESIAN_POINT('Ctrl Pts',(-39.2226330521072,38.5100891706157,42.0231711075335));
#33536=CARTESIAN_POINT('Ctrl Pts',(-39.2804711185133,38.6376536725081,42.0785952381606));
#33537=CARTESIAN_POINT('Ctrl Pts',(-39.334259757427,38.7685660813717,42.1297063260836));
#33538=CARTESIAN_POINT('Ctrl Pts',(-39.3880483963409,38.8994784902351,42.1808174140066));
#33539=CARTESIAN_POINT('Ctrl Pts',(-39.4377874886664,39.0337385162099,42.2276153460581));
#33540=CARTESIAN_POINT('Ctrl Pts',(-39.4832745528305,39.1707996036594,42.2699096137572));
#33541=CARTESIAN_POINT('Ctrl Pts',(-39.5287616169945,39.307860691109,42.3122038814564));
#33542=CARTESIAN_POINT('Ctrl Pts',(-39.569996552282,39.4477225365593,42.3499943911576));
#33543=CARTESIAN_POINT('Ctrl Pts',(-39.6068114964706,39.5898157800732,42.3831273024607));
#33544=CARTESIAN_POINT('Ctrl Pts',(-39.6436264406592,39.731909023587,42.4162602137638));
#33545=CARTESIAN_POINT('Ctrl Pts',(-39.6760213122352,39.8762333505486,42.4447354533078));
#33546=CARTESIAN_POINT('Ctrl Pts',(-39.7038642357611,40.0222012348209,42.4684371019829));
#33547=CARTESIAN_POINT('Ctrl Pts',(-39.731707159287,40.1681691190932,42.4921387506579));
#33548=CARTESIAN_POINT('Ctrl Pts',(-39.7549980731144,40.3157802374815,42.511066755985));
#33549=CARTESIAN_POINT('Ctrl Pts',(-39.7736421628699,40.4644336837353,42.5251440644412));
#33550=CARTESIAN_POINT('Ctrl Pts',(-39.7922862526254,40.6130871299891,42.5392213728974));
#33551=CARTESIAN_POINT('Ctrl Pts',(-39.8062834770282,40.7627825749675,42.5484479533134));
#33552=CARTESIAN_POINT('Ctrl Pts',(-39.8155768551427,40.9129106273891,42.5527862454437));
#33553=CARTESIAN_POINT('Ctrl Pts',(-39.8248702332572,41.0630386798108,42.557124537574));
#33554=CARTESIAN_POINT('Ctrl Pts',(-39.8294597445064,41.2135990072699,42.556574531813));
#33555=CARTESIAN_POINT('Ctrl Pts',(-39.8293267055689,41.3639786976575,42.5511384671649));
#33556=CARTESIAN_POINT('Ctrl Pts',(-39.8291936666312,41.5143583880452,42.5457024025167));
#33557=CARTESIAN_POINT('Ctrl Pts',(-39.8243380778014,41.6645571083984,42.5353802910175));
#33558=CARTESIAN_POINT('Ctrl Pts',(-39.8147797055691,41.8139634186653,42.5202141526818));
#33559=CARTESIAN_POINT('Ctrl Pts',(-39.8052213333368,41.9633697289321,42.5050480143461));
#33560=CARTESIAN_POINT('Ctrl Pts',(-39.7909601988658,42.1119832983048,42.4850378827539));
#33561=CARTESIAN_POINT('Ctrl Pts',(-39.7720543574363,42.2591991396813,42.4602652166278));
#33562=CARTESIAN_POINT('Ctrl Pts',(-39.7531485160068,42.4064149810577,42.4354925505018));
#33563=CARTESIAN_POINT('Ctrl Pts',(-39.7295980094791,42.5522327684799,42.4059574046923));
#33564=CARTESIAN_POINT('Ctrl Pts',(-39.7014987089959,42.6960588961218,42.3717800130538));
#33565=CARTESIAN_POINT('Ctrl Pts',(-39.6733994085126,42.8398850237637,42.3376026214152));
#33566=CARTESIAN_POINT('Ctrl Pts',(-39.6407513762898,42.9817191731726,42.2987830596216));
#33567=CARTESIAN_POINT('Ctrl Pts',(-39.6036875183501,43.1209839554103,42.2554793572141));
#33568=CARTESIAN_POINT('Ctrl Pts',(-39.5666236604103,43.2602487376481,42.2121756548065));
#33569=CARTESIAN_POINT('Ctrl Pts',(-39.5251440588185,43.3969438443617,42.1643879076659));
#33570=CARTESIAN_POINT('Ctrl Pts',(-39.4794175718025,43.5305128070077,42.1123106536853));
#33571=CARTESIAN_POINT('Ctrl Pts',(-39.4336504457071,43.6642004780878,42.0601871164279));
#33572=CARTESIAN_POINT('Ctrl Pts',(-39.383628983482,43.7947561496885,42.0037665599188));
#33573=CARTESIAN_POINT('Ctrl Pts',(-39.3295571628989,43.921647389681,41.9432790580052));
#33574=CARTESIAN_POINT('Ctrl Pts',(-38.3401070380879,37.396188156926,41.4895374854793));
#33575=CARTESIAN_POINT('Ctrl Pts',(-38.4248693212561,37.4955353174855,41.5735409108681));
#33576=CARTESIAN_POINT('Ctrl Pts',(-38.506514813727,37.6004370897919,41.65411973065));
#33577=CARTESIAN_POINT('Ctrl Pts',(-38.5846906414969,37.7104401067918,41.7309256030157));
#33578=CARTESIAN_POINT('Ctrl Pts',(-38.6628664692668,37.8204431237917,41.8077314753812));
#33579=CARTESIAN_POINT('Ctrl Pts',(-38.7375724378322,37.9355471118982,41.880764209148));
#33580=CARTESIAN_POINT('Ctrl Pts',(-38.8084856098052,38.0552546781698,41.9497080168992));
#33581=CARTESIAN_POINT('Ctrl Pts',(-38.8793987817783,38.1749622444414,42.0186518246504));
#33582=CARTESIAN_POINT('Ctrl Pts',(-38.9465189806562,38.2992730912161,42.0835065346916));
#33583=CARTESIAN_POINT('Ctrl Pts',(-39.0095559897528,38.427650086403,42.1439916370817));
#33584=CARTESIAN_POINT('Ctrl Pts',(-39.0725929988496,38.5560270815899,42.2044767394719));
#33585=CARTESIAN_POINT('Ctrl Pts',(-39.1315466611802,38.6884699060094,42.260592083481));
#33586=CARTESIAN_POINT('Ctrl Pts',(-39.1861619833017,38.8244063172954,42.3120948561651));
#33587=CARTESIAN_POINT('Ctrl Pts',(-39.2407773054231,38.9603427285815,42.3635976288492));
#33588=CARTESIAN_POINT('Ctrl Pts',(-39.2910541512182,39.099772388779,42.4104877017388));
#33589=CARTESIAN_POINT('Ctrl Pts',(-39.3367749499686,39.2420928764857,42.4525620540421));
#33590=CARTESIAN_POINT('Ctrl Pts',(-39.3824957487191,39.3844133641924,42.4946364063455));
#33591=CARTESIAN_POINT('Ctrl Pts',(-39.423660386346,39.5296243255813,42.5318949329592));
#33592=CARTESIAN_POINT('Ctrl Pts',(-39.4600905923665,39.6770983514491,42.5641761580101));
#33593=CARTESIAN_POINT('Ctrl Pts',(-39.496520798387,39.824572377317,42.5964573830611));
#33594=CARTESIAN_POINT('Ctrl Pts',(-39.5282164817421,39.974309101005,42.6237612257167));
#33595=CARTESIAN_POINT('Ctrl Pts',(-39.555040211571,40.1256615321412,42.645969150317));
#33596=CARTESIAN_POINT('Ctrl Pts',(-39.5818639414,40.2770139632773,42.6681770749175));
#33597=CARTESIAN_POINT('Ctrl Pts',(-39.6038156504478,40.4299817255212,42.6852890255972));
#33598=CARTESIAN_POINT('Ctrl Pts',(-39.6207999354897,40.5839038229087,42.6972304327144));
#33599=CARTESIAN_POINT('Ctrl Pts',(-39.6377842205318,40.7378259202961,42.7091718398316));
#33600=CARTESIAN_POINT('Ctrl Pts',(-39.6498010386968,40.8927019700386,42.7159426729704));
#33601=CARTESIAN_POINT('Ctrl Pts',(-39.6567978408013,41.0478626671964,42.717512975975));
#33602=CARTESIAN_POINT('Ctrl Pts',(-39.6637946429058,41.2030233643541,42.7190832789797));
#33603=CARTESIAN_POINT('Ctrl Pts',(-39.6657714108332,41.3584683229798,42.715453047148));
#33604=CARTESIAN_POINT('Ctrl Pts',(-39.6627189071036,41.5135256978668,42.7066372013421));
#33605=CARTESIAN_POINT('Ctrl Pts',(-39.659666403374,41.6685830727536,42.6978213555362));
#33606=CARTESIAN_POINT('Ctrl Pts',(-39.6515846347838,41.8232524781121,42.683819916811));
#33607=CARTESIAN_POINT('Ctrl Pts',(-39.6385077605088,41.9768653196993,42.6646925603359));
#33608=CARTESIAN_POINT('Ctrl Pts',(-39.6254308862338,42.1304781612864,42.6455652038608));
#33609=CARTESIAN_POINT('Ctrl Pts',(-39.6073589379277,42.2830340567859,42.6213119762699));
#33610=CARTESIAN_POINT('Ctrl Pts',(-39.5843691828914,42.4338734269017,42.5920367990964));
#33611=CARTESIAN_POINT('Ctrl Pts',(-39.5613794278551,42.5847127970175,42.562761621923));
#33612=CARTESIAN_POINT('Ctrl Pts',(-39.5334719223308,42.7338352661928,42.5284645669829));
#33613=CARTESIAN_POINT('Ctrl Pts',(-39.5007663821658,42.8805959572736,42.489292913312));
#33614=CARTESIAN_POINT('Ctrl Pts',(-39.4680608420009,43.0273566483544,42.4501212596411));
#33615=CARTESIAN_POINT('Ctrl Pts',(-39.4305573475459,43.1717551957721,42.4060751036235));
#33616=CARTESIAN_POINT('Ctrl Pts',(-39.3884170381864,43.3131669860338,42.3573438196041));
#33617=CARTESIAN_POINT('Ctrl Pts',(-39.346276728827,43.4545787762955,42.3086125355848));
#33618=CARTESIAN_POINT('Ctrl Pts',(-39.2994997083353,43.593003456964,42.2551962436915));
#33619=CARTESIAN_POINT('Ctrl Pts',(-39.2482871579526,43.7278420662347,42.1973247888432));
#33620=CARTESIAN_POINT('Ctrl Pts',(-39.197029092792,43.8628005123285,42.1394019011646));
#33621=CARTESIAN_POINT('Ctrl Pts',(-39.1413277366783,43.9941661731301,42.0770160711227));
#33622=CARTESIAN_POINT('Ctrl Pts',(-39.0814232252891,44.1213693905809,42.0104363569345));
#33623=CARTESIAN_POINT('Ctrl Pts',(-38.1698933472347,37.4023057767316,41.654374420382));
#33624=CARTESIAN_POINT('Ctrl Pts',(-38.2574371396393,37.5046775074782,41.740752380849));
#33625=CARTESIAN_POINT('Ctrl Pts',(-38.3416705748698,37.6129487843841,41.8234930542166));
#33626=CARTESIAN_POINT('Ctrl Pts',(-38.422207032264,37.7266226511676,41.9022165301249));
#33627=CARTESIAN_POINT('Ctrl Pts',(-38.5027434896582,37.8402965179512,41.9809400060332));
#33628=CARTESIAN_POINT('Ctrl Pts',(-38.5795827433154,37.959372655871,42.0556460634807));
#33629=CARTESIAN_POINT('Ctrl Pts',(-38.6523720426952,38.0833045948027,42.1259915980532));
#33630=CARTESIAN_POINT('Ctrl Pts',(-38.725161342075,38.2072365337344,42.1963371326256));
#33631=CARTESIAN_POINT('Ctrl Pts',(-38.7939004829064,38.3360239262585,42.2623219467166));
#33632=CARTESIAN_POINT('Ctrl Pts',(-38.8582738129496,38.4690757875448,42.3236428832583));
#33633=CARTESIAN_POINT('Ctrl Pts',(-38.9226471429928,38.602127648831,42.3849638198));
#33634=CARTESIAN_POINT('Ctrl Pts',(-38.9826544814682,38.7394436059457,42.441620706383));
#33635=CARTESIAN_POINT('Ctrl Pts',(-39.0380201640102,38.8803935651702,42.4933531100336));
#33636=CARTESIAN_POINT('Ctrl Pts',(-39.0933858465522,39.0213435243946,42.5450855136842));
#33637=CARTESIAN_POINT('Ctrl Pts',(-39.1441097175204,39.165927090677,42.5918932887627));
#33638=CARTESIAN_POINT('Ctrl Pts',(-39.1899586250542,39.3134808246791,42.6335611131595));
#33639=CARTESIAN_POINT('Ctrl Pts',(-39.235807532588,39.4610345586814,42.6752289375563));
#33640=CARTESIAN_POINT('Ctrl Pts',(-39.2767813476062,39.6115580468308,42.7117566937311));
#33641=CARTESIAN_POINT('Ctrl Pts',(-39.3126915674182,39.7643605724095,42.7429761454479));
#33642=CARTESIAN_POINT('Ctrl Pts',(-39.3486017872303,39.9171630979881,42.7741955971648));
#33643=CARTESIAN_POINT('Ctrl Pts',(-39.3794483104926,40.0722442326687,42.8001066560573));
#33644=CARTESIAN_POINT('Ctrl Pts',(-39.4050890128859,40.2288923003061,42.8205897169714));
#33645=CARTESIAN_POINT('Ctrl Pts',(-39.4307297152792,40.3855403679434,42.8410727778855));
#33646=CARTESIAN_POINT('Ctrl Pts',(-39.4511645241242,40.543754929356,42.8561277824382));
#33647=CARTESIAN_POINT('Ctrl Pts',(-39.4662989994119,40.7028098591025,42.8656848578283));
#33648=CARTESIAN_POINT('Ctrl Pts',(-39.4814334746995,40.8618647888489,42.8752419332184));
#33649=CARTESIAN_POINT('Ctrl Pts',(-39.491267573081,41.0217596408937,42.8793010515829));
#33650=CARTESIAN_POINT('Ctrl Pts',(-39.4957554095817,41.1817604835205,42.8778427197039));
#33651=CARTESIAN_POINT('Ctrl Pts',(-39.5002432460823,41.3417613261473,42.8763843878249));
#33652=CARTESIAN_POINT('Ctrl Pts',(-39.4993848070836,41.5018677105294,42.869408608619));
#33653=CARTESIAN_POINT('Ctrl Pts',(-39.493183190154,41.6613446140811,42.8569464556646));
#33654=CARTESIAN_POINT('Ctrl Pts',(-39.4869815732246,41.8208215176326,42.8444843027102));
#33655=CARTESIAN_POINT('Ctrl Pts',(-39.4754367946057,41.9796684928248,42.8265358096833));
#33656=CARTESIAN_POINT('Ctrl Pts',(-39.4586009147309,42.1371561528159,42.803182342358));
#33657=CARTESIAN_POINT('Ctrl Pts',(-39.4417650348561,42.2946438128069,42.7798288750327));
#33658=CARTESIAN_POINT('Ctrl Pts',(-39.419638099685,42.4507717154438,42.7510704975448));
#33659=CARTESIAN_POINT('Ctrl Pts',(-39.3923206657399,42.6048227861614,42.7170381338524));
#33660=CARTESIAN_POINT('Ctrl Pts',(-39.3650032317948,42.7588738568789,42.68300577016));
#33661=CARTESIAN_POINT('Ctrl Pts',(-39.3324953743416,42.9108476629302,42.6436995142815));
#33662=CARTESIAN_POINT('Ctrl Pts',(-39.2949452362731,43.0600460076279,42.599298661516));
#33663=CARTESIAN_POINT('Ctrl Pts',(-39.2573950982045,43.2092443523257,42.5548978087504));
#33664=CARTESIAN_POINT('Ctrl Pts',(-39.2148027834144,43.3556668162752,42.50540248215));
#33665=CARTESIAN_POINT('Ctrl Pts',(-39.1673626766853,43.4986404754819,42.4510387193772));
#33666=CARTESIAN_POINT('Ctrl Pts',(-39.1199225699561,43.6416141346887,42.3966749566045));
#33667=CARTESIAN_POINT('Ctrl Pts',(-39.0676348028709,43.7811385869357,42.3374429086328));
#33668=CARTESIAN_POINT('Ctrl Pts',(-39.010738234995,43.9165723466299,42.2736132990986));
#33669=CARTESIAN_POINT('Ctrl Pts',(-38.9537911007125,44.052126472083,42.2097269614679));
#33670=CARTESIAN_POINT('Ctrl Pts',(-38.892227128286,44.1835822485594,42.1412350643881));
#33671=CARTESIAN_POINT('Ctrl Pts',(-38.8263282286146,44.3103338969357,42.0684513874025));
#33672=CARTESIAN_POINT('Ctrl Pts',(-38.0000876683942,37.4088997145424,41.8196126328366));
#33673=CARTESIAN_POINT('Ctrl Pts',(-38.0904681512693,37.5142776343105,41.9082850918914));
#33674=CARTESIAN_POINT('Ctrl Pts',(-38.1773371111399,37.6259135682359,41.9930992333451));
#33675=CARTESIAN_POINT('Ctrl Pts',(-38.2602708604475,37.7432630321777,42.0736413913554));
#33676=CARTESIAN_POINT('Ctrl Pts',(-38.3432046097552,37.8606124961195,42.1541835493656));
#33677=CARTESIAN_POINT('Ctrl Pts',(-38.4222028848055,37.9836751169552,42.2304534678416));
#33678=CARTESIAN_POINT('Ctrl Pts',(-38.4968803858612,38.111850678957,42.3020791538276));
#33679=CARTESIAN_POINT('Ctrl Pts',(-38.5715578869169,38.2400262409588,42.3737048398136));
#33680=CARTESIAN_POINT('Ctrl Pts',(-38.6419143765348,38.3733143365819,42.4406860655693));
#33681=CARTESIAN_POINT('Ctrl Pts',(-38.7076067036954,38.5110648771956,42.5026961420409));
#33682=CARTESIAN_POINT('Ctrl Pts',(-38.7732990308561,38.6488154178094,42.5647062185125));
#33683=CARTESIAN_POINT('Ctrl Pts',(-38.8343269866852,38.7910279654247,42.6217449485334));
#33684=CARTESIAN_POINT('Ctrl Pts',(-38.8903929183668,38.937008903999,42.6735341357586));
#33685=CARTESIAN_POINT('Ctrl Pts',(-38.9464588500485,39.0829898425733,42.7253233229839));
#33686=CARTESIAN_POINT('Ctrl Pts',(-38.9975625793161,39.2327387079484,42.7718628027449));
#33687=CARTESIAN_POINT('Ctrl Pts',(-39.0434548569381,39.3855251270308,42.8129255868781));
#33688=CARTESIAN_POINT('Ctrl Pts',(-39.0893471345601,39.5383115461131,42.8539883710113));
#33689=CARTESIAN_POINT('Ctrl Pts',(-39.1300278146177,39.6941350331057,42.8895743289534));
#33690=CARTESIAN_POINT('Ctrl Pts',(-39.1652984843805,39.852235587009,42.9195098963547));
#33691=CARTESIAN_POINT('Ctrl Pts',(-39.2005691541434,40.0103361409123,42.9494454637562));
#33692=CARTESIAN_POINT('Ctrl Pts',(-39.2304297014648,40.1707132590325,42.9737305454333));
#33693=CARTESIAN_POINT('Ctrl Pts',(-39.2547344868207,40.3325847308073,42.9922466950162));
#33694=CARTESIAN_POINT('Ctrl Pts',(-39.2790392721765,40.494456202582,43.0107628445991));
#33695=CARTESIAN_POINT('Ctrl Pts',(-39.2977882182871,40.6578215133272,43.0235100032131));
#33696=CARTESIAN_POINT('Ctrl Pts',(-39.310889880424,40.821883878049,43.0304259986301));
#33697=CARTESIAN_POINT('Ctrl Pts',(-39.3239915425609,40.9859462427706,43.0373419940472));
#33698=CARTESIAN_POINT('Ctrl Pts',(-39.3314458790656,41.1507051398183,43.0384268042762));
#33699=CARTESIAN_POINT('Ctrl Pts',(-39.333216532603,41.31535698716,43.0336751381041));
#33700=CARTESIAN_POINT('Ctrl Pts',(-39.3349871861405,41.4800088345017,43.0289234719321));
#33701=CARTESIAN_POINT('Ctrl Pts',(-39.3310741510799,41.6445531086124,43.0183353444663));
#33702=CARTESIAN_POINT('Ctrl Pts',(-39.3214965123727,41.8081872741634,43.0019623971693));
#33703=CARTESIAN_POINT('Ctrl Pts',(-39.3119188736654,41.9718214397145,42.9855894498722));
#33704=CARTESIAN_POINT('Ctrl Pts',(-39.2966766617635,42.1345449764166,42.963431734802));
#33705=CARTESIAN_POINT('Ctrl Pts',(-39.2758442176283,42.2955642291726,42.9355973220397));
#33706=CARTESIAN_POINT('Ctrl Pts',(-39.2550117734931,42.4565834819286,42.9077629092774));
#33707=CARTESIAN_POINT('Ctrl Pts',(-39.2285891633622,42.6158979387632,42.8742518873238));
#33708=CARTESIAN_POINT('Ctrl Pts',(-39.19670525858,42.7727305716617,42.8352277000236));
#33709=CARTESIAN_POINT('Ctrl Pts',(-39.1648213537978,42.9295632045603,42.7962035127234));
#33710=CARTESIAN_POINT('Ctrl Pts',(-39.1274762557409,43.083913514859,42.7516662841563));
#33711=CARTESIAN_POINT('Ctrl Pts',(-39.084852108241,43.2350286861848,42.7018332365743));
#33712=CARTESIAN_POINT('Ctrl Pts',(-39.042227960741,43.3861438575105,42.6520001889924));
#33713=CARTESIAN_POINT('Ctrl Pts',(-38.9943248993241,43.5340234093782,42.596871480843));
#33714=CARTESIAN_POINT('Ctrl Pts',(-38.9413765624222,43.6779460852896,42.5367159924989));
#33715=CARTESIAN_POINT('Ctrl Pts',(-38.8884282255205,43.821868761201,42.4765605041547));
#33716=CARTESIAN_POINT('Ctrl Pts',(-38.8304347814866,43.9618341035397,42.4113784268845));
#33717=CARTESIAN_POINT('Ctrl Pts',(-38.7676790828296,44.097159455865,42.3414876746605));
#33718=CARTESIAN_POINT('Ctrl Pts',(-38.7048676105065,44.2326050776027,42.2715348075442));
#33719=CARTESIAN_POINT('Ctrl Pts',(-38.6372856148521,44.3634020271021,42.1968651147725));
#33720=CARTESIAN_POINT('Ctrl Pts',(-38.5652632803349,44.4889112104465,42.1178434117343));
#33721=CARTESIAN_POINT('Ctrl Pts',(-38.0398886763558,37.4073630839945,41.7808966890927));
#33722=CARTESIAN_POINT('Ctrl Pts',(-38.196487830305,37.401351958814,41.6286232707617));
#33723=CARTESIAN_POINT('Ctrl Pts',(-38.353424823516,37.395735231147,41.4766821154713));
#33724=CARTESIAN_POINT('Ctrl Pts',(-38.5105944106295,37.3903900363274,41.3249697149942));
#33725=CARTESIAN_POINT('Ctrl Pts',(-38.5891792041849,37.3877174389176,41.249113514757));
#33726=CARTESIAN_POINT('Ctrl Pts',(-38.6678226442078,37.3851133060814,41.1733149929954));
#33727=CARTESIAN_POINT('Ctrl Pts',(-38.7465138697966,37.3825649586746,41.0975634680728));
#33728=CARTESIAN_POINT('Ctrl Pts',(-38.825205095388,37.3800166112678,41.0218119431476));
#33729=CARTESIAN_POINT('Ctrl Pts',(-38.9039441351633,37.3775240826995,40.946107443207));
#33730=CARTESIAN_POINT('Ctrl Pts',(-38.9827210478919,37.3750757674608,40.8704401911061));
#33731=CARTESIAN_POINT('Ctrl Pts',(-39.0614979606169,37.3726274522222,40.7947729390086));
#33732=CARTESIAN_POINT('Ctrl Pts',(-39.1403127743051,37.3702233830122,40.7191429622981));
#33733=CARTESIAN_POINT('Ctrl Pts',(-39.2191560456546,37.3678525356093,40.6435409735397));
#33734=CARTESIAN_POINT('Ctrl Pts',(-39.2979993170057,37.3654816882064,40.5679389847796));
#33735=CARTESIAN_POINT('Ctrl Pts',(-39.3768710769017,37.3631440986645,40.4923650143452));
#33736=CARTESIAN_POINT('Ctrl Pts',(-39.4557619421374,37.3608288129201,40.4168098339066));
#33737=CARTESIAN_POINT('Ctrl Pts',(-39.5346528073732,37.3585135271757,40.341254653468));
#33738=CARTESIAN_POINT('Ctrl Pts',(-39.6135628167506,37.3562205905267,40.2657183011866));
#33739=CARTESIAN_POINT('Ctrl Pts',(-39.6924821306133,37.3539385160429,40.1901910998149));
#33740=CARTESIAN_POINT('Ctrl Pts',(-39.7714014444796,37.3516564415591,40.1146638984399));
#33741=CARTESIAN_POINT('Ctrl Pts',(-39.8503301182025,37.3493852938815,40.0391459024319));
#33742=CARTESIAN_POINT('Ctrl Pts',(-39.9292571604855,37.3471122416419,39.9636263019119));
#33743=CARTESIAN_POINT('Ctrl Pts',(-40.0081842027615,37.3448391894025,39.8881067013986));
#33744=CARTESIAN_POINT('Ctrl Pts',(-40.087109702463,37.3425643363435,39.8125855837718));
#33745=CARTESIAN_POINT('Ctrl Pts',(-40.166020457705,37.3402722704297,39.7370499650508));
#33746=CARTESIAN_POINT('Ctrl Pts',(-40.2449312129548,37.3379802045157,39.6615143463223));
#33747=CARTESIAN_POINT('Ctrl Pts',(-40.3238273833577,37.3356711120805,39.5859643834778));
#33748=CARTESIAN_POINT('Ctrl Pts',(-40.4026917455433,37.3333248863596,39.5103831374279));
#33749=CARTESIAN_POINT('Ctrl Pts',(-40.4421239266295,37.3321517734993,39.4725925144092));
#33750=CARTESIAN_POINT('Ctrl Pts',(-40.4815480803642,37.3309692894147,39.4347939965346));
#33751=CARTESIAN_POINT('Ctrl Pts',(-40.520961424251,37.329774185787,39.3969848472346));
#33752=CARTESIAN_POINT('Ctrl Pts',(-40.5603747681469,37.328579082159,39.3591756979259));
#33753=CARTESIAN_POINT('Ctrl Pts',(-40.5997773169133,37.3273713761704,39.3213559316673));
#33754=CARTESIAN_POINT('Ctrl Pts',(-40.6391656485399,37.3261470729261,39.2835221829305));
#33755=CARTESIAN_POINT('Ctrl Pts',(-40.678553980157,37.3249227696822,39.2456884342028));
#33756=CARTESIAN_POINT('Ctrl Pts',(-40.7179281175588,37.3236818959449,39.2078407255431));
#33757=CARTESIAN_POINT('Ctrl Pts',(-40.7572837211927,37.3224193856699,39.1699747890254));
#33758=CARTESIAN_POINT('Ctrl Pts',(-40.7966393248366,37.3211568753946,39.1321088524983));
#33759=CARTESIAN_POINT('Ctrl Pts',(-40.8359764322357,37.3198727723864,39.0942247250169));
#33760=CARTESIAN_POINT('Ctrl Pts',(-40.8752893413857,37.3185604200586,39.0563167986917));
#33761=CARTESIAN_POINT('Ctrl Pts',(-40.9146022505253,37.3172480677311,39.0184088723765));
#33762=CARTESIAN_POINT('Ctrl Pts',(-40.9538910266967,37.3159075422936,38.9804772114209));
#33763=CARTESIAN_POINT('Ctrl Pts',(-40.9931478523898,37.3145297174934,38.942514127347));
#33764=CARTESIAN_POINT('Ctrl Pts',(-41.0324046780937,37.3131518926928,38.9045510432627));
#33765=CARTESIAN_POINT('Ctrl Pts',(-41.0716296760241,37.3117369117765,38.8665566567397));
#33766=CARTESIAN_POINT('Ctrl Pts',(-41.110811545496,37.3102715821923,38.8285198536169));
#33767=CARTESIAN_POINT('Ctrl Pts',(-41.1304024802235,37.3095389174004,38.8095014520637));
#33768=CARTESIAN_POINT('Ctrl Pts',(-41.1499825689311,37.3087935908378,38.7904723835099));
#33769=CARTESIAN_POINT('Ctrl Pts',(-41.1695498758672,37.3080333426855,38.7714307441549));
#33770=CARTESIAN_POINT('Ctrl Pts',(-41.1891171828148,37.3072730945327,38.7523891047887));
#33771=CARTESIAN_POINT('Ctrl Pts',(-41.208671719699,37.3064979384582,38.733334906136));
#33772=CARTESIAN_POINT('Ctrl Pts',(-41.2282110281082,37.3057050044836,38.7142657303626));
#33773=CARTESIAN_POINT('Ctrl Pts',(-41.2477503365059,37.3049120705096,38.6951965546006));
#33774=CARTESIAN_POINT('Ctrl Pts',(-41.2672744347923,37.3041013800735,38.6761124197787));
#33775=CARTESIAN_POINT('Ctrl Pts',(-41.2867801198516,37.3032691938202,38.6570101756499));
#33776=CARTESIAN_POINT('Ctrl Pts',(-41.3062858049228,37.3024370075665,38.6379079315096));
#33777=CARTESIAN_POINT('Ctrl Pts',(-41.3257731069796,37.3015833607664,38.6187876077765));
#33778=CARTESIAN_POINT('Ctrl Pts',(-41.3452377207335,37.3007032273755,38.5996449702233));
#33779=CARTESIAN_POINT('Ctrl Pts',(-41.3647023344753,37.2998230939851,38.580502332682));
#33780=CARTESIAN_POINT('Ctrl Pts',(-41.3841443126135,37.298916535526,38.5613374331501));
#33781=CARTESIAN_POINT('Ctrl Pts',(-41.4035576403255,37.2979765302234,38.5421443560828));
#33782=CARTESIAN_POINT('Ctrl Pts',(-41.4229709680498,37.2970365249202,38.5229512790035));
#33783=CARTESIAN_POINT('Ctrl Pts',(-41.4423557441877,37.2960631881607,38.5037301215973));
#33784=CARTESIAN_POINT('Ctrl Pts',(-41.4617031412364,37.2950462146141,38.484472202064));
#33785=CARTESIAN_POINT('Ctrl Pts',(-41.4810505382725,37.2940292410683,38.4652142825432));
#33786=CARTESIAN_POINT('Ctrl Pts',(-41.5003607592692,37.2929688677782,38.4459198005936));
#33787=CARTESIAN_POINT('Ctrl Pts',(-41.5196199854035,37.2918489624883,38.4265751654797));
#33788=CARTESIAN_POINT('Ctrl Pts',(-41.5292495984738,37.2912890098432,38.4169028479197));
#33789=CARTESIAN_POINT('Ctrl Pts',(-41.5388663699674,37.2907140657909,38.4072179007401));
#33790=CARTESIAN_POINT('Ctrl Pts',(-41.5484677647746,37.2901211708148,38.3975178306749));
#33791=CARTESIAN_POINT('Ctrl Pts',(-41.5580691595883,37.2895282758384,38.3878177606031));
#33792=CARTESIAN_POINT('Ctrl Pts',(-41.5676552001071,37.2889174560781,38.3781025896675));
#33793=CARTESIAN_POINT('Ctrl Pts',(-41.5772224902082,37.2882847468604,38.3683689778));
#33794=CARTESIAN_POINT('Ctrl Pts',(-41.5867897802965,37.2876520376437,38.3586353659456));
#33795=CARTESIAN_POINT('Ctrl Pts',(-41.5963383565882,37.2869974817215,38.3488833491761));
#33796=CARTESIAN_POINT('Ctrl Pts',(-41.6058635266892,37.286315601138,38.3391083125477));
#33797=CARTESIAN_POINT('Ctrl Pts',(-41.6153886968031,37.2856337205536,38.3293332759061));
#33798=CARTESIAN_POINT('Ctrl Pts',(-41.6248905220874,37.2849245869414,38.3195352797541));
#33799=CARTESIAN_POINT('Ctrl Pts',(-41.6343622916865,37.2841803659703,38.3097077240023));
#33800=CARTESIAN_POINT('Ctrl Pts',(-41.6438340612728,37.2834361450001,38.299880168264));
#33801=CARTESIAN_POINT('Ctrl Pts',(-41.6532758769268,37.2826569554584,38.2900231529994));
#33802=CARTESIAN_POINT('Ctrl Pts',(-41.6626778025202,37.2818311977926,38.2801269060814));
#33803=CARTESIAN_POINT('Ctrl Pts',(-41.6720797281266,37.2810054401256,38.2702306591499));
#33804=CARTESIAN_POINT('Ctrl Pts',(-41.6814419126922,37.280133288302,38.2602953271252));
#33805=CARTESIAN_POINT('Ctrl Pts',(-41.6907493023114,37.2791971682157,38.2503061045745));
#33806=CARTESIAN_POINT('Ctrl Pts',(-41.6954029971114,37.2787291081736,38.2453114933095));
#33807=CARTESIAN_POINT('Ctrl Pts',(-41.7000428977186,37.2782449446291,38.2403033155323));
#33808=CARTESIAN_POINT('Ctrl Pts',(-41.7046664632498,37.2777417113255,38.2352790722985));
#33809=CARTESIAN_POINT('Ctrl Pts',(-41.7092900287873,37.2772384780212,38.2302548290579));
#33810=CARTESIAN_POINT('Ctrl Pts',(-41.7138972585809,37.276716174178,38.2252145197037));
#33811=CARTESIAN_POINT('Ctrl Pts',(-41.7184851250849,37.2761712654037,38.2201551666616));
#33812=CARTESIAN_POINT('Ctrl Pts',(-41.7230729915889,37.2756263566294,38.2150958136196));
#33813=CARTESIAN_POINT('Ctrl Pts',(-41.7276414848393,37.2750588312918,38.21001740709));
#33814=CARTESIAN_POINT('Ctrl Pts',(-41.7321871653729,37.2744646741212,38.20491656438));
#33815=CARTESIAN_POINT('Ctrl Pts',(-41.7367328459131,37.2738705169498,38.1998157216626));
#33816=CARTESIAN_POINT('Ctrl Pts',(-41.7412556909106,37.2732497012984,38.1946924203157));
#33817=CARTESIAN_POINT('Ctrl Pts',(-41.7457520939533,37.2725980169989,38.1895431134528));
#33818=CARTESIAN_POINT('Ctrl Pts',(-41.7502484969831,37.2719463327013,38.1843938066046));
#33819=CARTESIAN_POINT('Ctrl Pts',(-41.7547184267385,37.271263743193,38.1792184634379));
#33820=CARTESIAN_POINT('Ctrl Pts',(-41.7591585257862,37.2705463289669,38.1740137819355));
#33821=CARTESIAN_POINT('Ctrl Pts',(-41.7635986248468,37.2698289147387,38.1688091004181));
#33822=CARTESIAN_POINT('Ctrl Pts',(-41.7680088677799,37.2690766461175,38.163575055565));
#33823=CARTESIAN_POINT('Ctrl Pts',(-41.7723865878687,37.2682864099468,38.1583090246749));
#33824=CARTESIAN_POINT('Ctrl Pts',(-41.7767643079513,37.2674961737772,38.1530429937924));
#33825=CARTESIAN_POINT('Ctrl Pts',(-41.7811094995483,37.2666679632042,38.1477449708898));
#33826=CARTESIAN_POINT('Ctrl Pts',(-41.7854204349472,37.2657997620299,38.1424132579943));
#33827=CARTESIAN_POINT('Ctrl Pts',(-41.7864981687969,37.2655827117364,38.1410803297704));
#33828=CARTESIAN_POINT('Ctrl Pts',(-41.7875737620729,37.2653631624537,38.1397452962095));
#33829=CARTESIAN_POINT('Ctrl Pts',(-41.7886472050151,37.2651411028499,38.1384081478136));
#33830=CARTESIAN_POINT('Ctrl Pts',(-41.7889155657455,37.2650855879501,38.1380738607211));
#33831=CARTESIAN_POINT('Ctrl Pts',(-41.7891882242383,37.2650307276919,38.1377366532483));
#33832=CARTESIAN_POINT('Ctrl Pts',(-41.789451172242,37.2649739597976,38.137405330718));
#33833=CARTESIAN_POINT('Ctrl Pts',(-41.7897141202531,37.2649171919017,38.1370740081785));
#33834=CARTESIAN_POINT('Ctrl Pts',(-41.7899770299188,37.2648604923531,38.1367426435067));
#33835=CARTESIAN_POINT('Ctrl Pts',(-41.7902399729327,37.2648037333654,38.1364113154772));
#33836=CARTESIAN_POINT('Ctrl Pts',(-41.7907658589594,37.2646902153904,38.1357486594197));
#33837=CARTESIAN_POINT('Ctrl Pts',(-41.7912917036929,37.2645767709905,38.1350859579939));
#33838=CARTESIAN_POINT('Ctrl Pts',(-41.7918175742758,37.2644632804643,38.1344232849708));
#33839=CARTESIAN_POINT('Ctrl Pts',(-41.7939210565952,37.2640093183625,38.1317725928941));
#33840=CARTESIAN_POINT('Ctrl Pts',(-41.7960245110482,37.2635554059264,38.1291218701979));
#33841=CARTESIAN_POINT('Ctrl Pts',(-41.7981279794346,37.2631014686576,38.1264711628116));
#33842=CARTESIAN_POINT('Origin',(-36.3078527277528,58.7571818148754,39.9768461872608));
#33843=CARTESIAN_POINT('',(-33.5529552244032,70.2939023154161,29.521482977958));
#33844=CARTESIAN_POINT('',(-26.1333050833765,70.2640602812185,36.2258025733947));
#33845=CARTESIAN_POINT('Origin',(-29.8431301538898,70.2789812983173,32.8736427756763));
#33846=CARTESIAN_POINT('',(-40.0176777982662,58.7721028319742,36.6246863895425));
#33847=CARTESIAN_POINT('',(-40.0176777982662,58.7721028319742,36.6246863895425));
#33848=CARTESIAN_POINT('',(-32.5980276572394,58.7422607977766,43.3290059849791));
#33849=CARTESIAN_POINT('Origin',(-36.3078527277528,58.7571818148754,39.9768461872608));
#33850=CARTESIAN_POINT('',(-32.5980276572394,58.7422607977766,43.3290059849791));
#33851=CARTESIAN_POINT('Origin',(-32.5980276572394,58.7422607977766,43.3290059849791));
#33852=CARTESIAN_POINT('',(-24.4181484426939,68.1256242727979,34.3181253946216));
#33853=CARTESIAN_POINT('',(-26.1333050833765,70.2640602812185,36.2258025733947));
#33854=CARTESIAN_POINT('',(-30.8828710165569,56.603824789356,41.4213288062061));
#33855=CARTESIAN_POINT('',(-32.5980276572394,58.7422607977766,43.3290059849791));
#33856=CARTESIAN_POINT('',(-30.8828710165569,56.603824789356,41.4213288062061));
#33857=CARTESIAN_POINT('Origin',(-30.14514456676,51.0735937808341,33.1223948565145));
#33858=CARTESIAN_POINT('',(-23.7241967287056,67.8609953274847,34.5204571570535));
#33859=CARTESIAN_POINT('Origin',(-23.680421992897,62.595393264276,26.01919144493));
#33860=CARTESIAN_POINT('',(-30.1889193025686,56.3391958440429,41.623660568638));
#33861=CARTESIAN_POINT('Origin',(-30.14514456676,51.0735937808341,33.1223948565145));
#33862=CARTESIAN_POINT('',(-30.1889193025686,56.3391958440429,41.623660568638));
#33863=CARTESIAN_POINT('Origin',(-5.81522832743221,46.4801655823699,45.702859600428));
#33864=CARTESIAN_POINT('Origin',(-17.0047025368452,45.7553165663936,36.4551430811504));
#33865=CARTESIAN_POINT('',(-19.0137036843474,67.8420495966423,38.7768102493421));
#33866=CARTESIAN_POINT('',(-10.5399799629823,57.2771160498355,29.3519396695659));
#33867=CARTESIAN_POINT('',(-10.5399799629823,57.2771160498355,29.3519396695659));
#33868=CARTESIAN_POINT('',(-25.4784262582104,56.3202501132004,45.8800136609266));
#33869=CARTESIAN_POINT('',(-25.4784262582104,56.3202501132004,45.8800136609266));
#33870=CARTESIAN_POINT('',(-17.0047025368452,45.7553165663936,36.4551430811504));
#33871=CARTESIAN_POINT('',(-17.0047025368452,45.7553165663936,36.4551430811504));
#33872=CARTESIAN_POINT('',(-17.0047025368452,45.7553165663936,36.4551430811504));
#33873=CARTESIAN_POINT('Origin',(-25.4784262582104,56.3202501132004,45.8800136609266));
#33874=CARTESIAN_POINT('',(-19.0137036843474,67.8420495966423,38.7768102493421));
#33875=CARTESIAN_POINT('',(-25.4784262582104,56.3202501132004,45.8800136609266));
#33876=CARTESIAN_POINT('Origin',(-17.0047025368452,45.7553165663936,36.4551430811504));
#33877=CARTESIAN_POINT('',(-10.5399799629823,57.2771160498355,29.3519396695659));
#33878=CARTESIAN_POINT('',(-17.0047025368452,45.7553165663936,36.4551430811504));
#33879=CARTESIAN_POINT('Origin',(-37.9028116553955,37.2474344007039,41.6462389504159));
#33880=CARTESIAN_POINT('Origin',(-40.0176777982662,58.7721028319742,36.6246863895425));
#33881=CARTESIAN_POINT('',(-33.5529552244032,70.2939023154161,29.521482977958));
#33882=CARTESIAN_POINT('',(-40.0176777982662,58.7721028319742,36.6246863895425));
#33883=CARTESIAN_POINT('Origin',(-29.8431301538898,70.2789812983173,32.8736427756763));
#33884=CARTESIAN_POINT('Origin',(-44.6514843000067,41.123844669555,31.2333209653637));
#33885=CARTESIAN_POINT('Origin',(-18.0776624288824,72.5809528165923,19.8630818215568));
#33886=CARTESIAN_POINT('Origin',(-36.3078527277528,58.7571818148754,39.9768461872608));
#33887=CARTESIAN_POINT('Origin',(-53.2977525215594,44.2689648703008,19.9340598087839));
#33888=CARTESIAN_POINT('Origin',(-7.08622728734316,53.9840227357375,43.4139320205864));
#33889=CARTESIAN_POINT('',(-13.7639124142673,54.0108805665153,37.3800443846934));
#33890=CARTESIAN_POINT('',(-14.8937422437826,55.4195383727563,38.6366937953302));
#33891=CARTESIAN_POINT('',(-13.7639124142673,54.0108805665153,37.3800443846934));
#33892=CARTESIAN_POINT('',(-8.21605711685851,55.3926805419784,44.6705814312232));
#33893=CARTESIAN_POINT('',(-8.21605711685851,55.3926805419784,44.6705814312232));
#33894=CARTESIAN_POINT('',(-7.08622728734316,53.9840227357375,43.4139320205864));
#33895=CARTESIAN_POINT('',(-7.08622728734316,53.9840227357375,43.4139320205864));
#33896=CARTESIAN_POINT('',(-7.08622728734316,53.9840227357375,43.4139320205864));
#33897=CARTESIAN_POINT('Origin',(-7.34481619029768,53.5231507563998,43.6980601570498));
#33898=CARTESIAN_POINT('',(-14.0225013172218,53.5500085871777,37.6641725211568));
#33899=CARTESIAN_POINT('',(-14.0225013172218,53.5500085871777,37.6641725211568));
#33900=CARTESIAN_POINT('',(-7.34481619029768,53.5231507563998,43.6980601570498));
#33901=CARTESIAN_POINT('',(-7.34481619029768,53.5231507563998,43.6980601570498));
#33902=CARTESIAN_POINT('',(-7.34481619029768,53.5231507563998,43.6980601570498));
#33903=CARTESIAN_POINT('Origin',(-12.5509467813568,62.5506302129796,36.075670838085));
#33904=CARTESIAN_POINT('',(-15.1523311467371,54.9586663934186,38.9208219317936));
#33905=CARTESIAN_POINT('',(-15.1523311467371,54.9586663934186,38.9208219317936));
#33906=CARTESIAN_POINT('',(-14.8937422437826,55.4195383727563,38.6366937953302));
#33907=CARTESIAN_POINT('Origin',(-16.2626702143646,66.7932946931195,17.8286736257813));
#33908=CARTESIAN_POINT('Origin',(-8.21605711685851,55.3926805419784,44.6705814312232));
#33909=CARTESIAN_POINT('',(-8.47464601981303,54.9318085626407,44.9547095676866));
#33910=CARTESIAN_POINT('',(-8.47464601981303,54.9318085626407,44.9547095676866));
#33911=CARTESIAN_POINT('',(-8.21605711685851,55.3926805419784,44.6705814312232));
#33912=CARTESIAN_POINT('Origin',(-5.87326165443273,62.5237723822018,42.109558473978));
#33913=CARTESIAN_POINT('',(-8.47464601981303,54.9318085626407,44.9547095676866));
#33914=CARTESIAN_POINT('Origin',(-8.47464601981303,54.9318085626407,44.9547095676866));
#33915=CARTESIAN_POINT('Origin',(-9.55849548170321,62.9036549880343,48.8745226900051));
#62948=UNCERTAINTY_MEASURE_WITH_UNIT(LENGTH_MEASURE(0.01),#62975,
'DISTANCE_ACCURACY_VALUE',
'Maximum model space distance between geometric entities at asserted c
onnectivities');
#62960=UNCERTAINTY_MEASURE_WITH_UNIT(LENGTH_MEASURE(0.01),#62975,
'DISTANCE_ACCURACY_VALUE',
'Maximum model space distance between geometric entities at asserted c
onnectivities');
#62962=(
GEOMETRIC_REPRESENTATION_CONTEXT(3)
GLOBAL_UNCERTAINTY_ASSIGNED_CONTEXT((#62948))
GLOBAL_UNIT_ASSIGNED_CONTEXT((#62975,#62977,#62978))
REPRESENTATION_CONTEXT('','3D')
);
#62974=(
GEOMETRIC_REPRESENTATION_CONTEXT(3)
GLOBAL_UNCERTAINTY_ASSIGNED_CONTEXT((#62960))
GLOBAL_UNIT_ASSIGNED_CONTEXT((#62975,#62977,#62978))
REPRESENTATION_CONTEXT('','3D')
);
#62975=(
LENGTH_UNIT()
NAMED_UNIT(*)
SI_UNIT(.MILLI.,.METRE.)
);
#62977=(
NAMED_UNIT(*)
PLANE_ANGLE_UNIT()
SI_UNIT($,.RADIAN.)
);
#62978=(
NAMED_UNIT(*)
SI_UNIT($,.STERADIAN.)
SOLID_ANGLE_UNIT()
);
#62980=SHAPE_DEFINITION_REPRESENTATION(#62993,#63021);
#62993=PRODUCT_DEFINITION_SHAPE('',$,#63035);
#63021=SHAPE_REPRESENTATION('',(#15338),#62962);
#63033=PRODUCT_DEFINITION_CONTEXT('part definition',#63074,'design');
#63035=PRODUCT_DEFINITION('Fuel Injector & Bracket',
'Fuel Injector & Bracket',#63048,#63033);
#63048=PRODUCT_DEFINITION_FORMATION('',$,#63077);
#63074=APPLICATION_CONTEXT(
'Core Data for Automotive Mechanical Design Process');
#63075=PRODUCT_CONTEXT('part definition',#63074,'mechanical');
#63077=PRODUCT('Fuel Injector & Bracket','Fuel Injector & Bracket',$,(#63075));
#63090=PRESENTATION_STYLE_ASSIGNMENT((#63092));
#63092=SURFACE_STYLE_USAGE(.BOTH.,#63094);
#63094=SURFACE_SIDE_STYLE('',(#63096));
#63096=SURFACE_STYLE_FILL_AREA(#63098);
#63098=FILL_AREA_STYLE('Opaque(202,209,238)',(#63100));
#63100=FILL_AREA_STYLE_COLOUR('Opaque(202,209,238)',#63102);
#63102=COLOUR_RGB('Opaque(202,209,238)', 0.66274510, 0.83137255, 0.94901961);
ENDSEC;
END-ISO-10303-21;
